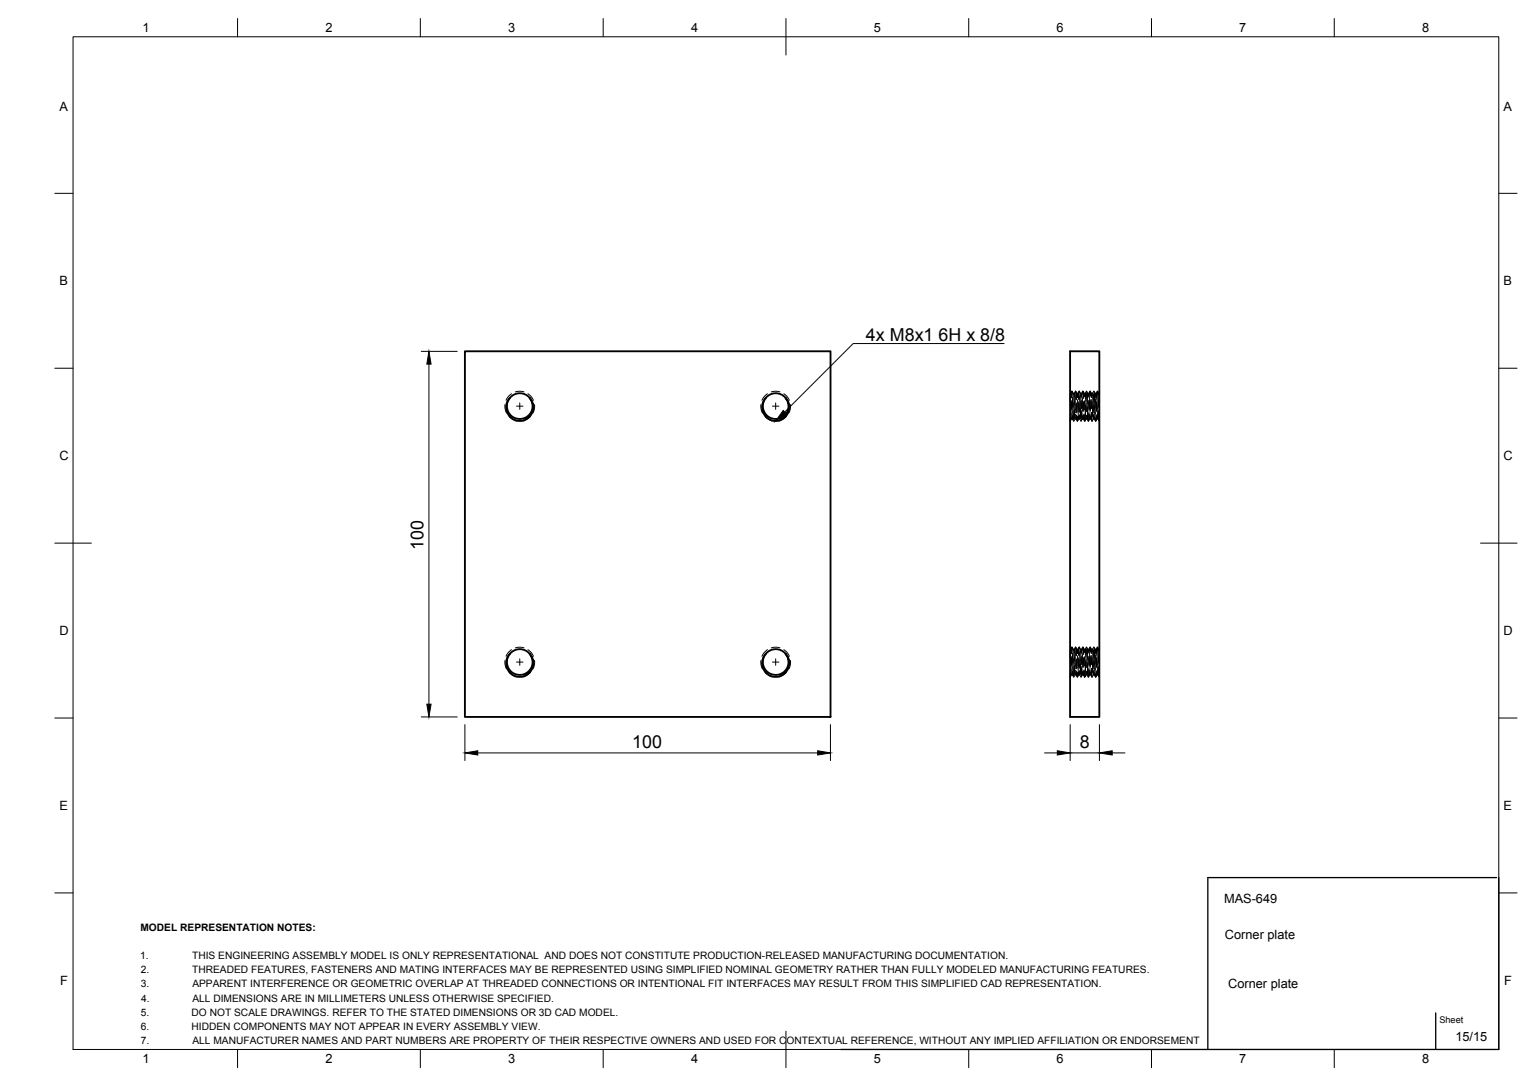
ISO-10303-21;
HEADER;
/* Generated by software containing ST-Developer
 * from STEP Tools, Inc. (www.steptools.com) 
 */

FILE_DESCRIPTION(
/* description */ ('Independent equipment support assembly with bolted 600 x 500 mm welde
d perimeter frame, four adjustable legs and swivel feet. Nominal overa
ll height 518 mm. No load rating assigned.'),
/* implementation_level */ '2;1');

FILE_NAME(
/* name */ 'Corner plate.step',
/* time_stamp */ '2026-11-07T17:30:39-08:00',
/* author */ (''),
/* organization */ (''),
/* preprocessor_version */ 'ST-DEVELOPER v20.2',
/* originating_system */ 'Autodesk Translation Framework v15.17.0.0',
/* authorisation */ '');

FILE_SCHEMA (('AUTOMOTIVE_DESIGN { 1 0 10303 214 3 1 1 }'));
ENDSEC;

DATA;
#10=MECHANICAL_DESIGN_GEOMETRIC_PRESENTATION_REPRESENTATION('',(#2210),#63755);
#257=B_SPLINE_SURFACE_WITH_KNOTS('',3,3,((#20700,#20701,#20702,#20703,#20704,
#20705,#20706,#20707,#20708,#20709,#20710,#20711,#20712,#20713,#20714,#20715,
#20716,#20717,#20718,#20719,#20720,#20721,#20722,#20723,#20724,#20725,#20726,
#20727,#20728,#20729,#20730,#20731,#20732,#20733,#20734,#20735,#20736,#20737,
#20738,#20739,#20740,#20741,#20742,#20743,#20744,#20745,#20746,#20747,#20748,
#20749,#20750,#20751,#20752,#20753,#20754,#20755),(#20756,#20757,#20758,
#20759,#20760,#20761,#20762,#20763,#20764,#20765,#20766,#20767,#20768,#20769,
#20770,#20771,#20772,#20773,#20774,#20775,#20776,#20777,#20778,#20779,#20780,
#20781,#20782,#20783,#20784,#20785,#20786,#20787,#20788,#20789,#20790,#20791,
#20792,#20793,#20794,#20795,#20796,#20797,#20798,#20799,#20800,#20801,#20802,
#20803,#20804,#20805,#20806,#20807,#20808,#20809,#20810,#20811),(#20812,
#20813,#20814,#20815,#20816,#20817,#20818,#20819,#20820,#20821,#20822,#20823,
#20824,#20825,#20826,#20827,#20828,#20829,#20830,#20831,#20832,#20833,#20834,
#20835,#20836,#20837,#20838,#20839,#20840,#20841,#20842,#20843,#20844,#20845,
#20846,#20847,#20848,#20849,#20850,#20851,#20852,#20853,#20854,#20855,#20856,
#20857,#20858,#20859,#20860,#20861,#20862,#20863,#20864,#20865,#20866,#20867),
(#20868,#20869,#20870,#20871,#20872,#20873,#20874,#20875,#20876,#20877,
#20878,#20879,#20880,#20881,#20882,#20883,#20884,#20885,#20886,#20887,#20888,
#20889,#20890,#20891,#20892,#20893,#20894,#20895,#20896,#20897,#20898,#20899,
#20900,#20901,#20902,#20903,#20904,#20905,#20906,#20907,#20908,#20909,#20910,
#20911,#20912,#20913,#20914,#20915,#20916,#20917,#20918,#20919,#20920,#20921,
#20922,#20923)),.UNSPECIFIED.,.F.,.F.,.F.,(4,4),(4,1,1,1,1,1,1,1,1,1,1,
1,1,1,1,1,1,1,1,1,1,1,1,1,1,1,1,1,1,1,1,1,1,1,1,1,1,1,1,1,1,1,1,1,1,1,1,
1,1,1,1,1,1,4),(0.,0.0642013499338865),(11.8589888623078,12.8454497557128,
13.8319106491178,14.8183715425228,15.8048324359278,16.7912933293328,17.7777542227378,
18.7642151161428,19.7506760095478,20.7371369029528,21.7235977963578,22.7100586897628,
23.6965195831678,24.6829804765728,25.6694413699778,26.6559022633828,27.6423631567878,
28.6288240501928,29.6152849435978,30.6017458370028,31.5882067304078,32.5746676238129,
33.5611285172179,34.5475894106229,35.5340503040279,36.5205111974329,37.5069720908379,
38.4934329842429,39.4798938776479,40.4663547710529,41.4528156644579,42.4392765578629,
43.4257374512679,44.4121983446729,45.3986592380779,46.3851201314829,47.3715810248879,
48.3580419182929,49.3445028116979,50.3309637051029,51.3174245985079,52.3038854919129,
53.2903463853179,54.2768072787229,55.2632681721279,56.2497290655329,57.2361899589379,
58.2226508523429,59.2091117457479,60.1955726391529,61.1820335325579,62.1684944259629,
63.1549553193679,64.1414162127729),.UNSPECIFIED.);
#258=B_SPLINE_SURFACE_WITH_KNOTS('',3,3,((#21140,#21141,#21142,#21143,#21144,
#21145,#21146,#21147,#21148,#21149,#21150,#21151,#21152,#21153,#21154,#21155,
#21156,#21157,#21158,#21159,#21160,#21161,#21162,#21163,#21164,#21165,#21166,
#21167,#21168,#21169,#21170,#21171,#21172,#21173,#21174,#21175,#21176,#21177,
#21178,#21179,#21180,#21181,#21182,#21183,#21184,#21185,#21186,#21187,#21188,
#21189,#21190,#21191,#21192,#21193,#21194,#21195),(#21196,#21197,#21198,
#21199,#21200,#21201,#21202,#21203,#21204,#21205,#21206,#21207,#21208,#21209,
#21210,#21211,#21212,#21213,#21214,#21215,#21216,#21217,#21218,#21219,#21220,
#21221,#21222,#21223,#21224,#21225,#21226,#21227,#21228,#21229,#21230,#21231,
#21232,#21233,#21234,#21235,#21236,#21237,#21238,#21239,#21240,#21241,#21242,
#21243,#21244,#21245,#21246,#21247,#21248,#21249,#21250,#21251),(#21252,
#21253,#21254,#21255,#21256,#21257,#21258,#21259,#21260,#21261,#21262,#21263,
#21264,#21265,#21266,#21267,#21268,#21269,#21270,#21271,#21272,#21273,#21274,
#21275,#21276,#21277,#21278,#21279,#21280,#21281,#21282,#21283,#21284,#21285,
#21286,#21287,#21288,#21289,#21290,#21291,#21292,#21293,#21294,#21295,#21296,
#21297,#21298,#21299,#21300,#21301,#21302,#21303,#21304,#21305,#21306,#21307),
(#21308,#21309,#21310,#21311,#21312,#21313,#21314,#21315,#21316,#21317,
#21318,#21319,#21320,#21321,#21322,#21323,#21324,#21325,#21326,#21327,#21328,
#21329,#21330,#21331,#21332,#21333,#21334,#21335,#21336,#21337,#21338,#21339,
#21340,#21341,#21342,#21343,#21344,#21345,#21346,#21347,#21348,#21349,#21350,
#21351,#21352,#21353,#21354,#21355,#21356,#21357,#21358,#21359,#21360,#21361,
#21362,#21363)),.UNSPECIFIED.,.F.,.F.,.F.,(4,4),(4,1,1,1,1,1,1,1,1,1,1,
1,1,1,1,1,1,1,1,1,1,1,1,1,1,1,1,1,1,1,1,1,1,1,1,1,1,1,1,1,1,1,1,1,1,1,1,
1,1,1,1,1,1,4),(0.,0.0642013499338865),(14.3984001269718,15.3848610203768,
16.3713219137818,17.3577828071868,18.3442437005918,19.3307045939968,20.3171654874019,
21.3036263808069,22.2900872742119,23.2765481676169,24.2630090610219,25.2494699544269,
26.2359308478319,27.2223917412369,28.2088526346419,29.1953135280469,30.1817744214519,
31.1682353148569,32.1546962082619,33.1411571016669,34.1276179950719,35.1140788884769,
36.1005397818819,37.0870006752869,38.0734615686919,39.0599224620969,40.0463833555019,
41.0328442489069,42.0193051423119,43.0057660357169,43.9922269291219,44.9786878225269,
45.9651487159319,46.9516096093369,47.9380705027419,48.9245313961469,49.9109922895519,
50.8974531829569,51.8839140763619,52.8703749697669,53.856835863172,54.843296756577,
55.829757649982,56.816218543387,57.802679436792,58.789140330197,59.775601223602,
60.762062117007,61.748523010412,62.734983903817,63.721444797222,64.707905690627,
65.694366584032,66.680827477437),.UNSPECIFIED.);
#259=B_SPLINE_SURFACE_WITH_KNOTS('',3,3,((#22184,#22185,#22186,#22187,#22188,
#22189,#22190,#22191,#22192,#22193,#22194,#22195,#22196,#22197,#22198,#22199,
#22200,#22201,#22202,#22203,#22204,#22205,#22206,#22207,#22208,#22209,#22210,
#22211,#22212,#22213,#22214,#22215,#22216,#22217,#22218,#22219,#22220,#22221,
#22222,#22223,#22224,#22225,#22226,#22227,#22228,#22229,#22230,#22231,#22232,
#22233,#22234,#22235,#22236,#22237,#22238,#22239),(#22240,#22241,#22242,
#22243,#22244,#22245,#22246,#22247,#22248,#22249,#22250,#22251,#22252,#22253,
#22254,#22255,#22256,#22257,#22258,#22259,#22260,#22261,#22262,#22263,#22264,
#22265,#22266,#22267,#22268,#22269,#22270,#22271,#22272,#22273,#22274,#22275,
#22276,#22277,#22278,#22279,#22280,#22281,#22282,#22283,#22284,#22285,#22286,
#22287,#22288,#22289,#22290,#22291,#22292,#22293,#22294,#22295),(#22296,
#22297,#22298,#22299,#22300,#22301,#22302,#22303,#22304,#22305,#22306,#22307,
#22308,#22309,#22310,#22311,#22312,#22313,#22314,#22315,#22316,#22317,#22318,
#22319,#22320,#22321,#22322,#22323,#22324,#22325,#22326,#22327,#22328,#22329,
#22330,#22331,#22332,#22333,#22334,#22335,#22336,#22337,#22338,#22339,#22340,
#22341,#22342,#22343,#22344,#22345,#22346,#22347,#22348,#22349,#22350,#22351),
(#22352,#22353,#22354,#22355,#22356,#22357,#22358,#22359,#22360,#22361,
#22362,#22363,#22364,#22365,#22366,#22367,#22368,#22369,#22370,#22371,#22372,
#22373,#22374,#22375,#22376,#22377,#22378,#22379,#22380,#22381,#22382,#22383,
#22384,#22385,#22386,#22387,#22388,#22389,#22390,#22391,#22392,#22393,#22394,
#22395,#22396,#22397,#22398,#22399,#22400,#22401,#22402,#22403,#22404,#22405,
#22406,#22407)),.UNSPECIFIED.,.F.,.F.,.F.,(4,4),(4,1,1,1,1,1,1,1,1,1,1,
1,1,1,1,1,1,1,1,1,1,1,1,1,1,1,1,1,1,1,1,1,1,1,1,1,1,1,1,1,1,1,1,1,1,1,1,
1,1,1,1,1,1,4),(0.,0.0642013499338865),(11.8589888623078,12.8454497557128,
13.8319106491178,14.8183715425228,15.8048324359278,16.7912933293328,17.7777542227378,
18.7642151161428,19.7506760095478,20.7371369029528,21.7235977963578,22.7100586897628,
23.6965195831678,24.6829804765728,25.6694413699778,26.6559022633828,27.6423631567879,
28.6288240501929,29.6152849435979,30.6017458370029,31.5882067304079,32.5746676238129,
33.5611285172179,34.5475894106229,35.5340503040279,36.5205111974329,37.5069720908379,
38.4934329842429,39.4798938776479,40.4663547710529,41.4528156644579,42.4392765578629,
43.4257374512679,44.4121983446729,45.3986592380779,46.3851201314829,47.3715810248879,
48.3580419182929,49.3445028116979,50.3309637051029,51.3174245985079,52.3038854919129,
53.2903463853179,54.2768072787229,55.2632681721279,56.2497290655329,57.2361899589379,
58.2226508523429,59.2091117457479,60.1955726391529,61.1820335325579,62.1684944259629,
63.154955319368,64.141416212773),.UNSPECIFIED.);
#260=B_SPLINE_SURFACE_WITH_KNOTS('',3,3,((#22530,#22531,#22532,#22533,#22534,
#22535,#22536,#22537,#22538,#22539,#22540,#22541,#22542,#22543,#22544,#22545,
#22546,#22547,#22548,#22549,#22550,#22551,#22552,#22553,#22554,#22555,#22556,
#22557,#22558,#22559,#22560,#22561,#22562,#22563,#22564,#22565,#22566,#22567,
#22568,#22569,#22570,#22571,#22572,#22573,#22574,#22575,#22576,#22577,#22578,
#22579,#22580,#22581,#22582,#22583,#22584,#22585),(#22586,#22587,#22588,
#22589,#22590,#22591,#22592,#22593,#22594,#22595,#22596,#22597,#22598,#22599,
#22600,#22601,#22602,#22603,#22604,#22605,#22606,#22607,#22608,#22609,#22610,
#22611,#22612,#22613,#22614,#22615,#22616,#22617,#22618,#22619,#22620,#22621,
#22622,#22623,#22624,#22625,#22626,#22627,#22628,#22629,#22630,#22631,#22632,
#22633,#22634,#22635,#22636,#22637,#22638,#22639,#22640,#22641),(#22642,
#22643,#22644,#22645,#22646,#22647,#22648,#22649,#22650,#22651,#22652,#22653,
#22654,#22655,#22656,#22657,#22658,#22659,#22660,#22661,#22662,#22663,#22664,
#22665,#22666,#22667,#22668,#22669,#22670,#22671,#22672,#22673,#22674,#22675,
#22676,#22677,#22678,#22679,#22680,#22681,#22682,#22683,#22684,#22685,#22686,
#22687,#22688,#22689,#22690,#22691,#22692,#22693,#22694,#22695,#22696,#22697),
(#22698,#22699,#22700,#22701,#22702,#22703,#22704,#22705,#22706,#22707,
#22708,#22709,#22710,#22711,#22712,#22713,#22714,#22715,#22716,#22717,#22718,
#22719,#22720,#22721,#22722,#22723,#22724,#22725,#22726,#22727,#22728,#22729,
#22730,#22731,#22732,#22733,#22734,#22735,#22736,#22737,#22738,#22739,#22740,
#22741,#22742,#22743,#22744,#22745,#22746,#22747,#22748,#22749,#22750,#22751,
#22752,#22753)),.UNSPECIFIED.,.F.,.F.,.F.,(4,4),(4,1,1,1,1,1,1,1,1,1,1,
1,1,1,1,1,1,1,1,1,1,1,1,1,1,1,1,1,1,1,1,1,1,1,1,1,1,1,1,1,1,1,1,1,1,1,1,
1,1,1,1,1,1,4),(0.,0.0642013499338865),(14.3984001269718,15.3848610203768,
16.3713219137818,17.3577828071869,18.3442437005919,19.3307045939969,20.3171654874019,
21.3036263808069,22.2900872742119,23.2765481676169,24.2630090610219,25.2494699544269,
26.2359308478319,27.2223917412369,28.2088526346419,29.1953135280469,30.1817744214519,
31.1682353148569,32.1546962082619,33.1411571016669,34.1276179950719,35.1140788884769,
36.1005397818819,37.0870006752869,38.0734615686919,39.0599224620969,40.0463833555019,
41.0328442489069,42.0193051423119,43.0057660357169,43.9922269291219,44.9786878225269,
45.9651487159319,46.9516096093369,47.9380705027419,48.9245313961469,49.9109922895519,
50.8974531829569,51.8839140763619,52.8703749697669,53.856835863172,54.843296756577,
55.829757649982,56.816218543387,57.802679436792,58.789140330197,59.775601223602,
60.762062117007,61.748523010412,62.734983903817,63.721444797222,64.707905690627,
65.694366584032,66.680827477437),.UNSPECIFIED.);
#261=B_SPLINE_SURFACE_WITH_KNOTS('',3,3,((#22895,#22896,#22897,#22898,#22899,
#22900,#22901,#22902,#22903,#22904,#22905,#22906,#22907,#22908,#22909,#22910,
#22911,#22912,#22913,#22914,#22915,#22916,#22917,#22918,#22919,#22920,#22921,
#22922,#22923,#22924,#22925,#22926,#22927,#22928,#22929,#22930,#22931,#22932,
#22933,#22934,#22935,#22936,#22937,#22938,#22939,#22940,#22941,#22942,#22943,
#22944,#22945,#22946,#22947,#22948,#22949,#22950),(#22951,#22952,#22953,
#22954,#22955,#22956,#22957,#22958,#22959,#22960,#22961,#22962,#22963,#22964,
#22965,#22966,#22967,#22968,#22969,#22970,#22971,#22972,#22973,#22974,#22975,
#22976,#22977,#22978,#22979,#22980,#22981,#22982,#22983,#22984,#22985,#22986,
#22987,#22988,#22989,#22990,#22991,#22992,#22993,#22994,#22995,#22996,#22997,
#22998,#22999,#23000,#23001,#23002,#23003,#23004,#23005,#23006),(#23007,
#23008,#23009,#23010,#23011,#23012,#23013,#23014,#23015,#23016,#23017,#23018,
#23019,#23020,#23021,#23022,#23023,#23024,#23025,#23026,#23027,#23028,#23029,
#23030,#23031,#23032,#23033,#23034,#23035,#23036,#23037,#23038,#23039,#23040,
#23041,#23042,#23043,#23044,#23045,#23046,#23047,#23048,#23049,#23050,#23051,
#23052,#23053,#23054,#23055,#23056,#23057,#23058,#23059,#23060,#23061,#23062),
(#23063,#23064,#23065,#23066,#23067,#23068,#23069,#23070,#23071,#23072,
#23073,#23074,#23075,#23076,#23077,#23078,#23079,#23080,#23081,#23082,#23083,
#23084,#23085,#23086,#23087,#23088,#23089,#23090,#23091,#23092,#23093,#23094,
#23095,#23096,#23097,#23098,#23099,#23100,#23101,#23102,#23103,#23104,#23105,
#23106,#23107,#23108,#23109,#23110,#23111,#23112,#23113,#23114,#23115,#23116,
#23117,#23118)),.UNSPECIFIED.,.F.,.F.,.F.,(4,4),(4,1,1,1,1,1,1,1,1,1,1,
1,1,1,1,1,1,1,1,1,1,1,1,1,1,1,1,1,1,1,1,1,1,1,1,1,1,1,1,1,1,1,1,1,1,1,1,
1,1,1,1,1,1,4),(0.,0.0642013499338865),(11.8589888623078,12.8454497557128,
13.8319106491178,14.8183715425228,15.8048324359278,16.7912933293328,17.7777542227378,
18.7642151161428,19.7506760095478,20.7371369029528,21.7235977963578,22.7100586897628,
23.6965195831678,24.6829804765728,25.6694413699778,26.6559022633828,27.6423631567878,
28.6288240501928,29.6152849435978,30.6017458370028,31.5882067304078,32.5746676238129,
33.5611285172179,34.5475894106229,35.5340503040279,36.5205111974329,37.5069720908379,
38.4934329842429,39.4798938776479,40.4663547710529,41.4528156644579,42.4392765578629,
43.4257374512679,44.4121983446729,45.3986592380779,46.3851201314829,47.3715810248879,
48.3580419182929,49.3445028116979,50.3309637051029,51.3174245985079,52.3038854919129,
53.2903463853179,54.2768072787229,55.2632681721279,56.2497290655329,57.2361899589379,
58.2226508523429,59.2091117457479,60.1955726391529,61.1820335325579,62.1684944259629,
63.1549553193679,64.1414162127729),.UNSPECIFIED.);
#262=B_SPLINE_SURFACE_WITH_KNOTS('',3,3,((#23241,#23242,#23243,#23244,#23245,
#23246,#23247,#23248,#23249,#23250,#23251,#23252,#23253,#23254,#23255,#23256,
#23257,#23258,#23259,#23260,#23261,#23262,#23263,#23264,#23265,#23266,#23267,
#23268,#23269,#23270,#23271,#23272,#23273,#23274,#23275,#23276,#23277,#23278,
#23279,#23280,#23281,#23282,#23283,#23284,#23285,#23286,#23287,#23288,#23289,
#23290,#23291,#23292,#23293,#23294,#23295,#23296),(#23297,#23298,#23299,
#23300,#23301,#23302,#23303,#23304,#23305,#23306,#23307,#23308,#23309,#23310,
#23311,#23312,#23313,#23314,#23315,#23316,#23317,#23318,#23319,#23320,#23321,
#23322,#23323,#23324,#23325,#23326,#23327,#23328,#23329,#23330,#23331,#23332,
#23333,#23334,#23335,#23336,#23337,#23338,#23339,#23340,#23341,#23342,#23343,
#23344,#23345,#23346,#23347,#23348,#23349,#23350,#23351,#23352),(#23353,
#23354,#23355,#23356,#23357,#23358,#23359,#23360,#23361,#23362,#23363,#23364,
#23365,#23366,#23367,#23368,#23369,#23370,#23371,#23372,#23373,#23374,#23375,
#23376,#23377,#23378,#23379,#23380,#23381,#23382,#23383,#23384,#23385,#23386,
#23387,#23388,#23389,#23390,#23391,#23392,#23393,#23394,#23395,#23396,#23397,
#23398,#23399,#23400,#23401,#23402,#23403,#23404,#23405,#23406,#23407,#23408),
(#23409,#23410,#23411,#23412,#23413,#23414,#23415,#23416,#23417,#23418,
#23419,#23420,#23421,#23422,#23423,#23424,#23425,#23426,#23427,#23428,#23429,
#23430,#23431,#23432,#23433,#23434,#23435,#23436,#23437,#23438,#23439,#23440,
#23441,#23442,#23443,#23444,#23445,#23446,#23447,#23448,#23449,#23450,#23451,
#23452,#23453,#23454,#23455,#23456,#23457,#23458,#23459,#23460,#23461,#23462,
#23463,#23464)),.UNSPECIFIED.,.F.,.F.,.F.,(4,4),(4,1,1,1,1,1,1,1,1,1,1,
1,1,1,1,1,1,1,1,1,1,1,1,1,1,1,1,1,1,1,1,1,1,1,1,1,1,1,1,1,1,1,1,1,1,1,1,
1,1,1,1,1,1,4),(0.,0.0642013499338865),(14.3984001269718,15.3848610203768,
16.3713219137818,17.3577828071868,18.3442437005918,19.3307045939968,20.3171654874019,
21.3036263808069,22.2900872742119,23.2765481676169,24.2630090610219,25.2494699544269,
26.2359308478319,27.2223917412369,28.2088526346419,29.1953135280469,30.1817744214519,
31.1682353148569,32.1546962082619,33.1411571016669,34.1276179950719,35.1140788884769,
36.1005397818819,37.0870006752869,38.0734615686919,39.0599224620969,40.0463833555019,
41.0328442489069,42.0193051423119,43.0057660357169,43.9922269291219,44.9786878225269,
45.9651487159319,46.9516096093369,47.9380705027419,48.9245313961469,49.9109922895519,
50.8974531829569,51.8839140763619,52.8703749697669,53.856835863172,54.843296756577,
55.829757649982,56.816218543387,57.802679436792,58.789140330197,59.775601223602,
60.762062117007,61.748523010412,62.734983903817,63.721444797222,64.707905690627,
65.694366584032,66.680827477437),.UNSPECIFIED.);
#263=B_SPLINE_SURFACE_WITH_KNOTS('',3,3,((#23606,#23607,#23608,#23609,#23610,
#23611,#23612,#23613,#23614,#23615,#23616,#23617,#23618,#23619,#23620,#23621,
#23622,#23623,#23624,#23625,#23626,#23627,#23628,#23629,#23630,#23631,#23632,
#23633,#23634,#23635,#23636,#23637,#23638,#23639,#23640,#23641,#23642,#23643,
#23644,#23645,#23646,#23647,#23648,#23649,#23650,#23651,#23652,#23653,#23654,
#23655,#23656,#23657,#23658,#23659,#23660,#23661),(#23662,#23663,#23664,
#23665,#23666,#23667,#23668,#23669,#23670,#23671,#23672,#23673,#23674,#23675,
#23676,#23677,#23678,#23679,#23680,#23681,#23682,#23683,#23684,#23685,#23686,
#23687,#23688,#23689,#23690,#23691,#23692,#23693,#23694,#23695,#23696,#23697,
#23698,#23699,#23700,#23701,#23702,#23703,#23704,#23705,#23706,#23707,#23708,
#23709,#23710,#23711,#23712,#23713,#23714,#23715,#23716,#23717),(#23718,
#23719,#23720,#23721,#23722,#23723,#23724,#23725,#23726,#23727,#23728,#23729,
#23730,#23731,#23732,#23733,#23734,#23735,#23736,#23737,#23738,#23739,#23740,
#23741,#23742,#23743,#23744,#23745,#23746,#23747,#23748,#23749,#23750,#23751,
#23752,#23753,#23754,#23755,#23756,#23757,#23758,#23759,#23760,#23761,#23762,
#23763,#23764,#23765,#23766,#23767,#23768,#23769,#23770,#23771,#23772,#23773),
(#23774,#23775,#23776,#23777,#23778,#23779,#23780,#23781,#23782,#23783,
#23784,#23785,#23786,#23787,#23788,#23789,#23790,#23791,#23792,#23793,#23794,
#23795,#23796,#23797,#23798,#23799,#23800,#23801,#23802,#23803,#23804,#23805,
#23806,#23807,#23808,#23809,#23810,#23811,#23812,#23813,#23814,#23815,#23816,
#23817,#23818,#23819,#23820,#23821,#23822,#23823,#23824,#23825,#23826,#23827,
#23828,#23829)),.UNSPECIFIED.,.F.,.F.,.F.,(4,4),(4,1,1,1,1,1,1,1,1,1,1,
1,1,1,1,1,1,1,1,1,1,1,1,1,1,1,1,1,1,1,1,1,1,1,1,1,1,1,1,1,1,1,1,1,1,1,1,
1,1,1,1,1,1,4),(0.,0.0642013499338865),(11.8589888623078,12.8454497557128,
13.8319106491178,14.8183715425228,15.8048324359278,16.7912933293328,17.7777542227378,
18.7642151161428,19.7506760095478,20.7371369029528,21.7235977963578,22.7100586897628,
23.6965195831678,24.6829804765728,25.6694413699778,26.6559022633828,27.6423631567879,
28.6288240501929,29.6152849435979,30.6017458370029,31.5882067304079,32.5746676238129,
33.5611285172179,34.5475894106229,35.5340503040279,36.5205111974329,37.5069720908379,
38.4934329842429,39.4798938776479,40.4663547710529,41.4528156644579,42.4392765578629,
43.4257374512679,44.4121983446729,45.3986592380779,46.3851201314829,47.3715810248879,
48.3580419182929,49.3445028116979,50.3309637051029,51.3174245985079,52.3038854919129,
53.2903463853179,54.2768072787229,55.2632681721279,56.2497290655329,57.2361899589379,
58.2226508523429,59.2091117457479,60.1955726391529,61.1820335325579,62.1684944259629,
63.154955319368,64.141416212773),.UNSPECIFIED.);
#264=B_SPLINE_SURFACE_WITH_KNOTS('',3,3,((#23952,#23953,#23954,#23955,#23956,
#23957,#23958,#23959,#23960,#23961,#23962,#23963,#23964,#23965,#23966,#23967,
#23968,#23969,#23970,#23971,#23972,#23973,#23974,#23975,#23976,#23977,#23978,
#23979,#23980,#23981,#23982,#23983,#23984,#23985,#23986,#23987,#23988,#23989,
#23990,#23991,#23992,#23993,#23994,#23995,#23996,#23997,#23998,#23999,#24000,
#24001,#24002,#24003,#24004,#24005,#24006,#24007),(#24008,#24009,#24010,
#24011,#24012,#24013,#24014,#24015,#24016,#24017,#24018,#24019,#24020,#24021,
#24022,#24023,#24024,#24025,#24026,#24027,#24028,#24029,#24030,#24031,#24032,
#24033,#24034,#24035,#24036,#24037,#24038,#24039,#24040,#24041,#24042,#24043,
#24044,#24045,#24046,#24047,#24048,#24049,#24050,#24051,#24052,#24053,#24054,
#24055,#24056,#24057,#24058,#24059,#24060,#24061,#24062,#24063),(#24064,
#24065,#24066,#24067,#24068,#24069,#24070,#24071,#24072,#24073,#24074,#24075,
#24076,#24077,#24078,#24079,#24080,#24081,#24082,#24083,#24084,#24085,#24086,
#24087,#24088,#24089,#24090,#24091,#24092,#24093,#24094,#24095,#24096,#24097,
#24098,#24099,#24100,#24101,#24102,#24103,#24104,#24105,#24106,#24107,#24108,
#24109,#24110,#24111,#24112,#24113,#24114,#24115,#24116,#24117,#24118,#24119),
(#24120,#24121,#24122,#24123,#24124,#24125,#24126,#24127,#24128,#24129,
#24130,#24131,#24132,#24133,#24134,#24135,#24136,#24137,#24138,#24139,#24140,
#24141,#24142,#24143,#24144,#24145,#24146,#24147,#24148,#24149,#24150,#24151,
#24152,#24153,#24154,#24155,#24156,#24157,#24158,#24159,#24160,#24161,#24162,
#24163,#24164,#24165,#24166,#24167,#24168,#24169,#24170,#24171,#24172,#24173,
#24174,#24175)),.UNSPECIFIED.,.F.,.F.,.F.,(4,4),(4,1,1,1,1,1,1,1,1,1,1,
1,1,1,1,1,1,1,1,1,1,1,1,1,1,1,1,1,1,1,1,1,1,1,1,1,1,1,1,1,1,1,1,1,1,1,1,
1,1,1,1,1,1,4),(0.,0.0642013499338865),(14.3984001269718,15.3848610203768,
16.3713219137818,17.3577828071869,18.3442437005919,19.3307045939969,20.3171654874019,
21.3036263808069,22.2900872742119,23.2765481676169,24.2630090610219,25.2494699544269,
26.2359308478319,27.2223917412369,28.2088526346419,29.1953135280469,30.1817744214519,
31.1682353148569,32.1546962082619,33.1411571016669,34.1276179950719,35.1140788884769,
36.1005397818819,37.0870006752869,38.0734615686919,39.0599224620969,40.0463833555019,
41.0328442489069,42.0193051423119,43.0057660357169,43.9922269291219,44.9786878225269,
45.9651487159319,46.9516096093369,47.9380705027419,48.9245313961469,49.9109922895519,
50.8974531829569,51.8839140763619,52.8703749697669,53.856835863172,54.843296756577,
55.829757649982,56.816218543387,57.802679436792,58.789140330197,59.775601223602,
60.762062117007,61.748523010412,62.734983903817,63.721444797222,64.707905690627,
65.694366584032,66.680827477437),.UNSPECIFIED.);
#285=CIRCLE('',#14528,3.5175);
#286=CIRCLE('',#14536,3.5175);
#287=CIRCLE('',#14538,3.5175);
#288=CIRCLE('',#14546,3.5175);
#289=CIRCLE('',#14548,3.5175);
#290=CIRCLE('',#14556,3.5175);
#291=CIRCLE('',#14558,3.5175);
#292=CIRCLE('',#14566,3.5175);
#293=CIRCLE('',#14568,4.0735);
#294=CIRCLE('',#14576,4.07350000000001);
#295=CIRCLE('',#14578,4.0735);
#296=CIRCLE('',#14586,4.07350000000001);
#297=CIRCLE('',#14588,4.0735);
#298=CIRCLE('',#14596,4.0735);
#299=CIRCLE('',#14598,4.0735);
#300=CIRCLE('',#14606,4.0735);
#487=B_SPLINE_CURVE_WITH_KNOTS('',3,(#18487,#18488,#18489,#18490),
 .UNSPECIFIED.,.F.,.F.,(4,4),(51.5750455984138,52.2824273504652),
 .UNSPECIFIED.);
#488=B_SPLINE_CURVE_WITH_KNOTS('',3,(#18493,#18494,#18495,#18496,#18497,
#18498,#18499,#18500,#18501,#18502),.UNSPECIFIED.,.F.,.F.,(4,3,3,4),(-50.2654824574367,
-49.3230446702501,-48.3365837768451,-47.8312715558983),.UNSPECIFIED.);
#489=B_SPLINE_CURVE_WITH_KNOTS('',3,(#18507,#18508,#18509,#18510,#18511,
#18512,#18513,#18514,#18515,#18516,#18517,#18518,#18519,#18520,#18521,#18522,
#18523,#18524,#18525,#18526,#18527,#18528,#18529,#18530,#18531),
 .UNSPECIFIED.,.F.,.F.,(4,3,3,3,3,3,3,3,4),(45.2918602912342,45.3772010966301,
46.3636619900351,47.3501228834401,48.3365837768452,49.3230446702501,50.3095055636552,
51.2959664570602,51.5750455984138),.UNSPECIFIED.);
#490=B_SPLINE_CURVE_WITH_KNOTS('',3,(#18532,#18533,#18534,#18535,#18536,
#18537,#18538,#18539,#18540,#18541,#18542,#18543,#18544,#18545,#18546,#18547,
#18548,#18549,#18550,#18551,#18552,#18553),.UNSPECIFIED.,.F.,.F.,(4,3,3,
3,3,3,3,4),(-47.8312715558983,-47.3501228834401,-46.3636619900351,-45.3772010966301,
-44.3907402032251,-43.4042793098201,-42.4178184164151,-41.5480862487187),
 .UNSPECIFIED.);
#491=B_SPLINE_CURVE_WITH_KNOTS('',3,(#18558,#18559,#18560,#18561,#18562,
#18563,#18564,#18565,#18566,#18567,#18568,#18569,#18570,#18571,#18572,#18573,
#18574,#18575,#18576,#18577,#18578,#18579),.UNSPECIFIED.,.F.,.F.,(4,3,3,
3,3,3,3,4),(39.0086749840546,39.4584357362001,40.4448966296051,41.4313575230101,
42.4178184164151,43.4042793098201,44.3907402032251,45.2918602912342),
 .UNSPECIFIED.);
#492=B_SPLINE_CURVE_WITH_KNOTS('',3,(#18580,#18581,#18582,#18583,#18584,
#18585,#18586,#18587,#18588,#18589,#18590,#18591,#18592,#18593,#18594,#18595,
#18596,#18597,#18598,#18599,#18600,#18601,#18602,#18603,#18604),
 .UNSPECIFIED.,.F.,.F.,(4,3,3,3,3,3,3,3,4),(-41.5480862487187,-41.4313575230101,
-40.4448966296051,-39.4584357362001,-38.4719748427951,-37.4855139493901,
-36.4990530559851,-35.5125921625801,-35.2649009415391),.UNSPECIFIED.);
#493=B_SPLINE_CURVE_WITH_KNOTS('',3,(#18609,#18610,#18611,#18612,#18613,
#18614,#18615,#18616,#18617,#18618,#18619,#18620,#18621,#18622,#18623,#18624,
#18625,#18626,#18627,#18628,#18629,#18630),.UNSPECIFIED.,.F.,.F.,(4,3,3,
3,3,3,3,4),(32.725489676875,33.5396703757701,34.5261312691751,35.5125921625801,
36.4990530559851,37.4855139493901,38.4719748427951,39.0086749840546),
 .UNSPECIFIED.);
#494=B_SPLINE_CURVE_WITH_KNOTS('',3,(#18631,#18632,#18633,#18634,#18635,
#18636,#18637,#18638,#18639,#18640,#18641,#18642,#18643,#18644,#18645,#18646,
#18647,#18648,#18649,#18650,#18651,#18652),.UNSPECIFIED.,.F.,.F.,(4,3,3,
3,3,3,3,4),(-35.2649009415391,-34.5261312691751,-33.5396703757701,-32.5532094823651,
-31.5667485889601,-30.5802876955551,-29.5938268021501,-28.9817156343595),
 .UNSPECIFIED.);
#495=B_SPLINE_CURVE_WITH_KNOTS('',3,(#18657,#18658,#18659,#18660,#18661,
#18662,#18663,#18664,#18665,#18666,#18667,#18668,#18669,#18670,#18671,#18672,
#18673,#18674,#18675,#18676,#18677,#18678,#18679,#18680,#18681),
 .UNSPECIFIED.,.F.,.F.,(4,3,3,3,3,3,3,3,4),(26.4423043696954,26.6344441219351,
27.6209050153401,28.6073659087451,29.5938268021501,30.5802876955551,31.5667485889601,
32.5532094823651,32.725489676875),.UNSPECIFIED.);
#496=B_SPLINE_CURVE_WITH_KNOTS('',3,(#18682,#18683,#18684,#18685,#18686,
#18687,#18688,#18689,#18690,#18691,#18692,#18693,#18694,#18695,#18696,#18697,
#18698,#18699,#18700,#18701,#18702,#18703),.UNSPECIFIED.,.F.,.F.,(4,3,3,
3,3,3,3,4),(-28.9817156343595,-28.6073659087451,-27.6209050153401,-26.6344441219351,
-25.6479832285301,-24.6615223351251,-23.6750614417201,-22.6985303271799),
 .UNSPECIFIED.);
#497=B_SPLINE_CURVE_WITH_KNOTS('',3,(#18708,#18709,#18710,#18711,#18712,
#18713,#18714,#18715,#18716,#18717,#18718,#18719,#18720,#18721,#18722,#18723,
#18724,#18725,#18726,#18727,#18728,#18729),.UNSPECIFIED.,.F.,.F.,(4,3,3,
3,3,3,3,4),(20.1591190625159,20.7156787615051,21.7021396549101,22.6886005483151,
23.6750614417201,24.6615223351251,25.6479832285301,26.4423043696954),
 .UNSPECIFIED.);
#498=B_SPLINE_CURVE_WITH_KNOTS('',3,(#18730,#18731,#18732,#18733,#18734,
#18735,#18736,#18737,#18738,#18739,#18740,#18741,#18742,#18743,#18744,#18745,
#18746,#18747,#18748,#18749,#18750,#18751,#18752,#18753,#18754),
 .UNSPECIFIED.,.F.,.F.,(4,3,3,3,3,3,3,3,4),(-22.6985303271799,-22.6886005483151,
-21.7021396549101,-20.7156787615051,-19.7292178681001,-18.7427569746951,
-17.7562960812901,-16.7698351878851,-16.4153450200003),.UNSPECIFIED.);
#499=B_SPLINE_CURVE_WITH_KNOTS('',3,(#18759,#18760,#18761,#18762,#18763,
#18764,#18765,#18766,#18767,#18768,#18769,#18770,#18771,#18772,#18773,#18774,
#18775,#18776,#18777,#18778,#18779,#18780),.UNSPECIFIED.,.F.,.F.,(4,3,3,
3,3,3,3,4),(13.8759337553363,14.7969134010751,15.78337429448,16.7698351878851,
17.75629608129,18.7427569746951,19.7292178681001,20.1591190625159),
 .UNSPECIFIED.);
#500=B_SPLINE_CURVE_WITH_KNOTS('',3,(#18781,#18782,#18783,#18784,#18785,
#18786,#18787,#18788,#18789,#18790,#18791,#18792,#18793,#18794,#18795,#18796,
#18797,#18798,#18799,#18800,#18801,#18802),.UNSPECIFIED.,.F.,.F.,(4,3,3,
3,3,3,3,4),(-16.4153450200003,-15.78337429448,-14.796913401075,-13.81045250767,
-12.823991614265,-11.83753072086,-10.851069827455,-10.1321597128207),
 .UNSPECIFIED.);
#501=B_SPLINE_CURVE_WITH_KNOTS('',3,(#18808,#18809,#18810,#18811,#18812,
#18813,#18814,#18815,#18816,#18817,#18818,#18819,#18820),.UNSPECIFIED.,
 .F.,.F.,(4,3,3,3,4),(-3.84897440564115,-2.95938268021501,-1.97292178681001,
-0.986460893405001,0.),.UNSPECIFIED.);
#502=B_SPLINE_CURVE_WITH_KNOTS('',3,(#18823,#18824,#18825,#18826,#18827,
#18828,#18829,#18830,#18831,#18832,#18833,#18834,#18835,#18836,#18837,#18838,
#18839,#18840,#18841),.UNSPECIFIED.,.F.,.F.,(4,3,3,3,3,3,4),(2.01694489302848,
2.95938268021501,3.94584357362001,4.93230446702502,5.91876536043002,6.90522625383502,
7.59274844815668),.UNSPECIFIED.);
#503=B_SPLINE_CURVE_WITH_KNOTS('',3,(#18847,#18848,#18849,#18850),
 .UNSPECIFIED.,.F.,.F.,(4,4),(51.5750455984138,52.2824273504652),
 .UNSPECIFIED.);
#504=B_SPLINE_CURVE_WITH_KNOTS('',3,(#18853,#18854,#18855,#18856,#18857,
#18858,#18859,#18860,#18861,#18862),.UNSPECIFIED.,.F.,.F.,(4,3,3,4),(-50.2654824574367,
-49.3230446702501,-48.3365837768451,-47.8312715558982),.UNSPECIFIED.);
#505=B_SPLINE_CURVE_WITH_KNOTS('',3,(#18867,#18868,#18869,#18870,#18871,
#18872,#18873,#18874,#18875,#18876,#18877,#18878,#18879,#18880,#18881,#18882,
#18883,#18884,#18885,#18886,#18887,#18888,#18889,#18890,#18891),
 .UNSPECIFIED.,.F.,.F.,(4,3,3,3,3,3,3,3,4),(45.2918602912342,45.3772010966301,
46.3636619900351,47.3501228834401,48.3365837768451,49.3230446702501,50.3095055636551,
51.2959664570602,51.5750455984138),.UNSPECIFIED.);
#506=B_SPLINE_CURVE_WITH_KNOTS('',3,(#18892,#18893,#18894,#18895,#18896,
#18897,#18898,#18899,#18900,#18901,#18902,#18903,#18904,#18905,#18906,#18907,
#18908,#18909,#18910,#18911,#18912,#18913),.UNSPECIFIED.,.F.,.F.,(4,3,3,
3,3,3,3,4),(-47.8312715558982,-47.3501228834401,-46.3636619900351,-45.3772010966301,
-44.3907402032251,-43.4042793098201,-42.4178184164151,-41.5480862487187),
 .UNSPECIFIED.);
#507=B_SPLINE_CURVE_WITH_KNOTS('',3,(#18918,#18919,#18920,#18921,#18922,
#18923,#18924,#18925,#18926,#18927,#18928,#18929,#18930,#18931,#18932,#18933,
#18934,#18935,#18936,#18937,#18938,#18939),.UNSPECIFIED.,.F.,.F.,(4,3,3,
3,3,3,3,4),(39.0086749840546,39.4584357362001,40.4448966296051,41.4313575230101,
42.4178184164151,43.4042793098201,44.3907402032251,45.2918602912342),
 .UNSPECIFIED.);
#508=B_SPLINE_CURVE_WITH_KNOTS('',3,(#18940,#18941,#18942,#18943,#18944,
#18945,#18946,#18947,#18948,#18949,#18950,#18951,#18952,#18953,#18954,#18955,
#18956,#18957,#18958,#18959,#18960,#18961,#18962,#18963,#18964),
 .UNSPECIFIED.,.F.,.F.,(4,3,3,3,3,3,3,3,4),(-41.5480862487187,-41.4313575230101,
-40.4448966296051,-39.4584357362001,-38.4719748427951,-37.4855139493901,
-36.4990530559851,-35.5125921625801,-35.2649009415391),.UNSPECIFIED.);
#509=B_SPLINE_CURVE_WITH_KNOTS('',3,(#18969,#18970,#18971,#18972,#18973,
#18974,#18975,#18976,#18977,#18978,#18979,#18980,#18981,#18982,#18983,#18984,
#18985,#18986,#18987,#18988,#18989,#18990),.UNSPECIFIED.,.F.,.F.,(4,3,3,
3,3,3,3,4),(32.725489676875,33.5396703757701,34.5261312691751,35.5125921625801,
36.4990530559851,37.4855139493901,38.4719748427951,39.0086749840546),
 .UNSPECIFIED.);
#510=B_SPLINE_CURVE_WITH_KNOTS('',3,(#18991,#18992,#18993,#18994,#18995,
#18996,#18997,#18998,#18999,#19000,#19001,#19002,#19003,#19004,#19005,#19006,
#19007,#19008,#19009,#19010,#19011,#19012),.UNSPECIFIED.,.F.,.F.,(4,3,3,
3,3,3,3,4),(-35.2649009415391,-34.5261312691751,-33.5396703757701,-32.5532094823651,
-31.5667485889601,-30.5802876955551,-29.5938268021501,-28.9817156343595),
 .UNSPECIFIED.);
#511=B_SPLINE_CURVE_WITH_KNOTS('',3,(#19017,#19018,#19019,#19020,#19021,
#19022,#19023,#19024,#19025,#19026,#19027,#19028,#19029,#19030,#19031,#19032,
#19033,#19034,#19035,#19036,#19037,#19038,#19039,#19040,#19041),
 .UNSPECIFIED.,.F.,.F.,(4,3,3,3,3,3,3,3,4),(26.4423043696954,26.6344441219351,
27.6209050153401,28.6073659087451,29.5938268021501,30.5802876955551,31.5667485889601,
32.5532094823651,32.725489676875),.UNSPECIFIED.);
#512=B_SPLINE_CURVE_WITH_KNOTS('',3,(#19042,#19043,#19044,#19045,#19046,
#19047,#19048,#19049,#19050,#19051,#19052,#19053,#19054,#19055,#19056,#19057,
#19058,#19059,#19060,#19061,#19062,#19063),.UNSPECIFIED.,.F.,.F.,(4,3,3,
3,3,3,3,4),(-28.9817156343595,-28.6073659087451,-27.6209050153401,-26.6344441219351,
-25.6479832285301,-24.6615223351251,-23.6750614417201,-22.6985303271799),
 .UNSPECIFIED.);
#513=B_SPLINE_CURVE_WITH_KNOTS('',3,(#19068,#19069,#19070,#19071,#19072,
#19073,#19074,#19075,#19076,#19077,#19078,#19079,#19080,#19081,#19082,#19083,
#19084,#19085,#19086,#19087,#19088,#19089),.UNSPECIFIED.,.F.,.F.,(4,3,3,
3,3,3,3,4),(20.1591190625158,20.7156787615051,21.7021396549101,22.6886005483151,
23.6750614417201,24.6615223351251,25.6479832285301,26.4423043696954),
 .UNSPECIFIED.);
#514=B_SPLINE_CURVE_WITH_KNOTS('',3,(#19090,#19091,#19092,#19093,#19094,
#19095,#19096,#19097,#19098,#19099,#19100,#19101,#19102,#19103,#19104,#19105,
#19106,#19107,#19108,#19109,#19110,#19111,#19112,#19113,#19114),
 .UNSPECIFIED.,.F.,.F.,(4,3,3,3,3,3,3,3,4),(-22.6985303271799,-22.6886005483151,
-21.7021396549101,-20.7156787615051,-19.7292178681001,-18.7427569746951,
-17.7562960812901,-16.7698351878851,-16.4153450200003),.UNSPECIFIED.);
#515=B_SPLINE_CURVE_WITH_KNOTS('',3,(#19119,#19120,#19121,#19122,#19123,
#19124,#19125,#19126,#19127,#19128,#19129,#19130,#19131,#19132,#19133,#19134,
#19135,#19136,#19137,#19138,#19139,#19140),.UNSPECIFIED.,.F.,.F.,(4,3,3,
3,3,3,3,4),(13.8759337553363,14.796913401075,15.78337429448,16.7698351878851,
17.7562960812901,18.7427569746951,19.7292178681001,20.1591190625158),
 .UNSPECIFIED.);
#516=B_SPLINE_CURVE_WITH_KNOTS('',3,(#19141,#19142,#19143,#19144,#19145,
#19146,#19147,#19148,#19149,#19150,#19151,#19152,#19153,#19154,#19155,#19156,
#19157,#19158,#19159,#19160,#19161,#19162),.UNSPECIFIED.,.F.,.F.,(4,3,3,
3,3,3,3,4),(-16.4153450200003,-15.7833742944801,-14.796913401075,-13.81045250767,
-12.823991614265,-11.83753072086,-10.851069827455,-10.1321597128207),
 .UNSPECIFIED.);
#517=B_SPLINE_CURVE_WITH_KNOTS('',3,(#19168,#19169,#19170,#19171,#19172,
#19173,#19174,#19175,#19176,#19177,#19178,#19179,#19180),.UNSPECIFIED.,
 .F.,.F.,(4,3,3,3,4),(-3.84897440564114,-2.95938268021501,-1.97292178681001,
-0.986460893405001,0.),.UNSPECIFIED.);
#518=B_SPLINE_CURVE_WITH_KNOTS('',3,(#19183,#19184,#19185,#19186,#19187,
#19188,#19189,#19190,#19191,#19192,#19193,#19194,#19195,#19196,#19197,#19198,
#19199,#19200,#19201),.UNSPECIFIED.,.F.,.F.,(4,3,3,3,3,3,4),(2.01694489302845,
2.95938268021501,3.94584357362001,4.93230446702501,5.91876536043001,6.90522625383501,
7.59274844815667),.UNSPECIFIED.);
#519=B_SPLINE_CURVE_WITH_KNOTS('',3,(#19207,#19208,#19209,#19210),
 .UNSPECIFIED.,.F.,.F.,(4,4),(51.5750455984138,52.2824273504652),
 .UNSPECIFIED.);
#520=B_SPLINE_CURVE_WITH_KNOTS('',3,(#19213,#19214,#19215,#19216,#19217,
#19218,#19219,#19220,#19221,#19222),.UNSPECIFIED.,.F.,.F.,(4,3,3,4),(-50.2654824574367,
-49.3230446702501,-48.3365837768451,-47.8312715558982),.UNSPECIFIED.);
#521=B_SPLINE_CURVE_WITH_KNOTS('',3,(#19227,#19228,#19229,#19230,#19231,
#19232,#19233,#19234,#19235,#19236,#19237,#19238,#19239,#19240,#19241,#19242,
#19243,#19244,#19245,#19246,#19247,#19248,#19249,#19250,#19251),
 .UNSPECIFIED.,.F.,.F.,(4,3,3,3,3,3,3,3,4),(45.2918602912342,45.3772010966301,
46.3636619900351,47.3501228834401,48.3365837768451,49.3230446702501,50.3095055636552,
51.2959664570602,51.5750455984138),.UNSPECIFIED.);
#522=B_SPLINE_CURVE_WITH_KNOTS('',3,(#19252,#19253,#19254,#19255,#19256,
#19257,#19258,#19259,#19260,#19261,#19262,#19263,#19264,#19265,#19266,#19267,
#19268,#19269,#19270,#19271,#19272,#19273),.UNSPECIFIED.,.F.,.F.,(4,3,3,
3,3,3,3,4),(-47.8312715558982,-47.3501228834401,-46.3636619900351,-45.3772010966301,
-44.3907402032251,-43.4042793098201,-42.4178184164151,-41.5480862487187),
 .UNSPECIFIED.);
#523=B_SPLINE_CURVE_WITH_KNOTS('',3,(#19278,#19279,#19280,#19281,#19282,
#19283,#19284,#19285,#19286,#19287,#19288,#19289,#19290,#19291,#19292,#19293,
#19294,#19295,#19296,#19297,#19298,#19299),.UNSPECIFIED.,.F.,.F.,(4,3,3,
3,3,3,3,4),(39.0086749840546,39.4584357362001,40.4448966296051,41.4313575230101,
42.4178184164151,43.4042793098201,44.3907402032251,45.2918602912342),
 .UNSPECIFIED.);
#524=B_SPLINE_CURVE_WITH_KNOTS('',3,(#19300,#19301,#19302,#19303,#19304,
#19305,#19306,#19307,#19308,#19309,#19310,#19311,#19312,#19313,#19314,#19315,
#19316,#19317,#19318,#19319,#19320,#19321,#19322,#19323,#19324),
 .UNSPECIFIED.,.F.,.F.,(4,3,3,3,3,3,3,3,4),(-41.5480862487187,-41.4313575230101,
-40.4448966296051,-39.4584357362001,-38.4719748427951,-37.4855139493901,
-36.4990530559851,-35.5125921625801,-35.2649009415391),.UNSPECIFIED.);
#525=B_SPLINE_CURVE_WITH_KNOTS('',3,(#19329,#19330,#19331,#19332,#19333,
#19334,#19335,#19336,#19337,#19338,#19339,#19340,#19341,#19342,#19343,#19344,
#19345,#19346,#19347,#19348,#19349,#19350),.UNSPECIFIED.,.F.,.F.,(4,3,3,
3,3,3,3,4),(32.725489676875,33.5396703757701,34.5261312691751,35.5125921625801,
36.4990530559851,37.4855139493901,38.4719748427951,39.0086749840546),
 .UNSPECIFIED.);
#526=B_SPLINE_CURVE_WITH_KNOTS('',3,(#19351,#19352,#19353,#19354,#19355,
#19356,#19357,#19358,#19359,#19360,#19361,#19362,#19363,#19364,#19365,#19366,
#19367,#19368,#19369,#19370,#19371,#19372),.UNSPECIFIED.,.F.,.F.,(4,3,3,
3,3,3,3,4),(-35.2649009415391,-34.5261312691751,-33.5396703757701,-32.5532094823651,
-31.5667485889601,-30.5802876955551,-29.5938268021501,-28.9817156343595),
 .UNSPECIFIED.);
#527=B_SPLINE_CURVE_WITH_KNOTS('',3,(#19377,#19378,#19379,#19380,#19381,
#19382,#19383,#19384,#19385,#19386,#19387,#19388,#19389,#19390,#19391,#19392,
#19393,#19394,#19395,#19396,#19397,#19398,#19399,#19400,#19401),
 .UNSPECIFIED.,.F.,.F.,(4,3,3,3,3,3,3,3,4),(26.4423043696954,26.6344441219351,
27.6209050153401,28.6073659087451,29.5938268021501,30.5802876955551,31.5667485889601,
32.5532094823651,32.725489676875),.UNSPECIFIED.);
#528=B_SPLINE_CURVE_WITH_KNOTS('',3,(#19402,#19403,#19404,#19405,#19406,
#19407,#19408,#19409,#19410,#19411,#19412,#19413,#19414,#19415,#19416,#19417,
#19418,#19419,#19420,#19421,#19422,#19423),.UNSPECIFIED.,.F.,.F.,(4,3,3,
3,3,3,3,4),(-28.9817156343595,-28.6073659087451,-27.6209050153401,-26.6344441219351,
-25.6479832285301,-24.6615223351251,-23.6750614417201,-22.6985303271799),
 .UNSPECIFIED.);
#529=B_SPLINE_CURVE_WITH_KNOTS('',3,(#19428,#19429,#19430,#19431,#19432,
#19433,#19434,#19435,#19436,#19437,#19438,#19439,#19440,#19441,#19442,#19443,
#19444,#19445,#19446,#19447,#19448,#19449),.UNSPECIFIED.,.F.,.F.,(4,3,3,
3,3,3,3,4),(20.1591190625158,20.7156787615051,21.7021396549101,22.6886005483151,
23.6750614417201,24.6615223351251,25.6479832285301,26.4423043696954),
 .UNSPECIFIED.);
#530=B_SPLINE_CURVE_WITH_KNOTS('',3,(#19450,#19451,#19452,#19453,#19454,
#19455,#19456,#19457,#19458,#19459,#19460,#19461,#19462,#19463,#19464,#19465,
#19466,#19467,#19468,#19469,#19470,#19471,#19472,#19473,#19474),
 .UNSPECIFIED.,.F.,.F.,(4,3,3,3,3,3,3,3,4),(-22.6985303271799,-22.6886005483151,
-21.7021396549101,-20.715678761505,-19.7292178681001,-18.742756974695,-17.75629608129,
-16.769835187885,-16.4153450200003),.UNSPECIFIED.);
#531=B_SPLINE_CURVE_WITH_KNOTS('',3,(#19479,#19480,#19481,#19482,#19483,
#19484,#19485,#19486,#19487,#19488,#19489,#19490,#19491,#19492,#19493,#19494,
#19495,#19496,#19497,#19498,#19499,#19500),.UNSPECIFIED.,.F.,.F.,(4,3,3,
3,3,3,3,4),(13.8759337553363,14.796913401075,15.78337429448,16.7698351878851,
17.7562960812901,18.7427569746951,19.7292178681001,20.1591190625158),
 .UNSPECIFIED.);
#532=B_SPLINE_CURVE_WITH_KNOTS('',3,(#19501,#19502,#19503,#19504,#19505,
#19506,#19507,#19508,#19509,#19510,#19511,#19512,#19513,#19514,#19515,#19516,
#19517,#19518,#19519,#19520,#19521,#19522),.UNSPECIFIED.,.F.,.F.,(4,3,3,
3,3,3,3,4),(-16.4153450200003,-15.78337429448,-14.796913401075,-13.81045250767,
-12.823991614265,-11.83753072086,-10.851069827455,-10.1321597128207),
 .UNSPECIFIED.);
#533=B_SPLINE_CURVE_WITH_KNOTS('',3,(#19528,#19529,#19530,#19531,#19532,
#19533,#19534,#19535,#19536,#19537,#19538,#19539,#19540),.UNSPECIFIED.,
 .F.,.F.,(4,3,3,3,4),(-3.84897440564114,-2.95938268021501,-1.97292178681001,
-0.986460893405004,0.),.UNSPECIFIED.);
#534=B_SPLINE_CURVE_WITH_KNOTS('',3,(#19543,#19544,#19545,#19546,#19547,
#19548,#19549,#19550,#19551,#19552,#19553,#19554,#19555,#19556,#19557,#19558,
#19559,#19560,#19561),.UNSPECIFIED.,.F.,.F.,(4,3,3,3,3,3,4),(2.01694489302844,
2.95938268021501,3.94584357362001,4.93230446702501,5.91876536043001,6.90522625383502,
7.59274844815667),.UNSPECIFIED.);
#535=B_SPLINE_CURVE_WITH_KNOTS('',3,(#19567,#19568,#19569,#19570),
 .UNSPECIFIED.,.F.,.F.,(4,4),(51.5750455984138,52.2824273504652),
 .UNSPECIFIED.);
#536=B_SPLINE_CURVE_WITH_KNOTS('',3,(#19573,#19574,#19575,#19576,#19577,
#19578,#19579,#19580,#19581,#19582),.UNSPECIFIED.,.F.,.F.,(4,3,3,4),(-50.2654824574367,
-49.3230446702501,-48.3365837768451,-47.8312715558983),.UNSPECIFIED.);
#537=B_SPLINE_CURVE_WITH_KNOTS('',3,(#19587,#19588,#19589,#19590,#19591,
#19592,#19593,#19594,#19595,#19596,#19597,#19598,#19599,#19600,#19601,#19602,
#19603,#19604,#19605,#19606,#19607,#19608,#19609,#19610,#19611),
 .UNSPECIFIED.,.F.,.F.,(4,3,3,3,3,3,3,3,4),(45.2918602912342,45.3772010966301,
46.3636619900351,47.3501228834401,48.3365837768452,49.3230446702501,50.3095055636552,
51.2959664570602,51.5750455984138),.UNSPECIFIED.);
#538=B_SPLINE_CURVE_WITH_KNOTS('',3,(#19612,#19613,#19614,#19615,#19616,
#19617,#19618,#19619,#19620,#19621,#19622,#19623,#19624,#19625,#19626,#19627,
#19628,#19629,#19630,#19631,#19632,#19633),.UNSPECIFIED.,.F.,.F.,(4,3,3,
3,3,3,3,4),(-47.8312715558983,-47.3501228834401,-46.3636619900351,-45.3772010966301,
-44.3907402032251,-43.4042793098201,-42.4178184164151,-41.5480862487187),
 .UNSPECIFIED.);
#539=B_SPLINE_CURVE_WITH_KNOTS('',3,(#19638,#19639,#19640,#19641,#19642,
#19643,#19644,#19645,#19646,#19647,#19648,#19649,#19650,#19651,#19652,#19653,
#19654,#19655,#19656,#19657,#19658,#19659),.UNSPECIFIED.,.F.,.F.,(4,3,3,
3,3,3,3,4),(39.0086749840546,39.4584357362001,40.4448966296051,41.4313575230101,
42.4178184164151,43.4042793098201,44.3907402032251,45.2918602912342),
 .UNSPECIFIED.);
#540=B_SPLINE_CURVE_WITH_KNOTS('',3,(#19660,#19661,#19662,#19663,#19664,
#19665,#19666,#19667,#19668,#19669,#19670,#19671,#19672,#19673,#19674,#19675,
#19676,#19677,#19678,#19679,#19680,#19681,#19682,#19683,#19684),
 .UNSPECIFIED.,.F.,.F.,(4,3,3,3,3,3,3,3,4),(-41.5480862487187,-41.4313575230101,
-40.4448966296051,-39.4584357362001,-38.4719748427951,-37.4855139493901,
-36.4990530559851,-35.5125921625801,-35.2649009415391),.UNSPECIFIED.);
#541=B_SPLINE_CURVE_WITH_KNOTS('',3,(#19689,#19690,#19691,#19692,#19693,
#19694,#19695,#19696,#19697,#19698,#19699,#19700,#19701,#19702,#19703,#19704,
#19705,#19706,#19707,#19708,#19709,#19710),.UNSPECIFIED.,.F.,.F.,(4,3,3,
3,3,3,3,4),(32.725489676875,33.5396703757701,34.5261312691751,35.5125921625801,
36.4990530559851,37.4855139493901,38.4719748427951,39.0086749840546),
 .UNSPECIFIED.);
#542=B_SPLINE_CURVE_WITH_KNOTS('',3,(#19711,#19712,#19713,#19714,#19715,
#19716,#19717,#19718,#19719,#19720,#19721,#19722,#19723,#19724,#19725,#19726,
#19727,#19728,#19729,#19730,#19731,#19732),.UNSPECIFIED.,.F.,.F.,(4,3,3,
3,3,3,3,4),(-35.2649009415391,-34.5261312691751,-33.5396703757701,-32.5532094823651,
-31.5667485889601,-30.5802876955551,-29.5938268021501,-28.9817156343595),
 .UNSPECIFIED.);
#543=B_SPLINE_CURVE_WITH_KNOTS('',3,(#19737,#19738,#19739,#19740,#19741,
#19742,#19743,#19744,#19745,#19746,#19747,#19748,#19749,#19750,#19751,#19752,
#19753,#19754,#19755,#19756,#19757,#19758,#19759,#19760,#19761),
 .UNSPECIFIED.,.F.,.F.,(4,3,3,3,3,3,3,3,4),(26.4423043696954,26.6344441219351,
27.6209050153401,28.6073659087451,29.5938268021501,30.5802876955551,31.5667485889601,
32.5532094823651,32.725489676875),.UNSPECIFIED.);
#544=B_SPLINE_CURVE_WITH_KNOTS('',3,(#19762,#19763,#19764,#19765,#19766,
#19767,#19768,#19769,#19770,#19771,#19772,#19773,#19774,#19775,#19776,#19777,
#19778,#19779,#19780,#19781,#19782,#19783),.UNSPECIFIED.,.F.,.F.,(4,3,3,
3,3,3,3,4),(-28.9817156343595,-28.6073659087451,-27.6209050153401,-26.6344441219351,
-25.6479832285301,-24.6615223351251,-23.6750614417201,-22.6985303271799),
 .UNSPECIFIED.);
#545=B_SPLINE_CURVE_WITH_KNOTS('',3,(#19788,#19789,#19790,#19791,#19792,
#19793,#19794,#19795,#19796,#19797,#19798,#19799,#19800,#19801,#19802,#19803,
#19804,#19805,#19806,#19807,#19808,#19809),.UNSPECIFIED.,.F.,.F.,(4,3,3,
3,3,3,3,4),(20.1591190625159,20.7156787615051,21.7021396549101,22.6886005483151,
23.6750614417201,24.6615223351251,25.6479832285301,26.4423043696954),
 .UNSPECIFIED.);
#546=B_SPLINE_CURVE_WITH_KNOTS('',3,(#19810,#19811,#19812,#19813,#19814,
#19815,#19816,#19817,#19818,#19819,#19820,#19821,#19822,#19823,#19824,#19825,
#19826,#19827,#19828,#19829,#19830,#19831,#19832,#19833,#19834),
 .UNSPECIFIED.,.F.,.F.,(4,3,3,3,3,3,3,3,4),(-22.6985303271799,-22.6886005483151,
-21.7021396549101,-20.7156787615051,-19.7292178681001,-18.7427569746951,
-17.7562960812901,-16.7698351878851,-16.4153450200003),.UNSPECIFIED.);
#547=B_SPLINE_CURVE_WITH_KNOTS('',3,(#19839,#19840,#19841,#19842,#19843,
#19844,#19845,#19846,#19847,#19848,#19849,#19850,#19851,#19852,#19853,#19854,
#19855,#19856,#19857,#19858,#19859,#19860),.UNSPECIFIED.,.F.,.F.,(4,3,3,
3,3,3,3,4),(13.8759337553363,14.7969134010751,15.78337429448,16.7698351878851,
17.75629608129,18.7427569746951,19.7292178681001,20.1591190625159),
 .UNSPECIFIED.);
#548=B_SPLINE_CURVE_WITH_KNOTS('',3,(#19861,#19862,#19863,#19864,#19865,
#19866,#19867,#19868,#19869,#19870,#19871,#19872,#19873,#19874,#19875,#19876,
#19877,#19878,#19879,#19880,#19881,#19882),.UNSPECIFIED.,.F.,.F.,(4,3,3,
3,3,3,3,4),(-16.4153450200003,-15.78337429448,-14.796913401075,-13.81045250767,
-12.823991614265,-11.83753072086,-10.851069827455,-10.1321597128207),
 .UNSPECIFIED.);
#549=B_SPLINE_CURVE_WITH_KNOTS('',3,(#19888,#19889,#19890,#19891,#19892,
#19893,#19894,#19895,#19896,#19897,#19898,#19899,#19900),.UNSPECIFIED.,
 .F.,.F.,(4,3,3,3,4),(-3.84897440564115,-2.95938268021501,-1.97292178681001,
-0.986460893405001,0.),.UNSPECIFIED.);
#550=B_SPLINE_CURVE_WITH_KNOTS('',3,(#19903,#19904,#19905,#19906,#19907,
#19908,#19909,#19910,#19911,#19912,#19913,#19914,#19915,#19916,#19917,#19918,
#19919,#19920,#19921),.UNSPECIFIED.,.F.,.F.,(4,3,3,3,3,3,4),(2.01694489302845,
2.95938268021501,3.94584357362001,4.93230446702501,5.91876536043001,6.90522625383502,
7.59274844815668),.UNSPECIFIED.);
#551=B_SPLINE_CURVE_WITH_KNOTS('',3,(#19927,#19928,#19929,#19930,#19931,
#19932,#19933,#19934),.UNSPECIFIED.,.F.,.F.,(4,1,1,1,1,4),(59.6902604182061,
60.1955726391529,61.1820335325579,62.1684944259629,63.154955319368,64.141416212773),
 .UNSPECIFIED.);
#552=B_SPLINE_CURVE_WITH_KNOTS('',3,(#19937,#19938,#19939,#19940,#19941,
#19942,#19943,#19944,#19945),.UNSPECIFIED.,.F.,.F.,(4,1,1,1,1,1,4),(59.6902604182061,
59.775601223602,60.762062117007,61.748523010412,62.734983903817,63.721444797222,
64.6638825844085),.UNSPECIFIED.);
#553=B_SPLINE_CURVE_WITH_KNOTS('',3,(#19950,#19951,#19952,#19953,#19954,
#19955,#19956,#19957,#19958,#19959),.UNSPECIFIED.,.F.,.F.,(4,1,1,1,1,1,
1,4),(53.4070751110265,54.2768072787229,55.2632681721279,56.2497290655329,
57.2361899589379,58.2226508523429,59.2091117457479,59.6902604182061),
 .UNSPECIFIED.);
#554=B_SPLINE_CURVE_WITH_KNOTS('',3,(#19960,#19961,#19962,#19963,#19964,
#19965,#19966,#19967,#19968,#19969),.UNSPECIFIED.,.F.,.F.,(4,1,1,1,1,1,
1,4),(53.4070751110265,53.856835863172,54.843296756577,55.829757649982,
56.816218543387,57.802679436792,58.789140330197,59.6902604182061),
 .UNSPECIFIED.);
#555=B_SPLINE_CURVE_WITH_KNOTS('',3,(#19974,#19975,#19976,#19977,#19978,
#19979,#19980,#19981,#19982,#19983,#19984),.UNSPECIFIED.,.F.,.F.,(4,1,1,
1,1,1,1,1,4),(47.1238898038469,47.3715810248879,48.3580419182929,49.3445028116979,
50.3309637051029,51.3174245985079,52.3038854919129,53.2903463853179,53.4070751110265),
 .UNSPECIFIED.);
#556=B_SPLINE_CURVE_WITH_KNOTS('',3,(#19985,#19986,#19987,#19988,#19989,
#19990,#19991,#19992,#19993,#19994),.UNSPECIFIED.,.F.,.F.,(4,1,1,1,1,1,
1,4),(47.1238898038469,47.9380705027419,48.9245313961469,49.9109922895519,
50.8974531829569,51.8839140763619,52.8703749697669,53.4070751110265),
 .UNSPECIFIED.);
#557=B_SPLINE_CURVE_WITH_KNOTS('',3,(#19999,#20000,#20001,#20002,#20003,
#20004,#20005,#20006,#20007,#20008),.UNSPECIFIED.,.F.,.F.,(4,1,1,1,1,1,
1,4),(40.8407044966673,41.4528156644579,42.4392765578629,43.4257374512679,
44.4121983446729,45.3986592380779,46.3851201314829,47.1238898038469),
 .UNSPECIFIED.);
#558=B_SPLINE_CURVE_WITH_KNOTS('',3,(#20009,#20010,#20011,#20012,#20013,
#20014,#20015,#20016,#20017,#20018,#20019),.UNSPECIFIED.,.F.,.F.,(4,1,1,
1,1,1,1,1,4),(40.8407044966673,41.0328442489069,42.0193051423119,43.0057660357169,
43.9922269291219,44.9786878225269,45.9651487159319,46.9516096093369,47.1238898038469),
 .UNSPECIFIED.);
#559=B_SPLINE_CURVE_WITH_KNOTS('',3,(#20024,#20025,#20026,#20027,#20028,
#20029,#20030,#20031,#20032,#20033),.UNSPECIFIED.,.F.,.F.,(4,1,1,1,1,1,
1,4),(34.5575191894877,35.5340503040279,36.5205111974329,37.5069720908379,
38.4934329842429,39.4798938776479,40.4663547710529,40.8407044966673),
 .UNSPECIFIED.);
#560=B_SPLINE_CURVE_WITH_KNOTS('',3,(#20034,#20035,#20036,#20037,#20038,
#20039,#20040,#20041,#20042,#20043),.UNSPECIFIED.,.F.,.F.,(4,1,1,1,1,1,
1,4),(34.5575191894877,35.1140788884769,36.1005397818819,37.0870006752869,
38.0734615686919,39.0599224620969,40.0463833555019,40.8407044966673),
 .UNSPECIFIED.);
#561=B_SPLINE_CURVE_WITH_KNOTS('',3,(#20048,#20049,#20050,#20051,#20052,
#20053,#20054,#20055,#20056,#20057,#20058),.UNSPECIFIED.,.F.,.F.,(4,1,1,
1,1,1,1,1,4),(28.2743338823081,28.6288240501929,29.6152849435979,30.6017458370029,
31.5882067304079,32.5746676238129,33.5611285172179,34.5475894106229,34.5575191894877),
 .UNSPECIFIED.);
#562=B_SPLINE_CURVE_WITH_KNOTS('',3,(#20059,#20060,#20061,#20062,#20063,
#20064,#20065,#20066,#20067,#20068),.UNSPECIFIED.,.F.,.F.,(4,1,1,1,1,1,
1,4),(28.2743338823081,29.1953135280469,30.1817744214519,31.1682353148569,
32.1546962082619,33.1411571016669,34.1276179950719,34.5575191894877),
 .UNSPECIFIED.);
#563=B_SPLINE_CURVE_WITH_KNOTS('',3,(#20073,#20074,#20075,#20076,#20077,
#20078,#20079,#20080,#20081,#20082),.UNSPECIFIED.,.F.,.F.,(4,1,1,1,1,1,
1,4),(21.9911485751285,22.7100586897628,23.6965195831678,24.6829804765728,
25.6694413699778,26.6559022633828,27.6423631567879,28.2743338823081),
 .UNSPECIFIED.);
#564=B_SPLINE_CURVE_WITH_KNOTS('',3,(#20083,#20084,#20085,#20086,#20087,
#20088,#20089,#20090,#20091,#20092,#20093),.UNSPECIFIED.,.F.,.F.,(4,1,1,
1,1,1,1,1,4),(21.9911485751285,22.2900872742119,23.2765481676169,24.2630090610219,
25.2494699544269,26.2359308478319,27.2223917412369,28.2088526346419,28.2743338823081),
 .UNSPECIFIED.);
#565=B_SPLINE_CURVE_WITH_KNOTS('',3,(#20099,#20100,#20101,#20102,#20103),
 .UNSPECIFIED.,.F.,.F.,(4,1,4),(14.3984001269718,15.3848610203768,15.7079632679489),
 .UNSPECIFIED.);
#566=B_SPLINE_CURVE_WITH_KNOTS('',3,(#20106,#20107,#20108,#20109,#20110),
 .UNSPECIFIED.,.F.,.F.,(4,1,4),(13.8759337553363,14.8183715425228,15.7079632679489),
 .UNSPECIFIED.);
#567=B_SPLINE_CURVE_WITH_KNOTS('',3,(#20116,#20117,#20118,#20119,#20120,
#20121,#20122,#20123),.UNSPECIFIED.,.F.,.F.,(4,1,1,1,1,4),(59.6902604182061,
60.1955726391529,61.1820335325579,62.1684944259629,63.1549553193679,64.1414162127729),
 .UNSPECIFIED.);
#568=B_SPLINE_CURVE_WITH_KNOTS('',3,(#20126,#20127,#20128,#20129,#20130,
#20131,#20132,#20133,#20134),.UNSPECIFIED.,.F.,.F.,(4,1,1,1,1,1,4),(59.6902604182061,
59.775601223602,60.762062117007,61.748523010412,62.734983903817,63.721444797222,
64.6638825844085),.UNSPECIFIED.);
#569=B_SPLINE_CURVE_WITH_KNOTS('',3,(#20139,#20140,#20141,#20142,#20143,
#20144,#20145,#20146,#20147,#20148),.UNSPECIFIED.,.F.,.F.,(4,1,1,1,1,1,
1,4),(53.4070751110265,54.2768072787229,55.2632681721279,56.2497290655329,
57.2361899589379,58.2226508523429,59.2091117457479,59.6902604182061),
 .UNSPECIFIED.);
#570=B_SPLINE_CURVE_WITH_KNOTS('',3,(#20149,#20150,#20151,#20152,#20153,
#20154,#20155,#20156,#20157,#20158),.UNSPECIFIED.,.F.,.F.,(4,1,1,1,1,1,
1,4),(53.4070751110265,53.856835863172,54.843296756577,55.829757649982,
56.816218543387,57.802679436792,58.789140330197,59.6902604182061),
 .UNSPECIFIED.);
#571=B_SPLINE_CURVE_WITH_KNOTS('',3,(#20163,#20164,#20165,#20166,#20167,
#20168,#20169,#20170,#20171,#20172,#20173),.UNSPECIFIED.,.F.,.F.,(4,1,1,
1,1,1,1,1,4),(47.1238898038469,47.3715810248879,48.3580419182929,49.3445028116979,
50.3309637051029,51.3174245985079,52.3038854919129,53.2903463853179,53.4070751110265),
 .UNSPECIFIED.);
#572=B_SPLINE_CURVE_WITH_KNOTS('',3,(#20174,#20175,#20176,#20177,#20178,
#20179,#20180,#20181,#20182,#20183),.UNSPECIFIED.,.F.,.F.,(4,1,1,1,1,1,
1,4),(47.1238898038469,47.9380705027419,48.9245313961469,49.9109922895519,
50.8974531829569,51.8839140763619,52.8703749697669,53.4070751110265),
 .UNSPECIFIED.);
#573=B_SPLINE_CURVE_WITH_KNOTS('',3,(#20188,#20189,#20190,#20191,#20192,
#20193,#20194,#20195,#20196,#20197),.UNSPECIFIED.,.F.,.F.,(4,1,1,1,1,1,
1,4),(40.8407044966673,41.4528156644579,42.4392765578629,43.4257374512679,
44.4121983446729,45.3986592380779,46.3851201314829,47.1238898038469),
 .UNSPECIFIED.);
#574=B_SPLINE_CURVE_WITH_KNOTS('',3,(#20198,#20199,#20200,#20201,#20202,
#20203,#20204,#20205,#20206,#20207,#20208),.UNSPECIFIED.,.F.,.F.,(4,1,1,
1,1,1,1,1,4),(40.8407044966673,41.0328442489069,42.0193051423119,43.0057660357169,
43.9922269291219,44.9786878225269,45.9651487159319,46.9516096093369,47.1238898038469),
 .UNSPECIFIED.);
#575=B_SPLINE_CURVE_WITH_KNOTS('',3,(#20213,#20214,#20215,#20216,#20217,
#20218,#20219,#20220,#20221,#20222),.UNSPECIFIED.,.F.,.F.,(4,1,1,1,1,1,
1,4),(34.5575191894877,35.5340503040279,36.5205111974329,37.5069720908379,
38.4934329842429,39.4798938776479,40.4663547710529,40.8407044966673),
 .UNSPECIFIED.);
#576=B_SPLINE_CURVE_WITH_KNOTS('',3,(#20223,#20224,#20225,#20226,#20227,
#20228,#20229,#20230,#20231,#20232),.UNSPECIFIED.,.F.,.F.,(4,1,1,1,1,1,
1,4),(34.5575191894877,35.1140788884769,36.1005397818819,37.0870006752869,
38.0734615686919,39.0599224620969,40.0463833555019,40.8407044966673),
 .UNSPECIFIED.);
#577=B_SPLINE_CURVE_WITH_KNOTS('',3,(#20237,#20238,#20239,#20240,#20241,
#20242,#20243,#20244,#20245,#20246,#20247),.UNSPECIFIED.,.F.,.F.,(4,1,1,
1,1,1,1,1,4),(28.2743338823081,28.6288240501928,29.6152849435978,30.6017458370028,
31.5882067304078,32.5746676238129,33.5611285172179,34.5475894106229,34.5575191894877),
 .UNSPECIFIED.);
#578=B_SPLINE_CURVE_WITH_KNOTS('',3,(#20248,#20249,#20250,#20251,#20252,
#20253,#20254,#20255,#20256,#20257),.UNSPECIFIED.,.F.,.F.,(4,1,1,1,1,1,
1,4),(28.2743338823081,29.1953135280469,30.1817744214519,31.1682353148569,
32.1546962082619,33.1411571016669,34.1276179950719,34.5575191894877),
 .UNSPECIFIED.);
#579=B_SPLINE_CURVE_WITH_KNOTS('',3,(#20262,#20263,#20264,#20265,#20266,
#20267,#20268,#20269,#20270,#20271),.UNSPECIFIED.,.F.,.F.,(4,1,1,1,1,1,
1,4),(21.9911485751285,22.7100586897628,23.6965195831678,24.6829804765728,
25.6694413699778,26.6559022633828,27.6423631567878,28.2743338823081),
 .UNSPECIFIED.);
#580=B_SPLINE_CURVE_WITH_KNOTS('',3,(#20272,#20273,#20274,#20275,#20276,
#20277,#20278,#20279,#20280,#20281,#20282),.UNSPECIFIED.,.F.,.F.,(4,1,1,
1,1,1,1,1,4),(21.9911485751285,22.2900872742119,23.2765481676169,24.2630090610219,
25.2494699544269,26.2359308478319,27.2223917412369,28.2088526346419,28.2743338823081),
 .UNSPECIFIED.);
#581=B_SPLINE_CURVE_WITH_KNOTS('',3,(#20288,#20289,#20290,#20291,#20292),
 .UNSPECIFIED.,.F.,.F.,(4,1,4),(14.3984001269718,15.3848610203768,15.7079632679489),
 .UNSPECIFIED.);
#582=B_SPLINE_CURVE_WITH_KNOTS('',3,(#20295,#20296,#20297,#20298,#20299),
 .UNSPECIFIED.,.F.,.F.,(4,1,4),(13.8759337553362,14.8183715425228,15.707963267949),
 .UNSPECIFIED.);
#583=B_SPLINE_CURVE_WITH_KNOTS('',3,(#20305,#20306,#20307,#20308,#20309,
#20310,#20311,#20312),.UNSPECIFIED.,.F.,.F.,(4,1,1,1,1,4),(59.6902604182061,
60.1955726391529,61.1820335325579,62.1684944259629,63.154955319368,64.141416212773),
 .UNSPECIFIED.);
#584=B_SPLINE_CURVE_WITH_KNOTS('',3,(#20315,#20316,#20317,#20318,#20319,
#20320,#20321,#20322,#20323),.UNSPECIFIED.,.F.,.F.,(4,1,1,1,1,1,4),(59.6902604182061,
59.775601223602,60.762062117007,61.748523010412,62.734983903817,63.721444797222,
64.6638825844085),.UNSPECIFIED.);
#585=B_SPLINE_CURVE_WITH_KNOTS('',3,(#20328,#20329,#20330,#20331,#20332,
#20333,#20334,#20335,#20336,#20337),.UNSPECIFIED.,.F.,.F.,(4,1,1,1,1,1,
1,4),(53.4070751110265,54.2768072787229,55.2632681721279,56.2497290655329,
57.2361899589379,58.2226508523429,59.2091117457479,59.6902604182061),
 .UNSPECIFIED.);
#586=B_SPLINE_CURVE_WITH_KNOTS('',3,(#20338,#20339,#20340,#20341,#20342,
#20343,#20344,#20345,#20346,#20347),.UNSPECIFIED.,.F.,.F.,(4,1,1,1,1,1,
1,4),(53.4070751110265,53.856835863172,54.843296756577,55.829757649982,
56.816218543387,57.802679436792,58.789140330197,59.6902604182061),
 .UNSPECIFIED.);
#587=B_SPLINE_CURVE_WITH_KNOTS('',3,(#20352,#20353,#20354,#20355,#20356,
#20357,#20358,#20359,#20360,#20361,#20362),.UNSPECIFIED.,.F.,.F.,(4,1,1,
1,1,1,1,1,4),(47.1238898038469,47.3715810248879,48.3580419182929,49.3445028116979,
50.3309637051029,51.3174245985079,52.3038854919129,53.2903463853179,53.4070751110265),
 .UNSPECIFIED.);
#588=B_SPLINE_CURVE_WITH_KNOTS('',3,(#20363,#20364,#20365,#20366,#20367,
#20368,#20369,#20370,#20371,#20372),.UNSPECIFIED.,.F.,.F.,(4,1,1,1,1,1,
1,4),(47.1238898038469,47.9380705027419,48.9245313961469,49.9109922895519,
50.8974531829569,51.8839140763619,52.8703749697669,53.4070751110265),
 .UNSPECIFIED.);
#589=B_SPLINE_CURVE_WITH_KNOTS('',3,(#20377,#20378,#20379,#20380,#20381,
#20382,#20383,#20384,#20385,#20386),.UNSPECIFIED.,.F.,.F.,(4,1,1,1,1,1,
1,4),(40.8407044966673,41.4528156644579,42.4392765578629,43.4257374512679,
44.4121983446729,45.3986592380779,46.3851201314829,47.1238898038469),
 .UNSPECIFIED.);
#590=B_SPLINE_CURVE_WITH_KNOTS('',3,(#20387,#20388,#20389,#20390,#20391,
#20392,#20393,#20394,#20395,#20396,#20397),.UNSPECIFIED.,.F.,.F.,(4,1,1,
1,1,1,1,1,4),(40.8407044966673,41.0328442489069,42.0193051423119,43.0057660357169,
43.9922269291219,44.9786878225269,45.9651487159319,46.9516096093369,47.1238898038469),
 .UNSPECIFIED.);
#591=B_SPLINE_CURVE_WITH_KNOTS('',3,(#20402,#20403,#20404,#20405,#20406,
#20407,#20408,#20409,#20410,#20411),.UNSPECIFIED.,.F.,.F.,(4,1,1,1,1,1,
1,4),(34.5575191894877,35.5340503040279,36.5205111974329,37.5069720908379,
38.4934329842429,39.4798938776479,40.4663547710529,40.8407044966673),
 .UNSPECIFIED.);
#592=B_SPLINE_CURVE_WITH_KNOTS('',3,(#20412,#20413,#20414,#20415,#20416,
#20417,#20418,#20419,#20420,#20421),.UNSPECIFIED.,.F.,.F.,(4,1,1,1,1,1,
1,4),(34.5575191894877,35.1140788884769,36.1005397818819,37.0870006752869,
38.0734615686919,39.0599224620969,40.0463833555019,40.8407044966673),
 .UNSPECIFIED.);
#593=B_SPLINE_CURVE_WITH_KNOTS('',3,(#20426,#20427,#20428,#20429,#20430,
#20431,#20432,#20433,#20434,#20435,#20436),.UNSPECIFIED.,.F.,.F.,(4,1,1,
1,1,1,1,1,4),(28.2743338823081,28.6288240501929,29.6152849435979,30.6017458370029,
31.5882067304079,32.5746676238129,33.5611285172179,34.5475894106229,34.5575191894877),
 .UNSPECIFIED.);
#594=B_SPLINE_CURVE_WITH_KNOTS('',3,(#20437,#20438,#20439,#20440,#20441,
#20442,#20443,#20444,#20445,#20446),.UNSPECIFIED.,.F.,.F.,(4,1,1,1,1,1,
1,4),(28.2743338823081,29.1953135280469,30.1817744214519,31.1682353148569,
32.1546962082619,33.1411571016669,34.1276179950719,34.5575191894877),
 .UNSPECIFIED.);
#595=B_SPLINE_CURVE_WITH_KNOTS('',3,(#20451,#20452,#20453,#20454,#20455,
#20456,#20457,#20458,#20459,#20460),.UNSPECIFIED.,.F.,.F.,(4,1,1,1,1,1,
1,4),(21.9911485751285,22.7100586897628,23.6965195831678,24.6829804765728,
25.6694413699778,26.6559022633828,27.6423631567879,28.2743338823081),
 .UNSPECIFIED.);
#596=B_SPLINE_CURVE_WITH_KNOTS('',3,(#20461,#20462,#20463,#20464,#20465,
#20466,#20467,#20468,#20469,#20470,#20471),.UNSPECIFIED.,.F.,.F.,(4,1,1,
1,1,1,1,1,4),(21.9911485751285,22.2900872742119,23.2765481676169,24.2630090610219,
25.2494699544269,26.2359308478319,27.2223917412369,28.2088526346419,28.2743338823081),
 .UNSPECIFIED.);
#597=B_SPLINE_CURVE_WITH_KNOTS('',3,(#20477,#20478,#20479,#20480,#20481),
 .UNSPECIFIED.,.F.,.F.,(4,1,4),(14.3984001269718,15.3848610203768,15.7079632679489),
 .UNSPECIFIED.);
#598=B_SPLINE_CURVE_WITH_KNOTS('',3,(#20484,#20485,#20486,#20487,#20488),
 .UNSPECIFIED.,.F.,.F.,(4,1,4),(13.8759337553363,14.8183715425228,15.707963267949),
 .UNSPECIFIED.);
#599=B_SPLINE_CURVE_WITH_KNOTS('',3,(#20494,#20495,#20496,#20497,#20498,
#20499,#20500,#20501),.UNSPECIFIED.,.F.,.F.,(4,1,1,1,1,4),(59.6902604182061,
60.1955726391529,61.1820335325579,62.1684944259629,63.1549553193679,64.1414162127729),
 .UNSPECIFIED.);
#600=B_SPLINE_CURVE_WITH_KNOTS('',3,(#20504,#20505,#20506,#20507,#20508,
#20509,#20510,#20511,#20512),.UNSPECIFIED.,.F.,.F.,(4,1,1,1,1,1,4),(59.6902604182061,
59.775601223602,60.762062117007,61.748523010412,62.734983903817,63.721444797222,
64.6638825844085),.UNSPECIFIED.);
#601=B_SPLINE_CURVE_WITH_KNOTS('',3,(#20517,#20518,#20519,#20520,#20521,
#20522,#20523,#20524,#20525,#20526),.UNSPECIFIED.,.F.,.F.,(4,1,1,1,1,1,
1,4),(53.4070751110265,54.2768072787229,55.2632681721279,56.2497290655329,
57.2361899589379,58.2226508523429,59.2091117457479,59.6902604182061),
 .UNSPECIFIED.);
#602=B_SPLINE_CURVE_WITH_KNOTS('',3,(#20527,#20528,#20529,#20530,#20531,
#20532,#20533,#20534,#20535,#20536),.UNSPECIFIED.,.F.,.F.,(4,1,1,1,1,1,
1,4),(53.4070751110265,53.856835863172,54.843296756577,55.829757649982,
56.816218543387,57.802679436792,58.789140330197,59.6902604182061),
 .UNSPECIFIED.);
#603=B_SPLINE_CURVE_WITH_KNOTS('',3,(#20541,#20542,#20543,#20544,#20545,
#20546,#20547,#20548,#20549,#20550,#20551),.UNSPECIFIED.,.F.,.F.,(4,1,1,
1,1,1,1,1,4),(47.1238898038469,47.3715810248879,48.3580419182929,49.3445028116979,
50.3309637051029,51.3174245985079,52.3038854919129,53.2903463853179,53.4070751110265),
 .UNSPECIFIED.);
#604=B_SPLINE_CURVE_WITH_KNOTS('',3,(#20552,#20553,#20554,#20555,#20556,
#20557,#20558,#20559,#20560,#20561),.UNSPECIFIED.,.F.,.F.,(4,1,1,1,1,1,
1,4),(47.1238898038469,47.9380705027419,48.9245313961469,49.9109922895519,
50.8974531829569,51.8839140763619,52.8703749697669,53.4070751110265),
 .UNSPECIFIED.);
#605=B_SPLINE_CURVE_WITH_KNOTS('',3,(#20566,#20567,#20568,#20569,#20570,
#20571,#20572,#20573,#20574,#20575),.UNSPECIFIED.,.F.,.F.,(4,1,1,1,1,1,
1,4),(40.8407044966673,41.4528156644579,42.4392765578629,43.4257374512679,
44.4121983446729,45.3986592380779,46.3851201314829,47.1238898038469),
 .UNSPECIFIED.);
#606=B_SPLINE_CURVE_WITH_KNOTS('',3,(#20576,#20577,#20578,#20579,#20580,
#20581,#20582,#20583,#20584,#20585,#20586),.UNSPECIFIED.,.F.,.F.,(4,1,1,
1,1,1,1,1,4),(40.8407044966673,41.0328442489069,42.0193051423119,43.0057660357169,
43.9922269291219,44.9786878225269,45.9651487159319,46.9516096093369,47.1238898038469),
 .UNSPECIFIED.);
#607=B_SPLINE_CURVE_WITH_KNOTS('',3,(#20591,#20592,#20593,#20594,#20595,
#20596,#20597,#20598,#20599,#20600),.UNSPECIFIED.,.F.,.F.,(4,1,1,1,1,1,
1,4),(34.5575191894877,35.5340503040279,36.5205111974329,37.5069720908379,
38.4934329842429,39.4798938776479,40.4663547710529,40.8407044966673),
 .UNSPECIFIED.);
#608=B_SPLINE_CURVE_WITH_KNOTS('',3,(#20601,#20602,#20603,#20604,#20605,
#20606,#20607,#20608,#20609,#20610),.UNSPECIFIED.,.F.,.F.,(4,1,1,1,1,1,
1,4),(34.5575191894877,35.1140788884769,36.1005397818819,37.0870006752869,
38.0734615686919,39.0599224620969,40.0463833555019,40.8407044966673),
 .UNSPECIFIED.);
#609=B_SPLINE_CURVE_WITH_KNOTS('',3,(#20615,#20616,#20617,#20618,#20619,
#20620,#20621,#20622,#20623,#20624,#20625),.UNSPECIFIED.,.F.,.F.,(4,1,1,
1,1,1,1,1,4),(28.2743338823081,28.6288240501928,29.6152849435978,30.6017458370028,
31.5882067304078,32.5746676238129,33.5611285172179,34.5475894106229,34.5575191894877),
 .UNSPECIFIED.);
#610=B_SPLINE_CURVE_WITH_KNOTS('',3,(#20626,#20627,#20628,#20629,#20630,
#20631,#20632,#20633,#20634,#20635),.UNSPECIFIED.,.F.,.F.,(4,1,1,1,1,1,
1,4),(28.2743338823081,29.1953135280469,30.1817744214519,31.1682353148569,
32.1546962082619,33.1411571016669,34.1276179950719,34.5575191894877),
 .UNSPECIFIED.);
#611=B_SPLINE_CURVE_WITH_KNOTS('',3,(#20640,#20641,#20642,#20643,#20644,
#20645,#20646,#20647,#20648,#20649),.UNSPECIFIED.,.F.,.F.,(4,1,1,1,1,1,
1,4),(21.9911485751285,22.7100586897628,23.6965195831678,24.6829804765728,
25.6694413699778,26.6559022633828,27.6423631567878,28.2743338823081),
 .UNSPECIFIED.);
#612=B_SPLINE_CURVE_WITH_KNOTS('',3,(#20650,#20651,#20652,#20653,#20654,
#20655,#20656,#20657,#20658,#20659,#20660),.UNSPECIFIED.,.F.,.F.,(4,1,1,
1,1,1,1,1,4),(21.9911485751285,22.2900872742119,23.2765481676169,24.2630090610219,
25.2494699544269,26.2359308478319,27.2223917412369,28.2088526346419,28.2743338823081),
 .UNSPECIFIED.);
#613=B_SPLINE_CURVE_WITH_KNOTS('',3,(#20666,#20667,#20668,#20669,#20670),
 .UNSPECIFIED.,.F.,.F.,(4,1,4),(14.3984001269718,15.3848610203768,15.7079632679489),
 .UNSPECIFIED.);
#614=B_SPLINE_CURVE_WITH_KNOTS('',3,(#20673,#20674,#20675,#20676,#20677),
 .UNSPECIFIED.,.F.,.F.,(4,1,4),(13.8759337553362,14.8183715425228,15.707963267949),
 .UNSPECIFIED.);
#615=B_SPLINE_CURVE_WITH_KNOTS('',3,(#20679,#20680,#20681,#20682,#20683,
#20684,#20685,#20686,#20687,#20688,#20689),.UNSPECIFIED.,.F.,.F.,(4,1,1,
1,1,1,1,1,4),(15.707963267949,15.8048324359278,16.7912933293328,17.7777542227378,
18.7642151161428,19.7506760095478,20.7371369029528,21.7235977963578,21.9911485751285),
 .UNSPECIFIED.);
#616=B_SPLINE_CURVE_WITH_KNOTS('',3,(#20690,#20691,#20692,#20693,#20694,
#20695,#20696,#20697,#20698,#20699),.UNSPECIFIED.,.F.,.F.,(4,1,1,1,1,1,
1,4),(15.7079632679489,16.3713219137818,17.3577828071868,18.3442437005918,
19.3307045939968,20.3171654874019,21.3036263808069,21.9911485751285),
 .UNSPECIFIED.);
#617=B_SPLINE_CURVE_WITH_KNOTS('',3,(#20924,#20925,#20926,#20927,#20928,
#20929,#20930,#20931,#20932,#20933,#20934,#20935,#20936,#20937,#20938,#20939,
#20940,#20941,#20942,#20943,#20944,#20945,#20946,#20947,#20948,#20949,#20950,
#20951,#20952,#20953,#20954,#20955,#20956,#20957,#20958,#20959,#20960,#20961,
#20962,#20963,#20964,#20965,#20966,#20967,#20968,#20969,#20970,#20971,#20972,
#20973,#20974,#20975,#20976,#20977,#20978,#20979,#20980,#20981,#20982,#20983,
#20984,#20985,#20986,#20987,#20988,#20989,#20990,#20991,#20992,#20993,#20994,
#20995,#20996,#20997,#20998,#20999,#21000,#21001,#21002,#21003,#21004,#21005,
#21006,#21007,#21008,#21009,#21010,#21011,#21012,#21013,#21014,#21015,#21016,
#21017,#21018,#21019,#21020),.UNSPECIFIED.,.F.,.F.,(4,3,3,3,3,3,3,3,3,3,
3,3,3,3,3,3,3,3,3,3,3,3,3,3,3,3,3,3,3,3,3,3,4),(0.,0.0368039760561726,0.0744333368184212,
0.113993729911609,0.148609073868149,0.155428926386467,0.160415234743925,
0.197652231831378,0.234804645306633,0.271449203389433,0.301316022933056,
0.308903620706599,0.314301810562592,0.350380482429235,0.385744360315095,
0.390916481563925,0.427339708572203,0.447829010654916,0.457282929707203,
0.462717601073039,0.49927396867586,0.535072006502099,0.570520288994985,
0.593601320607563,0.601390745293023,0.606406519246091,0.641366357839995,
0.669816903853899,0.683592867357584,0.691680491796103,0.725189672020684,
0.755168541895609,0.770777738583641),.UNSPECIFIED.);
#618=B_SPLINE_CURVE_WITH_KNOTS('',3,(#21021,#21022,#21023,#21024,#21025,
#21026,#21027,#21028,#21029,#21030,#21031,#21032,#21033,#21034,#21035,#21036,
#21037,#21038,#21039,#21040,#21041,#21042,#21043,#21044,#21045,#21046,#21047,
#21048,#21049,#21050,#21051,#21052,#21053,#21054,#21055,#21056,#21057,#21058,
#21059,#21060,#21061,#21062,#21063,#21064,#21065,#21066,#21067,#21068,#21069,
#21070,#21071,#21072,#21073,#21074,#21075,#21076,#21077,#21078,#21079,#21080,
#21081,#21082,#21083,#21084,#21085,#21086,#21087,#21088,#21089,#21090,#21091,
#21092,#21093,#21094,#21095,#21096,#21097,#21098,#21099,#21100,#21101,#21102,
#21103,#21104,#21105,#21106,#21107,#21108,#21109,#21110,#21111,#21112,#21113,
#21114),.UNSPECIFIED.,.F.,.F.,(4,3,3,3,3,3,3,3,3,3,3,3,3,3,3,3,3,3,3,3,
3,3,3,3,3,3,3,3,3,3,3,4),(0.,0.032722467477059,0.0662804545367435,0.10053688939052,
0.133256613707586,0.138568806761047,0.143645866999149,0.178633816756561,
0.214080697136686,0.251134193834276,0.278924316357469,0.285558989874725,
0.321777082201843,0.35776277380543,0.362294683927046,0.397656589907163,
0.419708610865643,0.427245995316486,0.432639299360784,0.468078725795143,
0.504737384281388,0.54174098163239,0.567834474583697,0.579481956142016,
0.584481809181592,0.622063983748247,0.654170219121896,0.668576993434055,
0.678363333947687,0.716158233455664,0.750488925242844,0.768398079192646),
 .UNSPECIFIED.);
#619=B_SPLINE_CURVE_WITH_KNOTS('',3,(#21115,#21116,#21117,#21118,#21119,
#21120,#21121,#21122,#21123,#21124,#21125,#21126,#21127,#21128,#21129,#21130,
#21131,#21132,#21133,#21134,#21135,#21136,#21137,#21138,#21139),
 .UNSPECIFIED.,.F.,.F.,(4,3,3,3,3,3,3,3,4),(-10.1321597128207,-9.86460893405003,
-8.87814804064502,-7.89168714724003,-6.90522625383502,-5.91876536043002,
-4.93230446702502,-3.94584357362001,-3.84897440564115),.UNSPECIFIED.);
#620=B_SPLINE_CURVE_WITH_KNOTS('',3,(#21364,#21365,#21366,#21367,#21368,
#21369,#21370,#21371,#21372,#21373,#21374,#21375,#21376,#21377,#21378,#21379,
#21380,#21381,#21382,#21383,#21384,#21385,#21386,#21387,#21388,#21389,#21390,
#21391,#21392,#21393,#21394,#21395,#21396,#21397,#21398,#21399,#21400,#21401,
#21402,#21403,#21404,#21405,#21406,#21407,#21408,#21409,#21410,#21411,#21412,
#21413,#21414,#21415,#21416,#21417,#21418,#21419,#21420,#21421,#21422,#21423,
#21424,#21425,#21426,#21427,#21428,#21429,#21430,#21431,#21432,#21433,#21434,
#21435,#21436,#21437,#21438,#21439,#21440,#21441,#21442,#21443,#21444,#21445,
#21446,#21447,#21448,#21449,#21450,#21451,#21452,#21453,#21454,#21455,#21456,
#21457),.UNSPECIFIED.,.F.,.F.,(4,3,3,3,3,3,3,3,3,3,3,3,3,3,3,3,3,3,3,3,
3,3,3,3,3,3,3,3,3,3,3,4),(0.,0.0327225799773267,0.0662806658545984,0.100537171029244,
0.133256860141472,0.138569969050608,0.143646002487887,0.178634022059388,
0.214080931165366,0.251134369355791,0.27892444799861,0.285558993885552,
0.321777092476967,0.357762747477908,0.362294683927068,0.397656542631737,
0.419708566544936,0.427246605750548,0.432639210952107,0.468078568034648,
0.504737197455354,0.541740788532467,0.567834305621274,0.579481260120421,
0.584480754431237,0.622062913075079,0.654169416117039,0.668576403279121,
0.678363443657298,0.716158340709877,0.750488925242921,0.768398079192729),
 .UNSPECIFIED.);
#621=B_SPLINE_CURVE_WITH_KNOTS('',3,(#21458,#21459,#21460,#21461,#21462,
#21463,#21464,#21465,#21466,#21467,#21468,#21469,#21470,#21471,#21472,#21473,
#21474,#21475,#21476,#21477,#21478,#21479,#21480,#21481,#21482),
 .UNSPECIFIED.,.F.,.F.,(4,3,3,3,3,3,3,3,4),(7.59274844815668,7.89168714724002,
8.87814804064503,9.86460893405003,10.851069827455,11.83753072086,12.823991614265,
13.81045250767,13.8759337553363),.UNSPECIFIED.);
#622=B_SPLINE_CURVE_WITH_KNOTS('',3,(#21483,#21484,#21485,#21486,#21487,
#21488,#21489,#21490,#21491,#21492,#21493,#21494,#21495,#21496,#21497,#21498,
#21499,#21500,#21501,#21502,#21503,#21504,#21505,#21506,#21507,#21508,#21509,
#21510,#21511,#21512,#21513,#21514,#21515,#21516,#21517,#21518,#21519,#21520,
#21521,#21522,#21523,#21524,#21525,#21526,#21527,#21528,#21529,#21530,#21531,
#21532,#21533,#21534,#21535,#21536,#21537,#21538,#21539,#21540,#21541,#21542,
#21543,#21544,#21545,#21546,#21547,#21548,#21549,#21550,#21551,#21552,#21553,
#21554,#21555,#21556,#21557,#21558,#21559,#21560,#21561,#21562,#21563,#21564,
#21565,#21566,#21567,#21568,#21569,#21570,#21571,#21572,#21573,#21574,#21575,
#21576,#21577,#21578,#21579),.UNSPECIFIED.,.F.,.F.,(4,3,3,3,3,3,3,3,3,3,
3,3,3,3,3,3,3,3,3,3,3,3,3,3,3,3,3,3,3,3,3,3,4),(0.,0.0368040733914109,0.0744334923513577,
0.113993866002931,0.148609192948057,0.155429662167008,0.160415950914505,
0.197652959912295,0.23480534579311,0.271449857509325,0.301316513522979,
0.308905291482282,0.314302114409216,0.350380752512021,0.385744595636286,
0.390916481563942,0.427339707606562,0.447829009749629,0.457282909273663,
0.462717595625807,0.499273963909537,0.53507200404104,0.57052027575377,0.593601309021504,
0.60139070143526,0.60640643038342,0.641366263001721,0.669816832725203,0.683592798284754,
0.691680481858046,0.725189622506651,0.755168541895646,0.770777738583679),
 .UNSPECIFIED.);
#623=B_SPLINE_CURVE_WITH_KNOTS('',3,(#21589,#21590,#21591,#21592,#21593,
#21594,#21595,#21596,#21597,#21598,#21599,#21600,#21601,#21602,#21603,#21604,
#21605,#21606,#21607,#21608,#21609,#21610,#21611,#21612,#21613,#21614,#21615,
#21616,#21617,#21618,#21619,#21620,#21621,#21622,#21623,#21624,#21625,#21626,
#21627,#21628,#21629,#21630,#21631,#21632,#21633,#21634,#21635,#21636,#21637,
#21638,#21639,#21640,#21641,#21642,#21643,#21644,#21645,#21646,#21647,#21648,
#21649,#21650,#21651,#21652,#21653,#21654,#21655,#21656,#21657,#21658,#21659,
#21660,#21661,#21662,#21663,#21664,#21665,#21666,#21667,#21668,#21669,#21670,
#21671,#21672,#21673,#21674,#21675,#21676,#21677,#21678,#21679,#21680,#21681,
#21682),.UNSPECIFIED.,.F.,.F.,(4,3,3,3,3,3,3,3,3,3,3,3,3,3,3,3,3,3,3,3,
3,3,3,3,3,3,3,3,3,3,3,4),(0.,0.0327224959120641,0.0662805079475318,0.100536960576692,
0.133256675995489,0.138569100515552,0.143645901206212,0.1786338686101,0.214080756253453,
0.251134238171856,0.278924349610658,0.285558990870915,0.321777084786821,
0.35776276714434,0.362294683927063,0.39765657796237,0.419708599667403,0.427246149485785,
0.432639276975905,0.468078685886249,0.504737337027106,0.541740932792406,
0.567834431848717,0.579481780097231,0.584481542244862,0.622063712786212,
0.654170015900382,0.6685768440841,0.678363361689231,0.716158260579035,0.750488925242892,
0.768398079192696),.UNSPECIFIED.);
#624=B_SPLINE_CURVE_WITH_KNOTS('',3,(#21683,#21684,#21685,#21686,#21687,
#21688,#21689,#21690,#21691,#21692,#21693,#21694,#21695,#21696,#21697,#21698,
#21699,#21700,#21701,#21702,#21703,#21704,#21705,#21706,#21707,#21708,#21709,
#21710,#21711,#21712,#21713,#21714,#21715,#21716,#21717,#21718,#21719,#21720,
#21721,#21722,#21723,#21724,#21725,#21726,#21727,#21728,#21729,#21730,#21731,
#21732,#21733,#21734,#21735,#21736,#21737,#21738,#21739,#21740,#21741,#21742,
#21743,#21744,#21745,#21746,#21747,#21748,#21749,#21750,#21751,#21752,#21753,
#21754,#21755,#21756,#21757,#21758,#21759,#21760,#21761,#21762,#21763,#21764,
#21765,#21766,#21767,#21768,#21769,#21770,#21771,#21772,#21773,#21774,#21775,
#21776,#21777,#21778,#21779),.UNSPECIFIED.,.F.,.F.,(4,3,3,3,3,3,3,3,3,3,
3,3,3,3,3,3,3,3,3,3,3,3,3,3,3,3,3,3,3,3,3,3,4),(0.,0.0368039914157241,0.0744333613634087,
0.113993751388472,0.148609092660403,0.155429042492168,0.160415347695229,
0.197652346662473,0.234804755786334,0.271449306551343,0.301316100304487,
0.308903884150417,0.314301858425386,0.350380524963378,0.385744397367857,
0.390916481563918,0.427339708424226,0.447829010516186,0.457282926489124,
0.462717600214839,0.499273967924932,0.53507200611566,0.570520286913965,
0.593601318786667,0.601390738323114,0.606406505217338,0.64136634286951,
0.669816892626028,0.683592856456032,0.691680490247784,0.725189664234744,
0.75516854189558,0.770777738583609),.UNSPECIFIED.);
#625=B_SPLINE_CURVE_WITH_KNOTS('',3,(#21780,#21781,#21782,#21783,#21784,
#21785,#21786,#21787,#21788,#21789,#21790,#21791,#21792,#21793,#21794,#21795,
#21796,#21797,#21798,#21799,#21800,#21801,#21802,#21803,#21804,#21805,#21806,
#21807,#21808,#21809,#21810,#21811,#21812,#21813,#21814,#21815,#21816,#21817,
#21818,#21819,#21820,#21821,#21822,#21823,#21824,#21825,#21826,#21827,#21828,
#21829,#21830,#21831,#21832,#21833,#21834,#21835,#21836,#21837,#21838,#21839,
#21840,#21841,#21842,#21843,#21844,#21845,#21846,#21847,#21848,#21849,#21850,
#21851,#21852,#21853,#21854,#21855,#21856,#21857,#21858,#21859,#21860,#21861,
#21862,#21863,#21864,#21865,#21866,#21867,#21868,#21869,#21870,#21871,#21872,
#21873),.UNSPECIFIED.,.F.,.F.,(4,3,3,3,3,3,3,3,3,3,3,3,3,3,3,3,3,3,3,3,
3,3,3,3,3,3,3,3,3,3,3,4),(0.,0.0327225294770781,0.0662805709960721,0.100537044605592,
0.133256749520777,0.138569447222746,0.143645941610917,0.17863392984422,
0.214080826059521,0.251134290526409,0.278924388876575,0.285558992053491,
0.321777087844177,0.357762759284444,0.362294683927074,0.397656563857957,
0.419708586444518,0.427246331524387,0.432639250564409,0.468078638783316,
0.50473728125208,0.541740875145429,0.567834381407617,0.579481572313244,
0.584481227357561,0.622063393148413,0.654169776172043,0.668576667903374,
0.678363394448717,0.71615829260595,0.750488925242933,0.768398079192735),
 .UNSPECIFIED.);
#626=B_SPLINE_CURVE_WITH_KNOTS('',3,(#21874,#21875,#21876,#21877,#21878,
#21879,#21880,#21881,#21882,#21883,#21884,#21885,#21886,#21887,#21888,#21889,
#21890,#21891,#21892,#21893,#21894,#21895,#21896,#21897,#21898,#21899,#21900,
#21901,#21902,#21903,#21904,#21905,#21906,#21907,#21908,#21909,#21910,#21911,
#21912,#21913,#21914,#21915,#21916,#21917,#21918,#21919,#21920,#21921,#21922,
#21923,#21924,#21925,#21926,#21927,#21928,#21929,#21930,#21931,#21932,#21933,
#21934,#21935,#21936,#21937,#21938,#21939,#21940,#21941,#21942,#21943,#21944,
#21945,#21946,#21947,#21948,#21949,#21950,#21951,#21952,#21953,#21954,#21955,
#21956,#21957,#21958,#21959,#21960,#21961,#21962,#21963,#21964,#21965,#21966,
#21967,#21968,#21969,#21970),.UNSPECIFIED.,.F.,.F.,(4,3,3,3,3,3,3,3,3,3,
3,3,3,3,3,3,3,3,3,3,3,3,3,3,3,3,3,3,3,3,3,3,4),(0.,0.0368040169038835,0.0744334020924358,
0.11399378702637,0.148609123843563,0.155429235171562,0.160415535189551,
0.197652537277058,0.234804939176668,0.271449477805488,0.301316228745094,
0.308904321525207,0.31430193792665,0.350380595626898,0.385744458930709,
0.390916481563911,0.427339708170469,0.447829010278287,0.45728292112946,
0.462717598788197,0.499273966676618,0.535072005472898,0.570520283450759,
0.593601315756361,0.601390726866048,0.606406481970154,0.641366318060403,
0.669816874019195,0.683592838382448,0.691680487645043,0.725189651274617,
0.75516854189557,0.770777738583599),.UNSPECIFIED.);
#627=B_SPLINE_CURVE_WITH_KNOTS('',3,(#21971,#21972,#21973,#21974,#21975,
#21976,#21977,#21978,#21979,#21980,#21981,#21982,#21983,#21984,#21985,#21986,
#21987,#21988,#21989,#21990,#21991,#21992,#21993,#21994,#21995,#21996,#21997,
#21998,#21999,#22000,#22001,#22002,#22003,#22004,#22005,#22006,#22007,#22008,
#22009,#22010,#22011,#22012,#22013,#22014,#22015,#22016,#22017,#22018,#22019,
#22020,#22021,#22022,#22023,#22024,#22025,#22026,#22027,#22028,#22029,#22030,
#22031,#22032,#22033,#22034,#22035,#22036,#22037,#22038,#22039,#22040,#22041,
#22042,#22043,#22044,#22045,#22046,#22047,#22048,#22049,#22050,#22051,#22052,
#22053,#22054,#22055,#22056,#22057,#22058,#22059,#22060,#22061,#22062,#22063,
#22064),.UNSPECIFIED.,.F.,.F.,(4,3,3,3,3,3,3,3,3,3,3,3,3,3,3,3,3,3,3,3,
3,3,3,3,3,3,3,3,3,3,3,4),(0.,0.0327224441775746,0.0662804107708102,0.100536831058394,
0.133256562666979,0.138568566128973,0.143645838996043,0.178633774293771,
0.214080648720454,0.251134157522108,0.278924289123348,0.285558989031475,
0.321777080052277,0.357762779229756,0.362294683927068,0.397656599693718,
0.419708620040541,0.427245869011975,0.432639317722629,0.468078758515067,
0.504737423019667,0.541741021670041,0.567834509616647,0.5794821004587,0.584482028048437,
0.622064205916635,0.6541703857482,0.668577115889702,0.678363311229139,0.716158211242659,
0.750488925242892,0.768398079192695),.UNSPECIFIED.);
#628=B_SPLINE_CURVE_WITH_KNOTS('',3,(#22065,#22066,#22067,#22068,#22069,
#22070,#22071,#22072,#22073,#22074,#22075,#22076,#22077,#22078,#22079,#22080,
#22081,#22082,#22083,#22084,#22085,#22086,#22087,#22088,#22089,#22090,#22091,
#22092,#22093,#22094,#22095,#22096,#22097,#22098,#22099,#22100,#22101,#22102,
#22103,#22104,#22105,#22106,#22107,#22108,#22109,#22110,#22111,#22112,#22113,
#22114,#22115,#22116,#22117,#22118,#22119,#22120,#22121,#22122,#22123,#22124,
#22125,#22126,#22127,#22128,#22129,#22130,#22131,#22132,#22133,#22134,#22135,
#22136,#22137,#22138,#22139,#22140,#22141,#22142,#22143,#22144,#22145,#22146,
#22147,#22148,#22149,#22150,#22151,#22152,#22153,#22154,#22155,#22156,#22157,
#22158,#22159,#22160,#22161),.UNSPECIFIED.,.F.,.F.,(4,3,3,3,3,3,3,3,3,3,
3,3,3,3,3,3,3,3,3,3,3,3,3,3,3,3,3,3,3,3,3,3,4),(0.,0.036804046830165,0.0744334499110545,
0.113993828867664,0.148609160454698,0.155429461366191,0.160415755364031,
0.197652761113477,0.234805154528782,0.271449678901402,0.301316379567035,
0.30890483519103,0.314302031357973,0.350380678677425,0.385744531292533,
0.390916481563933,0.427339707871941,0.447829009998422,0.457282914861488,
0.462717597114684,0.499273965212302,0.535072004716797,0.570520279377824,
0.59360131219255,0.601390713399489,0.606406454642536,0.641366288894707,
0.669816852144937,0.683592817141769,0.691680484574319,0.72518963603372,
0.75516854189563,0.77077773858366),.UNSPECIFIED.);
#629=B_SPLINE_CURVE_WITH_KNOTS('',3,(#22163,#22164,#22165,#22166,#22167,
#22168,#22169,#22170,#22171,#22172,#22173),.UNSPECIFIED.,.F.,.F.,(4,1,1,
1,1,1,1,1,4),(15.707963267949,15.8048324359278,16.7912933293328,17.7777542227378,
18.7642151161428,19.7506760095478,20.7371369029528,21.7235977963578,21.9911485751285),
 .UNSPECIFIED.);
#630=B_SPLINE_CURVE_WITH_KNOTS('',3,(#22174,#22175,#22176,#22177,#22178,
#22179,#22180,#22181,#22182,#22183),.UNSPECIFIED.,.F.,.F.,(4,1,1,1,1,1,
1,4),(15.7079632679489,16.3713219137818,17.3577828071869,18.3442437005919,
19.3307045939969,20.3171654874019,21.3036263808069,21.9911485751285),
 .UNSPECIFIED.);
#631=B_SPLINE_CURVE_WITH_KNOTS('',3,(#22408,#22409,#22410,#22411,#22412,
#22413,#22414,#22415,#22416,#22417,#22418,#22419,#22420,#22421,#22422,#22423,
#22424,#22425,#22426,#22427,#22428,#22429,#22430,#22431,#22432,#22433,#22434,
#22435,#22436,#22437,#22438,#22439,#22440,#22441,#22442,#22443,#22444,#22445,
#22446,#22447,#22448,#22449,#22450,#22451,#22452,#22453,#22454,#22455,#22456,
#22457,#22458,#22459,#22460,#22461,#22462,#22463,#22464,#22465,#22466,#22467,
#22468,#22469,#22470,#22471,#22472,#22473,#22474,#22475,#22476,#22477,#22478,
#22479,#22480,#22481,#22482,#22483,#22484,#22485,#22486,#22487,#22488,#22489,
#22490,#22491,#22492,#22493,#22494,#22495,#22496,#22497,#22498,#22499,#22500,
#22501,#22502,#22503,#22504),.UNSPECIFIED.,.F.,.F.,(4,3,3,3,3,3,3,3,3,3,
3,3,3,3,3,3,3,3,3,3,3,3,3,3,3,3,3,3,3,3,3,3,4),(0.,0.0368040006584821,0.0744333761311954,
0.113993764310286,0.14860910396699,0.155429112383965,0.160415415803185,
0.19765241590165,0.234804822404722,0.27144936877189,0.301316146969897,0.308904043046986,
0.314301887301155,0.350380550636825,0.385744419741531,0.39091648156392,
0.427339708332513,0.447829010430206,0.45728292453119,0.462717599696291,
0.499273967471206,0.535072005882051,0.570520285658179,0.593601317687859,
0.601390734201157,0.60640649698701,0.641366334082055,0.669816886035445,
0.683592850009941,0.691680489272535,0.725189659504915,0.755168541895614,
0.770777738583643),.UNSPECIFIED.);
#632=B_SPLINE_CURVE_WITH_KNOTS('',3,(#22505,#22506,#22507,#22508,#22509,
#22510,#22511,#22512,#22513,#22514,#22515,#22516,#22517,#22518,#22519,#22520,
#22521,#22522,#22523,#22524,#22525,#22526,#22527,#22528,#22529),
 .UNSPECIFIED.,.F.,.F.,(4,3,3,3,3,3,3,3,4),(-10.1321597128207,-9.86460893405003,
-8.87814804064502,-7.89168714724002,-6.90522625383502,-5.91876536043002,
-4.93230446702501,-3.94584357362001,-3.84897440564114),.UNSPECIFIED.);
#633=B_SPLINE_CURVE_WITH_KNOTS('',3,(#22754,#22755,#22756,#22757,#22758,
#22759,#22760,#22761,#22762,#22763,#22764,#22765,#22766,#22767,#22768,#22769,
#22770,#22771,#22772,#22773,#22774,#22775,#22776,#22777,#22778,#22779,#22780,
#22781,#22782,#22783,#22784,#22785,#22786,#22787,#22788,#22789,#22790,#22791,
#22792,#22793,#22794,#22795,#22796,#22797,#22798,#22799,#22800,#22801,#22802,
#22803,#22804,#22805,#22806,#22807,#22808,#22809,#22810,#22811,#22812,#22813,
#22814,#22815,#22816,#22817,#22818,#22819,#22820,#22821,#22822,#22823,#22824,
#22825,#22826,#22827,#22828,#22829,#22830,#22831,#22832,#22833,#22834,#22835,
#22836,#22837,#22838,#22839,#22840,#22841,#22842,#22843,#22844,#22845,#22846,
#22847),.UNSPECIFIED.,.F.,.F.,(4,3,3,3,3,3,3,3,3,3,3,3,3,3,3,3,3,3,3,3,
3,3,3,3,3,3,3,3,3,3,3,4),(0.,0.0327224852298601,0.0662804878799529,0.100536933829056,
0.133256652591307,0.138568990289855,0.143645888367285,0.178633849142766,
0.214080734056413,0.251134221524075,0.278924337124821,0.285558990484342,
0.321777083808023,0.357762769641534,0.362294683927059,0.397656582449134,
0.419708603873742,0.427246091593913,0.432639285230977,0.468078700718258,
0.504737354615871,0.541740950976496,0.567834447759792,0.579481845655055,
0.584481641657808,0.62206381370368,0.654170091588477,0.668576899729838,
0.678363351333556,0.716158250454694,0.750488925242868,0.768398079192674),
 .UNSPECIFIED.);
#634=B_SPLINE_CURVE_WITH_KNOTS('',3,(#22848,#22849,#22850,#22851,#22852,
#22853,#22854,#22855,#22856,#22857,#22858,#22859,#22860,#22861,#22862,#22863,
#22864,#22865,#22866,#22867,#22868,#22869,#22870,#22871,#22872),
 .UNSPECIFIED.,.F.,.F.,(4,3,3,3,3,3,3,3,4),(7.59274844815667,7.89168714724002,
8.87814804064502,9.86460893405003,10.851069827455,11.83753072086,12.823991614265,
13.81045250767,13.8759337553363),.UNSPECIFIED.);
#635=B_SPLINE_CURVE_WITH_KNOTS('',3,(#22874,#22875,#22876,#22877,#22878,
#22879,#22880,#22881,#22882,#22883,#22884),.UNSPECIFIED.,.F.,.F.,(4,1,1,
1,1,1,1,1,4),(15.707963267949,15.8048324359278,16.7912933293328,17.7777542227378,
18.7642151161428,19.7506760095478,20.7371369029528,21.7235977963578,21.9911485751285),
 .UNSPECIFIED.);
#636=B_SPLINE_CURVE_WITH_KNOTS('',3,(#22885,#22886,#22887,#22888,#22889,
#22890,#22891,#22892,#22893,#22894),.UNSPECIFIED.,.F.,.F.,(4,1,1,1,1,1,
1,4),(15.7079632679489,16.3713219137818,17.3577828071868,18.3442437005918,
19.3307045939968,20.3171654874019,21.3036263808069,21.9911485751285),
 .UNSPECIFIED.);
#637=B_SPLINE_CURVE_WITH_KNOTS('',3,(#23119,#23120,#23121,#23122,#23123,
#23124,#23125,#23126,#23127,#23128,#23129,#23130,#23131,#23132,#23133,#23134,
#23135,#23136,#23137,#23138,#23139,#23140,#23141,#23142,#23143,#23144,#23145,
#23146,#23147,#23148,#23149,#23150,#23151,#23152,#23153,#23154,#23155,#23156,
#23157,#23158,#23159,#23160,#23161,#23162,#23163,#23164,#23165,#23166,#23167,
#23168,#23169,#23170,#23171,#23172,#23173,#23174,#23175,#23176,#23177,#23178,
#23179,#23180,#23181,#23182,#23183,#23184,#23185,#23186,#23187,#23188,#23189,
#23190,#23191,#23192,#23193,#23194,#23195,#23196,#23197,#23198,#23199,#23200,
#23201,#23202,#23203,#23204,#23205,#23206,#23207,#23208,#23209,#23210,#23211,
#23212,#23213,#23214,#23215),.UNSPECIFIED.,.F.,.F.,(4,3,3,3,3,3,3,3,3,3,
3,3,3,3,3,3,3,3,3,3,3,3,3,3,3,3,3,3,3,3,3,3,4),(0.,0.0368039558979425,0.074433304608195,
0.113993701727663,0.148609049207197,0.155428774052918,0.160415086629183,
0.19765208124705,0.234804500431717,0.271449068097489,0.301315921464101,
0.308903275242872,0.314301747825082,0.350380426672586,0.385744311753463,
0.390916481563936,0.427339708778546,0.447829010848363,0.457282933923372,
0.462717602197838,0.49927396966006,0.535072007005015,0.570520291726377,
0.593601322997532,0.601390754314479,0.606406537654944,0.641366377472567,
0.669816918578329,0.683592881655056,0.691680493901417,0.725189682307058,
0.755168541895614,0.770777738583641),.UNSPECIFIED.);
#638=B_SPLINE_CURVE_WITH_KNOTS('',3,(#23216,#23217,#23218,#23219,#23220,
#23221,#23222,#23223,#23224,#23225,#23226,#23227,#23228,#23229,#23230,#23231,
#23232,#23233,#23234,#23235,#23236,#23237,#23238,#23239,#23240),
 .UNSPECIFIED.,.F.,.F.,(4,3,3,3,3,3,3,3,4),(-10.1321597128207,-9.86460893405003,
-8.87814804064502,-7.89168714724003,-6.90522625383502,-5.91876536043002,
-4.93230446702502,-3.94584357362001,-3.84897440564115),.UNSPECIFIED.);
#639=B_SPLINE_CURVE_WITH_KNOTS('',3,(#23465,#23466,#23467,#23468,#23469,
#23470,#23471,#23472,#23473,#23474,#23475,#23476,#23477,#23478,#23479,#23480,
#23481,#23482,#23483,#23484,#23485,#23486,#23487,#23488,#23489,#23490,#23491,
#23492,#23493,#23494,#23495,#23496,#23497,#23498,#23499,#23500,#23501,#23502,
#23503,#23504,#23505,#23506,#23507,#23508,#23509,#23510,#23511,#23512,#23513,
#23514,#23515,#23516,#23517,#23518,#23519,#23520,#23521,#23522,#23523,#23524,
#23525,#23526,#23527,#23528,#23529,#23530,#23531,#23532,#23533,#23534,#23535,
#23536,#23537,#23538,#23539,#23540,#23541,#23542,#23543,#23544,#23545,#23546,
#23547,#23548,#23549,#23550,#23551,#23552,#23553,#23554,#23555,#23556,#23557,
#23558),.UNSPECIFIED.,.F.,.F.,(4,3,3,3,3,3,3,3,3,3,3,3,3,3,3,3,3,3,3,3,
3,3,3,3,3,3,3,3,3,3,3,4),(0.,0.0327225492804934,0.0662806081929849,0.100537094180834,
0.133256792899112,0.138569651942616,0.143645965484312,0.178633966005382,
0.214080867277344,0.251134321439773,0.278924412061594,0.285558992744241,
0.321777089637378,0.35776275463403,0.362294683927058,0.397656555534726,
0.419708578641487,0.427246439006672,0.432639234997264,0.468078611004923,
0.504737248356826,0.541740841146129,0.567834351658225,0.579481449773753,
0.584481041781399,0.622063204762494,0.654169634882595,0.668576564062872,
0.678363413635591,0.716158311359956,0.750488925242897,0.768398079192707),
 .UNSPECIFIED.);
#640=B_SPLINE_CURVE_WITH_KNOTS('',3,(#23559,#23560,#23561,#23562,#23563,
#23564,#23565,#23566,#23567,#23568,#23569,#23570,#23571,#23572,#23573,#23574,
#23575,#23576,#23577,#23578,#23579,#23580,#23581,#23582,#23583),
 .UNSPECIFIED.,.F.,.F.,(4,3,3,3,3,3,3,3,4),(7.59274844815668,7.89168714724002,
8.87814804064503,9.86460893405003,10.851069827455,11.83753072086,12.823991614265,
13.81045250767,13.8759337553363),.UNSPECIFIED.);
#641=B_SPLINE_CURVE_WITH_KNOTS('',3,(#23585,#23586,#23587,#23588,#23589,
#23590,#23591,#23592,#23593,#23594,#23595),.UNSPECIFIED.,.F.,.F.,(4,1,1,
1,1,1,1,1,4),(15.7079632679489,15.8048324359278,16.7912933293328,17.7777542227378,
18.7642151161428,19.7506760095478,20.7371369029528,21.7235977963578,21.9911485751285),
 .UNSPECIFIED.);
#642=B_SPLINE_CURVE_WITH_KNOTS('',3,(#23596,#23597,#23598,#23599,#23600,
#23601,#23602,#23603,#23604,#23605),.UNSPECIFIED.,.F.,.F.,(4,1,1,1,1,1,
1,4),(15.7079632679489,16.3713219137818,17.3577828071869,18.3442437005919,
19.3307045939969,20.3171654874019,21.3036263808069,21.9911485751285),
 .UNSPECIFIED.);
#643=B_SPLINE_CURVE_WITH_KNOTS('',3,(#23830,#23831,#23832,#23833,#23834,
#23835,#23836,#23837,#23838,#23839,#23840,#23841,#23842,#23843,#23844,#23845,
#23846,#23847,#23848,#23849,#23850,#23851,#23852,#23853,#23854,#23855,#23856,
#23857,#23858,#23859,#23860,#23861,#23862,#23863,#23864,#23865,#23866,#23867,
#23868,#23869,#23870,#23871,#23872,#23873,#23874,#23875,#23876,#23877,#23878,
#23879,#23880,#23881,#23882,#23883,#23884,#23885,#23886,#23887,#23888,#23889,
#23890,#23891,#23892,#23893,#23894,#23895,#23896,#23897,#23898,#23899,#23900,
#23901,#23902,#23903,#23904,#23905,#23906,#23907,#23908,#23909,#23910,#23911,
#23912,#23913,#23914,#23915,#23916,#23917,#23918,#23919,#23920,#23921,#23922,
#23923,#23924,#23925,#23926),.UNSPECIFIED.,.F.,.F.,(4,3,3,3,3,3,3,3,3,3,
3,3,3,3,3,3,3,3,3,3,3,3,3,3,3,3,3,3,3,3,3,3,4),(0.,0.0368040296983295,0.0744334225357169,
0.113993804914242,0.148609139495452,0.155429331856321,0.160415629309949,
0.19765263296232,0.234805031233744,0.271449563770314,0.301316293218716,
0.308904541097941,0.314301977856807,0.350380631124549,0.385744489860858,
0.39091648156392,0.427339708037647,0.447829010153769,0.457282918385807,
0.462717598065727,0.499273966044462,0.535072005142963,0.570520281705417,
0.593601314229191,0.601390721049491,0.606406470197016,0.641366305496701,
0.669816864596427,0.6835928292529,0.691680486306265,0.725189644734797,0.755168541895606,
0.770777738583634),.UNSPECIFIED.);
#644=B_SPLINE_CURVE_WITH_KNOTS('',3,(#23927,#23928,#23929,#23930,#23931,
#23932,#23933,#23934,#23935,#23936,#23937,#23938,#23939,#23940,#23941,#23942,
#23943,#23944,#23945,#23946,#23947,#23948,#23949,#23950,#23951),
 .UNSPECIFIED.,.F.,.F.,(4,3,3,3,3,3,3,3,4),(-10.1321597128207,-9.86460893405003,
-8.87814804064502,-7.89168714724002,-6.90522625383502,-5.91876536043002,
-4.93230446702502,-3.94584357362001,-3.84897440564114),.UNSPECIFIED.);
#645=B_SPLINE_CURVE_WITH_KNOTS('',3,(#24176,#24177,#24178,#24179,#24180,
#24181,#24182,#24183,#24184,#24185,#24186,#24187,#24188,#24189,#24190,#24191,
#24192,#24193,#24194,#24195,#24196,#24197,#24198,#24199,#24200,#24201,#24202,
#24203,#24204,#24205,#24206,#24207,#24208,#24209,#24210,#24211,#24212,#24213,
#24214,#24215,#24216,#24217,#24218,#24219,#24220,#24221,#24222,#24223,#24224,
#24225,#24226,#24227,#24228,#24229,#24230,#24231,#24232,#24233,#24234,#24235,
#24236,#24237,#24238,#24239,#24240,#24241,#24242,#24243,#24244,#24245,#24246,
#24247,#24248,#24249,#24250,#24251,#24252,#24253,#24254,#24255,#24256,#24257,
#24258,#24259,#24260,#24261,#24262,#24263,#24264,#24265,#24266,#24267,#24268,
#24269),.UNSPECIFIED.,.F.,.F.,(4,3,3,3,3,3,3,3,3,3,3,3,3,3,3,3,3,3,3,3,
3,3,3,3,3,3,3,3,3,3,3,4),(0.,0.0327225146876364,0.0662805432171355,0.10053700758566,
0.133256717128334,0.138569294358745,0.143645923792125,0.178633902850418,
0.21408079528951,0.251134267448895,0.278924371568434,0.28555899152832,0.321777086502174,
0.357762762756158,0.36229468392705,0.397656570072467,0.419708592270616,
0.427246251204994,0.432639262274467,0.468078659615991,0.504737305906693,
0.541740900625277,0.567834403702473,0.579481664146009,0.584481366534682,
0.622063534445468,0.654169882144813,0.668576745773135,0.678363380045444,
0.716158278526066,0.750488925242846,0.768398079192654),.UNSPECIFIED.);
#646=B_SPLINE_CURVE_WITH_KNOTS('',3,(#24270,#24271,#24272,#24273,#24274,
#24275,#24276,#24277,#24278,#24279,#24280,#24281,#24282,#24283,#24284,#24285,
#24286,#24287,#24288,#24289,#24290,#24291,#24292,#24293,#24294),
 .UNSPECIFIED.,.F.,.F.,(4,3,3,3,3,3,3,3,4),(7.59274844815667,7.89168714724002,
8.87814804064502,9.86460893405002,10.851069827455,11.83753072086,12.823991614265,
13.81045250767,13.8759337553363),.UNSPECIFIED.);
#1590=CYLINDRICAL_SURFACE('',#14527,3.5175);
#1591=CYLINDRICAL_SURFACE('',#14529,3.5175);
#1592=CYLINDRICAL_SURFACE('',#14530,3.5175);
#1593=CYLINDRICAL_SURFACE('',#14531,3.5175);
#1594=CYLINDRICAL_SURFACE('',#14532,3.5175);
#1595=CYLINDRICAL_SURFACE('',#14533,3.5175);
#1596=CYLINDRICAL_SURFACE('',#14534,3.5175);
#1597=CYLINDRICAL_SURFACE('',#14535,3.5175);
#1598=CYLINDRICAL_SURFACE('',#14537,3.5175);
#1599=CYLINDRICAL_SURFACE('',#14539,3.5175);
#1600=CYLINDRICAL_SURFACE('',#14540,3.5175);
#1601=CYLINDRICAL_SURFACE('',#14541,3.5175);
#1602=CYLINDRICAL_SURFACE('',#14542,3.5175);
#1603=CYLINDRICAL_SURFACE('',#14543,3.5175);
#1604=CYLINDRICAL_SURFACE('',#14544,3.5175);
#1605=CYLINDRICAL_SURFACE('',#14545,3.5175);
#1606=CYLINDRICAL_SURFACE('',#14547,3.5175);
#1607=CYLINDRICAL_SURFACE('',#14549,3.5175);
#1608=CYLINDRICAL_SURFACE('',#14550,3.5175);
#1609=CYLINDRICAL_SURFACE('',#14551,3.5175);
#1610=CYLINDRICAL_SURFACE('',#14552,3.5175);
#1611=CYLINDRICAL_SURFACE('',#14553,3.5175);
#1612=CYLINDRICAL_SURFACE('',#14554,3.5175);
#1613=CYLINDRICAL_SURFACE('',#14555,3.5175);
#1614=CYLINDRICAL_SURFACE('',#14557,3.5175);
#1615=CYLINDRICAL_SURFACE('',#14559,3.5175);
#1616=CYLINDRICAL_SURFACE('',#14560,3.5175);
#1617=CYLINDRICAL_SURFACE('',#14561,3.5175);
#1618=CYLINDRICAL_SURFACE('',#14562,3.5175);
#1619=CYLINDRICAL_SURFACE('',#14563,3.5175);
#1620=CYLINDRICAL_SURFACE('',#14564,3.5175);
#1621=CYLINDRICAL_SURFACE('',#14565,3.5175);
#1622=CYLINDRICAL_SURFACE('',#14567,4.07350000000001);
#1623=CYLINDRICAL_SURFACE('',#14569,4.07350000000001);
#1624=CYLINDRICAL_SURFACE('',#14570,4.07350000000001);
#1625=CYLINDRICAL_SURFACE('',#14571,4.07350000000001);
#1626=CYLINDRICAL_SURFACE('',#14572,4.07350000000001);
#1627=CYLINDRICAL_SURFACE('',#14573,4.07350000000001);
#1628=CYLINDRICAL_SURFACE('',#14574,4.07350000000001);
#1629=CYLINDRICAL_SURFACE('',#14575,4.07350000000001);
#1630=CYLINDRICAL_SURFACE('',#14577,4.07350000000001);
#1631=CYLINDRICAL_SURFACE('',#14579,4.07350000000001);
#1632=CYLINDRICAL_SURFACE('',#14580,4.07350000000001);
#1633=CYLINDRICAL_SURFACE('',#14581,4.07350000000001);
#1634=CYLINDRICAL_SURFACE('',#14582,4.07350000000001);
#1635=CYLINDRICAL_SURFACE('',#14583,4.07350000000001);
#1636=CYLINDRICAL_SURFACE('',#14584,4.07350000000001);
#1637=CYLINDRICAL_SURFACE('',#14585,4.07350000000001);
#1638=CYLINDRICAL_SURFACE('',#14587,4.0735);
#1639=CYLINDRICAL_SURFACE('',#14589,4.0735);
#1640=CYLINDRICAL_SURFACE('',#14590,4.0735);
#1641=CYLINDRICAL_SURFACE('',#14591,4.0735);
#1642=CYLINDRICAL_SURFACE('',#14592,4.0735);
#1643=CYLINDRICAL_SURFACE('',#14593,4.0735);
#1644=CYLINDRICAL_SURFACE('',#14594,4.0735);
#1645=CYLINDRICAL_SURFACE('',#14595,4.0735);
#1646=CYLINDRICAL_SURFACE('',#14597,4.0735);
#1647=CYLINDRICAL_SURFACE('',#14599,4.0735);
#1648=CYLINDRICAL_SURFACE('',#14600,4.0735);
#1649=CYLINDRICAL_SURFACE('',#14601,4.0735);
#1650=CYLINDRICAL_SURFACE('',#14602,4.0735);
#1651=CYLINDRICAL_SURFACE('',#14603,4.0735);
#1652=CYLINDRICAL_SURFACE('',#14604,4.0735);
#1653=CYLINDRICAL_SURFACE('',#14605,4.0735);
#1654=CYLINDRICAL_SURFACE('',#14607,4.0735);
#1655=CYLINDRICAL_SURFACE('',#14609,4.0735);
#1656=CYLINDRICAL_SURFACE('',#14610,4.07350000000001);
#1657=CYLINDRICAL_SURFACE('',#14611,4.07350000000001);
#1658=CYLINDRICAL_SURFACE('',#14612,3.5175);
#1659=CYLINDRICAL_SURFACE('',#14613,3.5175);
#1660=CYLINDRICAL_SURFACE('',#14614,3.5175);
#1661=CYLINDRICAL_SURFACE('',#14615,3.5175);
#2178=SHAPE_REPRESENTATION_RELATIONSHIP('SRR','None',#63862,#2194);
#2194=ADVANCED_BREP_SHAPE_REPRESENTATION('',(#2226),#63740);
#2210=STYLED_ITEM('',(#63959),#2226);
#2226=MANIFOLD_SOLID_BREP('Body1',#14311);
#2244=FACE_BOUND('',#3155,.T.);
#2245=FACE_BOUND('',#3156,.T.);
#2246=FACE_BOUND('',#3157,.T.);
#2247=FACE_BOUND('',#3158,.T.);
#2248=FACE_BOUND('',#3177,.T.);
#2249=FACE_BOUND('',#3178,.T.);
#2250=FACE_BOUND('',#3179,.T.);
#2251=FACE_BOUND('',#3180,.T.);
#2323=FACE_OUTER_BOUND('',#3087,.T.);
#2324=FACE_OUTER_BOUND('',#3088,.T.);
#2325=FACE_OUTER_BOUND('',#3089,.T.);
#2326=FACE_OUTER_BOUND('',#3090,.T.);
#2327=FACE_OUTER_BOUND('',#3091,.T.);
#2328=FACE_OUTER_BOUND('',#3092,.T.);
#2329=FACE_OUTER_BOUND('',#3093,.T.);
#2330=FACE_OUTER_BOUND('',#3094,.T.);
#2331=FACE_OUTER_BOUND('',#3095,.T.);
#2332=FACE_OUTER_BOUND('',#3096,.T.);
#2333=FACE_OUTER_BOUND('',#3097,.T.);
#2334=FACE_OUTER_BOUND('',#3098,.T.);
#2335=FACE_OUTER_BOUND('',#3099,.T.);
#2336=FACE_OUTER_BOUND('',#3100,.T.);
#2337=FACE_OUTER_BOUND('',#3101,.T.);
#2338=FACE_OUTER_BOUND('',#3102,.T.);
#2339=FACE_OUTER_BOUND('',#3103,.T.);
#2340=FACE_OUTER_BOUND('',#3104,.T.);
#2341=FACE_OUTER_BOUND('',#3105,.T.);
#2342=FACE_OUTER_BOUND('',#3106,.T.);
#2343=FACE_OUTER_BOUND('',#3107,.T.);
#2344=FACE_OUTER_BOUND('',#3108,.T.);
#2345=FACE_OUTER_BOUND('',#3109,.T.);
#2346=FACE_OUTER_BOUND('',#3110,.T.);
#2347=FACE_OUTER_BOUND('',#3111,.T.);
#2348=FACE_OUTER_BOUND('',#3112,.T.);
#2349=FACE_OUTER_BOUND('',#3113,.T.);
#2350=FACE_OUTER_BOUND('',#3114,.T.);
#2351=FACE_OUTER_BOUND('',#3115,.T.);
#2352=FACE_OUTER_BOUND('',#3116,.T.);
#2353=FACE_OUTER_BOUND('',#3117,.T.);
#2354=FACE_OUTER_BOUND('',#3118,.T.);
#2355=FACE_OUTER_BOUND('',#3119,.T.);
#2356=FACE_OUTER_BOUND('',#3120,.T.);
#2357=FACE_OUTER_BOUND('',#3121,.T.);
#2358=FACE_OUTER_BOUND('',#3122,.T.);
#2359=FACE_OUTER_BOUND('',#3123,.T.);
#2360=FACE_OUTER_BOUND('',#3124,.T.);
#2361=FACE_OUTER_BOUND('',#3125,.T.);
#2362=FACE_OUTER_BOUND('',#3126,.T.);
#2363=FACE_OUTER_BOUND('',#3127,.T.);
#2364=FACE_OUTER_BOUND('',#3128,.T.);
#2365=FACE_OUTER_BOUND('',#3129,.T.);
#2366=FACE_OUTER_BOUND('',#3130,.T.);
#2367=FACE_OUTER_BOUND('',#3131,.T.);
#2368=FACE_OUTER_BOUND('',#3132,.T.);
#2369=FACE_OUTER_BOUND('',#3133,.T.);
#2370=FACE_OUTER_BOUND('',#3134,.T.);
#2371=FACE_OUTER_BOUND('',#3135,.T.);
#2372=FACE_OUTER_BOUND('',#3136,.T.);
#2373=FACE_OUTER_BOUND('',#3137,.T.);
#2374=FACE_OUTER_BOUND('',#3138,.T.);
#2375=FACE_OUTER_BOUND('',#3139,.T.);
#2376=FACE_OUTER_BOUND('',#3140,.T.);
#2377=FACE_OUTER_BOUND('',#3141,.T.);
#2378=FACE_OUTER_BOUND('',#3142,.T.);
#2379=FACE_OUTER_BOUND('',#3143,.T.);
#2380=FACE_OUTER_BOUND('',#3144,.T.);
#2381=FACE_OUTER_BOUND('',#3145,.T.);
#2382=FACE_OUTER_BOUND('',#3146,.T.);
#2383=FACE_OUTER_BOUND('',#3147,.T.);
#2384=FACE_OUTER_BOUND('',#3148,.T.);
#2385=FACE_OUTER_BOUND('',#3149,.T.);
#2386=FACE_OUTER_BOUND('',#3150,.T.);
#2387=FACE_OUTER_BOUND('',#3151,.T.);
#2388=FACE_OUTER_BOUND('',#3152,.T.);
#2389=FACE_OUTER_BOUND('',#3153,.T.);
#2390=FACE_OUTER_BOUND('',#3154,.T.);
#2391=FACE_OUTER_BOUND('',#3159,.T.);
#2392=FACE_OUTER_BOUND('',#3160,.T.);
#2393=FACE_OUTER_BOUND('',#3161,.T.);
#2394=FACE_OUTER_BOUND('',#3162,.T.);
#2395=FACE_OUTER_BOUND('',#3163,.T.);
#2396=FACE_OUTER_BOUND('',#3164,.T.);
#2397=FACE_OUTER_BOUND('',#3165,.T.);
#2398=FACE_OUTER_BOUND('',#3166,.T.);
#2399=FACE_OUTER_BOUND('',#3167,.T.);
#2400=FACE_OUTER_BOUND('',#3168,.T.);
#2401=FACE_OUTER_BOUND('',#3169,.T.);
#2402=FACE_OUTER_BOUND('',#3170,.T.);
#2403=FACE_OUTER_BOUND('',#3171,.T.);
#2404=FACE_OUTER_BOUND('',#3172,.T.);
#2405=FACE_OUTER_BOUND('',#3173,.T.);
#2406=FACE_OUTER_BOUND('',#3174,.T.);
#2407=FACE_OUTER_BOUND('',#3175,.T.);
#2408=FACE_OUTER_BOUND('',#3176,.T.);
#3087=EDGE_LOOP('',(#9223,#9224,#9225,#9226));
#3088=EDGE_LOOP('',(#9227,#9228,#9229,#9230));
#3089=EDGE_LOOP('',(#9231,#9232,#9233,#9234));
#3090=EDGE_LOOP('',(#9235,#9236,#9237,#9238));
#3091=EDGE_LOOP('',(#9239,#9240,#9241,#9242));
#3092=EDGE_LOOP('',(#9243,#9244,#9245,#9246));
#3093=EDGE_LOOP('',(#9247,#9248,#9249,#9250));
#3094=EDGE_LOOP('',(#9251,#9252,#9253,#9254));
#3095=EDGE_LOOP('',(#9255,#9256,#9257,#9258));
#3096=EDGE_LOOP('',(#9259,#9260,#9261,#9262));
#3097=EDGE_LOOP('',(#9263,#9264,#9265,#9266));
#3098=EDGE_LOOP('',(#9267,#9268,#9269,#9270));
#3099=EDGE_LOOP('',(#9271,#9272,#9273,#9274));
#3100=EDGE_LOOP('',(#9275,#9276,#9277,#9278));
#3101=EDGE_LOOP('',(#9279,#9280,#9281,#9282));
#3102=EDGE_LOOP('',(#9283,#9284,#9285,#9286));
#3103=EDGE_LOOP('',(#9287,#9288,#9289,#9290));
#3104=EDGE_LOOP('',(#9291,#9292,#9293,#9294));
#3105=EDGE_LOOP('',(#9295,#9296,#9297,#9298));
#3106=EDGE_LOOP('',(#9299,#9300,#9301,#9302));
#3107=EDGE_LOOP('',(#9303,#9304,#9305,#9306));
#3108=EDGE_LOOP('',(#9307,#9308,#9309,#9310));
#3109=EDGE_LOOP('',(#9311,#9312,#9313,#9314));
#3110=EDGE_LOOP('',(#9315,#9316,#9317,#9318));
#3111=EDGE_LOOP('',(#9319,#9320,#9321,#9322));
#3112=EDGE_LOOP('',(#9323,#9324,#9325,#9326));
#3113=EDGE_LOOP('',(#9327,#9328,#9329,#9330));
#3114=EDGE_LOOP('',(#9331,#9332,#9333,#9334));
#3115=EDGE_LOOP('',(#9335,#9336,#9337,#9338));
#3116=EDGE_LOOP('',(#9339,#9340,#9341,#9342));
#3117=EDGE_LOOP('',(#9343,#9344,#9345,#9346));
#3118=EDGE_LOOP('',(#9347,#9348,#9349,#9350));
#3119=EDGE_LOOP('',(#9351,#9352,#9353,#9354));
#3120=EDGE_LOOP('',(#9355,#9356,#9357,#9358));
#3121=EDGE_LOOP('',(#9359,#9360,#9361,#9362));
#3122=EDGE_LOOP('',(#9363,#9364,#9365,#9366));
#3123=EDGE_LOOP('',(#9367,#9368,#9369,#9370));
#3124=EDGE_LOOP('',(#9371,#9372,#9373,#9374));
#3125=EDGE_LOOP('',(#9375,#9376,#9377,#9378));
#3126=EDGE_LOOP('',(#9379,#9380,#9381,#9382));
#3127=EDGE_LOOP('',(#9383,#9384,#9385,#9386));
#3128=EDGE_LOOP('',(#9387,#9388,#9389,#9390));
#3129=EDGE_LOOP('',(#9391,#9392,#9393,#9394));
#3130=EDGE_LOOP('',(#9395,#9396,#9397,#9398));
#3131=EDGE_LOOP('',(#9399,#9400,#9401,#9402));
#3132=EDGE_LOOP('',(#9403,#9404,#9405,#9406));
#3133=EDGE_LOOP('',(#9407,#9408,#9409,#9410));
#3134=EDGE_LOOP('',(#9411,#9412,#9413,#9414));
#3135=EDGE_LOOP('',(#9415,#9416,#9417,#9418));
#3136=EDGE_LOOP('',(#9419,#9420,#9421,#9422));
#3137=EDGE_LOOP('',(#9423,#9424,#9425,#9426));
#3138=EDGE_LOOP('',(#9427,#9428,#9429,#9430));
#3139=EDGE_LOOP('',(#9431,#9432,#9433,#9434));
#3140=EDGE_LOOP('',(#9435,#9436,#9437,#9438));
#3141=EDGE_LOOP('',(#9439,#9440,#9441,#9442));
#3142=EDGE_LOOP('',(#9443,#9444,#9445,#9446));
#3143=EDGE_LOOP('',(#9447,#9448,#9449,#9450));
#3144=EDGE_LOOP('',(#9451,#9452,#9453,#9454));
#3145=EDGE_LOOP('',(#9455,#9456,#9457,#9458));
#3146=EDGE_LOOP('',(#9459,#9460,#9461,#9462));
#3147=EDGE_LOOP('',(#9463,#9464,#9465,#9466));
#3148=EDGE_LOOP('',(#9467,#9468,#9469,#9470));
#3149=EDGE_LOOP('',(#9471,#9472,#9473,#9474));
#3150=EDGE_LOOP('',(#9475,#9476,#9477,#9478));
#3151=EDGE_LOOP('',(#9479,#9480,#9481,#9482));
#3152=EDGE_LOOP('',(#9483,#9484,#9485,#9486,#9487,#9488,#9489,#9490,#9491,
#9492,#9493,#9494,#9495,#9496,#9497,#9498,#9499,#9500,#9501,#9502));
#3153=EDGE_LOOP('',(#9503,#9504,#9505,#9506,#9507,#9508,#9509,#9510,#9511,
#9512,#9513,#9514,#9515,#9516,#9517,#9518,#9519,#9520,#9521,#9522));
#3154=EDGE_LOOP('',(#9523,#9524,#9525,#9526));
#3155=EDGE_LOOP('',(#9527,#9528,#9529,#9530));
#3156=EDGE_LOOP('',(#9531,#9532,#9533,#9534));
#3157=EDGE_LOOP('',(#9535,#9536,#9537,#9538));
#3158=EDGE_LOOP('',(#9539,#9540,#9541,#9542));
#3159=EDGE_LOOP('',(#9543,#9544,#9545,#9546));
#3160=EDGE_LOOP('',(#9547,#9548,#9549,#9550,#9551,#9552,#9553,#9554,#9555,
#9556,#9557,#9558,#9559,#9560,#9561,#9562,#9563,#9564,#9565,#9566));
#3161=EDGE_LOOP('',(#9567,#9568,#9569,#9570,#9571,#9572,#9573,#9574,#9575,
#9576,#9577,#9578,#9579,#9580,#9581,#9582,#9583,#9584,#9585,#9586));
#3162=EDGE_LOOP('',(#9587,#9588,#9589,#9590));
#3163=EDGE_LOOP('',(#9591,#9592,#9593,#9594,#9595,#9596,#9597,#9598,#9599,
#9600,#9601,#9602,#9603,#9604,#9605,#9606,#9607,#9608,#9609,#9610));
#3164=EDGE_LOOP('',(#9611,#9612,#9613,#9614,#9615,#9616,#9617,#9618,#9619,
#9620,#9621,#9622,#9623,#9624,#9625,#9626,#9627,#9628,#9629,#9630));
#3165=EDGE_LOOP('',(#9631,#9632,#9633,#9634));
#3166=EDGE_LOOP('',(#9635,#9636,#9637,#9638,#9639,#9640,#9641,#9642,#9643,
#9644,#9645,#9646,#9647,#9648,#9649,#9650,#9651,#9652,#9653,#9654));
#3167=EDGE_LOOP('',(#9655,#9656,#9657,#9658,#9659,#9660,#9661,#9662,#9663,
#9664,#9665,#9666,#9667,#9668,#9669,#9670,#9671,#9672,#9673,#9674));
#3168=EDGE_LOOP('',(#9675,#9676,#9677,#9678));
#3169=EDGE_LOOP('',(#9679,#9680,#9681,#9682));
#3170=EDGE_LOOP('',(#9683,#9684,#9685,#9686));
#3171=EDGE_LOOP('',(#9687,#9688,#9689,#9690));
#3172=EDGE_LOOP('',(#9691,#9692,#9693,#9694));
#3173=EDGE_LOOP('',(#9695,#9696,#9697,#9698));
#3174=EDGE_LOOP('',(#9699,#9700,#9701,#9702));
#3175=EDGE_LOOP('',(#9703,#9704,#9705,#9706));
#3176=EDGE_LOOP('',(#9707,#9708,#9709,#9710));
#3177=EDGE_LOOP('',(#9711,#9712,#9713,#9714));
#3178=EDGE_LOOP('',(#9715,#9716,#9717,#9718));
#3179=EDGE_LOOP('',(#9719,#9720,#9721,#9722));
#3180=EDGE_LOOP('',(#9723,#9724,#9725,#9726));
#3934=LINE('',#18485,#4770);
#3935=LINE('',#18506,#4771);
#3936=LINE('',#18557,#4772);
#3937=LINE('',#18608,#4773);
#3938=LINE('',#18656,#4774);
#3939=LINE('',#18707,#4775);
#3940=LINE('',#18758,#4776);
#3941=LINE('',#18806,#4777);
#3942=LINE('',#18845,#4778);
#3943=LINE('',#18866,#4779);
#3944=LINE('',#18917,#4780);
#3945=LINE('',#18968,#4781);
#3946=LINE('',#19016,#4782);
#3947=LINE('',#19067,#4783);
#3948=LINE('',#19118,#4784);
#3949=LINE('',#19166,#4785);
#3950=LINE('',#19205,#4786);
#3951=LINE('',#19226,#4787);
#3952=LINE('',#19277,#4788);
#3953=LINE('',#19328,#4789);
#3954=LINE('',#19376,#4790);
#3955=LINE('',#19427,#4791);
#3956=LINE('',#19478,#4792);
#3957=LINE('',#19526,#4793);
#3958=LINE('',#19565,#4794);
#3959=LINE('',#19586,#4795);
#3960=LINE('',#19637,#4796);
#3961=LINE('',#19688,#4797);
#3962=LINE('',#19736,#4798);
#3963=LINE('',#19787,#4799);
#3964=LINE('',#19838,#4800);
#3965=LINE('',#19886,#4801);
#3966=LINE('',#19925,#4802);
#3967=LINE('',#19949,#4803);
#3968=LINE('',#19973,#4804);
#3969=LINE('',#19998,#4805);
#3970=LINE('',#20023,#4806);
#3971=LINE('',#20047,#4807);
#3972=LINE('',#20072,#4808);
#3973=LINE('',#20097,#4809);
#3974=LINE('',#20114,#4810);
#3975=LINE('',#20138,#4811);
#3976=LINE('',#20162,#4812);
#3977=LINE('',#20187,#4813);
#3978=LINE('',#20212,#4814);
#3979=LINE('',#20236,#4815);
#3980=LINE('',#20261,#4816);
#3981=LINE('',#20286,#4817);
#3982=LINE('',#20303,#4818);
#3983=LINE('',#20327,#4819);
#3984=LINE('',#20351,#4820);
#3985=LINE('',#20376,#4821);
#3986=LINE('',#20401,#4822);
#3987=LINE('',#20425,#4823);
#3988=LINE('',#20450,#4824);
#3989=LINE('',#20475,#4825);
#3990=LINE('',#20492,#4826);
#3991=LINE('',#20516,#4827);
#3992=LINE('',#20540,#4828);
#3993=LINE('',#20565,#4829);
#3994=LINE('',#20590,#4830);
#3995=LINE('',#20614,#4831);
#3996=LINE('',#20639,#4832);
#3997=LINE('',#20664,#4833);
#3998=LINE('',#21583,#4834);
#3999=LINE('',#21585,#4835);
#4000=LINE('',#21587,#4836);
#4001=LINE('',#21588,#4837);
#4002=LINE('',#24302,#4838);
#4003=LINE('',#24303,#4839);
#4004=LINE('',#24304,#4840);
#4005=LINE('',#24307,#4841);
#4006=LINE('',#24308,#4842);
#4007=LINE('',#24311,#4843);
#4008=LINE('',#24312,#4844);
#4009=LINE('',#24314,#4845);
#4770=VECTOR('',#15615,4.);
#4771=VECTOR('',#15620,4.);
#4772=VECTOR('',#15623,4.);
#4773=VECTOR('',#15626,4.);
#4774=VECTOR('',#15629,4.);
#4775=VECTOR('',#15632,4.);
#4776=VECTOR('',#15635,4.);
#4777=VECTOR('',#15638,4.);
#4778=VECTOR('',#15643,4.);
#4779=VECTOR('',#15648,4.);
#4780=VECTOR('',#15651,4.);
#4781=VECTOR('',#15654,4.);
#4782=VECTOR('',#15657,4.);
#4783=VECTOR('',#15660,4.);
#4784=VECTOR('',#15663,4.);
#4785=VECTOR('',#15666,4.);
#4786=VECTOR('',#15671,4.);
#4787=VECTOR('',#15676,4.);
#4788=VECTOR('',#15679,4.);
#4789=VECTOR('',#15682,4.);
#4790=VECTOR('',#15685,4.);
#4791=VECTOR('',#15688,4.);
#4792=VECTOR('',#15691,4.);
#4793=VECTOR('',#15694,4.);
#4794=VECTOR('',#15699,4.);
#4795=VECTOR('',#15704,4.);
#4796=VECTOR('',#15707,4.);
#4797=VECTOR('',#15710,4.);
#4798=VECTOR('',#15713,4.);
#4799=VECTOR('',#15716,4.);
#4800=VECTOR('',#15719,4.);
#4801=VECTOR('',#15722,4.);
#4802=VECTOR('',#15727,4.07350000000001);
#4803=VECTOR('',#15732,4.07350000000001);
#4804=VECTOR('',#15735,4.07350000000001);
#4805=VECTOR('',#15738,4.07350000000001);
#4806=VECTOR('',#15741,4.07350000000001);
#4807=VECTOR('',#15744,4.07350000000001);
#4808=VECTOR('',#15747,4.07350000000001);
#4809=VECTOR('',#15750,4.07350000000001);
#4810=VECTOR('',#15755,4.07350000000001);
#4811=VECTOR('',#15760,4.07350000000001);
#4812=VECTOR('',#15763,4.07350000000001);
#4813=VECTOR('',#15766,4.07350000000001);
#4814=VECTOR('',#15769,4.07350000000001);
#4815=VECTOR('',#15772,4.07350000000001);
#4816=VECTOR('',#15775,4.07350000000001);
#4817=VECTOR('',#15778,4.07350000000001);
#4818=VECTOR('',#15783,4.0735);
#4819=VECTOR('',#15788,4.0735);
#4820=VECTOR('',#15791,4.0735);
#4821=VECTOR('',#15794,4.0735);
#4822=VECTOR('',#15797,4.0735);
#4823=VECTOR('',#15800,4.0735);
#4824=VECTOR('',#15803,4.0735);
#4825=VECTOR('',#15806,4.0735);
#4826=VECTOR('',#15811,4.0735);
#4827=VECTOR('',#15816,4.0735);
#4828=VECTOR('',#15819,4.0735);
#4829=VECTOR('',#15822,4.0735);
#4830=VECTOR('',#15825,4.0735);
#4831=VECTOR('',#15828,4.0735);
#4832=VECTOR('',#15831,4.0735);
#4833=VECTOR('',#15834,4.0735);
#4834=VECTOR('',#15841,10.);
#4835=VECTOR('',#15842,10.);
#4836=VECTOR('',#15843,10.);
#4837=VECTOR('',#15844,10.);
#4838=VECTOR('',#15861,10.);
#4839=VECTOR('',#15862,10.);
#4840=VECTOR('',#15863,10.);
#4841=VECTOR('',#15866,10.);
#4842=VECTOR('',#15867,10.);
#4843=VECTOR('',#15870,10.);
#4844=VECTOR('',#15871,10.);
#4845=VECTOR('',#15874,10.);
#5590=VERTEX_POINT('',#18483);
#5591=VERTEX_POINT('',#18484);
#5592=VERTEX_POINT('',#18486);
#5593=VERTEX_POINT('',#18491);
#5594=VERTEX_POINT('',#18504);
#5595=VERTEX_POINT('',#18505);
#5596=VERTEX_POINT('',#18555);
#5597=VERTEX_POINT('',#18556);
#5598=VERTEX_POINT('',#18606);
#5599=VERTEX_POINT('',#18607);
#5600=VERTEX_POINT('',#18654);
#5601=VERTEX_POINT('',#18655);
#5602=VERTEX_POINT('',#18705);
#5603=VERTEX_POINT('',#18706);
#5604=VERTEX_POINT('',#18756);
#5605=VERTEX_POINT('',#18757);
#5606=VERTEX_POINT('',#18804);
#5607=VERTEX_POINT('',#18805);
#5608=VERTEX_POINT('',#18807);
#5609=VERTEX_POINT('',#18821);
#5610=VERTEX_POINT('',#18843);
#5611=VERTEX_POINT('',#18844);
#5612=VERTEX_POINT('',#18846);
#5613=VERTEX_POINT('',#18851);
#5614=VERTEX_POINT('',#18864);
#5615=VERTEX_POINT('',#18865);
#5616=VERTEX_POINT('',#18915);
#5617=VERTEX_POINT('',#18916);
#5618=VERTEX_POINT('',#18966);
#5619=VERTEX_POINT('',#18967);
#5620=VERTEX_POINT('',#19014);
#5621=VERTEX_POINT('',#19015);
#5622=VERTEX_POINT('',#19065);
#5623=VERTEX_POINT('',#19066);
#5624=VERTEX_POINT('',#19116);
#5625=VERTEX_POINT('',#19117);
#5626=VERTEX_POINT('',#19164);
#5627=VERTEX_POINT('',#19165);
#5628=VERTEX_POINT('',#19167);
#5629=VERTEX_POINT('',#19181);
#5630=VERTEX_POINT('',#19203);
#5631=VERTEX_POINT('',#19204);
#5632=VERTEX_POINT('',#19206);
#5633=VERTEX_POINT('',#19211);
#5634=VERTEX_POINT('',#19224);
#5635=VERTEX_POINT('',#19225);
#5636=VERTEX_POINT('',#19275);
#5637=VERTEX_POINT('',#19276);
#5638=VERTEX_POINT('',#19326);
#5639=VERTEX_POINT('',#19327);
#5640=VERTEX_POINT('',#19374);
#5641=VERTEX_POINT('',#19375);
#5642=VERTEX_POINT('',#19425);
#5643=VERTEX_POINT('',#19426);
#5644=VERTEX_POINT('',#19476);
#5645=VERTEX_POINT('',#19477);
#5646=VERTEX_POINT('',#19524);
#5647=VERTEX_POINT('',#19525);
#5648=VERTEX_POINT('',#19527);
#5649=VERTEX_POINT('',#19541);
#5650=VERTEX_POINT('',#19563);
#5651=VERTEX_POINT('',#19564);
#5652=VERTEX_POINT('',#19566);
#5653=VERTEX_POINT('',#19571);
#5654=VERTEX_POINT('',#19584);
#5655=VERTEX_POINT('',#19585);
#5656=VERTEX_POINT('',#19635);
#5657=VERTEX_POINT('',#19636);
#5658=VERTEX_POINT('',#19686);
#5659=VERTEX_POINT('',#19687);
#5660=VERTEX_POINT('',#19734);
#5661=VERTEX_POINT('',#19735);
#5662=VERTEX_POINT('',#19785);
#5663=VERTEX_POINT('',#19786);
#5664=VERTEX_POINT('',#19836);
#5665=VERTEX_POINT('',#19837);
#5666=VERTEX_POINT('',#19884);
#5667=VERTEX_POINT('',#19885);
#5668=VERTEX_POINT('',#19887);
#5669=VERTEX_POINT('',#19901);
#5670=VERTEX_POINT('',#19923);
#5671=VERTEX_POINT('',#19924);
#5672=VERTEX_POINT('',#19926);
#5673=VERTEX_POINT('',#19935);
#5674=VERTEX_POINT('',#19947);
#5675=VERTEX_POINT('',#19948);
#5676=VERTEX_POINT('',#19971);
#5677=VERTEX_POINT('',#19972);
#5678=VERTEX_POINT('',#19996);
#5679=VERTEX_POINT('',#19997);
#5680=VERTEX_POINT('',#20021);
#5681=VERTEX_POINT('',#20022);
#5682=VERTEX_POINT('',#20045);
#5683=VERTEX_POINT('',#20046);
#5684=VERTEX_POINT('',#20070);
#5685=VERTEX_POINT('',#20071);
#5686=VERTEX_POINT('',#20095);
#5687=VERTEX_POINT('',#20096);
#5688=VERTEX_POINT('',#20098);
#5689=VERTEX_POINT('',#20104);
#5690=VERTEX_POINT('',#20112);
#5691=VERTEX_POINT('',#20113);
#5692=VERTEX_POINT('',#20115);
#5693=VERTEX_POINT('',#20124);
#5694=VERTEX_POINT('',#20136);
#5695=VERTEX_POINT('',#20137);
#5696=VERTEX_POINT('',#20160);
#5697=VERTEX_POINT('',#20161);
#5698=VERTEX_POINT('',#20185);
#5699=VERTEX_POINT('',#20186);
#5700=VERTEX_POINT('',#20210);
#5701=VERTEX_POINT('',#20211);
#5702=VERTEX_POINT('',#20234);
#5703=VERTEX_POINT('',#20235);
#5704=VERTEX_POINT('',#20259);
#5705=VERTEX_POINT('',#20260);
#5706=VERTEX_POINT('',#20284);
#5707=VERTEX_POINT('',#20285);
#5708=VERTEX_POINT('',#20287);
#5709=VERTEX_POINT('',#20293);
#5710=VERTEX_POINT('',#20301);
#5711=VERTEX_POINT('',#20302);
#5712=VERTEX_POINT('',#20304);
#5713=VERTEX_POINT('',#20313);
#5714=VERTEX_POINT('',#20325);
#5715=VERTEX_POINT('',#20326);
#5716=VERTEX_POINT('',#20349);
#5717=VERTEX_POINT('',#20350);
#5718=VERTEX_POINT('',#20374);
#5719=VERTEX_POINT('',#20375);
#5720=VERTEX_POINT('',#20399);
#5721=VERTEX_POINT('',#20400);
#5722=VERTEX_POINT('',#20423);
#5723=VERTEX_POINT('',#20424);
#5724=VERTEX_POINT('',#20448);
#5725=VERTEX_POINT('',#20449);
#5726=VERTEX_POINT('',#20473);
#5727=VERTEX_POINT('',#20474);
#5728=VERTEX_POINT('',#20476);
#5729=VERTEX_POINT('',#20482);
#5730=VERTEX_POINT('',#20490);
#5731=VERTEX_POINT('',#20491);
#5732=VERTEX_POINT('',#20493);
#5733=VERTEX_POINT('',#20502);
#5734=VERTEX_POINT('',#20514);
#5735=VERTEX_POINT('',#20515);
#5736=VERTEX_POINT('',#20538);
#5737=VERTEX_POINT('',#20539);
#5738=VERTEX_POINT('',#20563);
#5739=VERTEX_POINT('',#20564);
#5740=VERTEX_POINT('',#20588);
#5741=VERTEX_POINT('',#20589);
#5742=VERTEX_POINT('',#20612);
#5743=VERTEX_POINT('',#20613);
#5744=VERTEX_POINT('',#20637);
#5745=VERTEX_POINT('',#20638);
#5746=VERTEX_POINT('',#20662);
#5747=VERTEX_POINT('',#20663);
#5748=VERTEX_POINT('',#20665);
#5749=VERTEX_POINT('',#20671);
#5750=VERTEX_POINT('',#21581);
#5751=VERTEX_POINT('',#21582);
#5752=VERTEX_POINT('',#21584);
#5753=VERTEX_POINT('',#21586);
#5754=VERTEX_POINT('',#24300);
#5755=VERTEX_POINT('',#24301);
#5756=VERTEX_POINT('',#24306);
#5757=VERTEX_POINT('',#24310);
#7034=EDGE_CURVE('',#5590,#5591,#3934,.T.);
#7035=EDGE_CURVE('',#5591,#5592,#487,.T.);
#7036=EDGE_CURVE('',#5593,#5592,#285,.F.);
#7037=EDGE_CURVE('',#5593,#5590,#488,.T.);
#7038=EDGE_CURVE('',#5594,#5595,#3935,.T.);
#7039=EDGE_CURVE('',#5595,#5591,#489,.T.);
#7040=EDGE_CURVE('',#5590,#5594,#490,.T.);
#7041=EDGE_CURVE('',#5596,#5597,#3936,.T.);
#7042=EDGE_CURVE('',#5597,#5595,#491,.T.);
#7043=EDGE_CURVE('',#5594,#5596,#492,.T.);
#7044=EDGE_CURVE('',#5598,#5599,#3937,.T.);
#7045=EDGE_CURVE('',#5599,#5597,#493,.T.);
#7046=EDGE_CURVE('',#5596,#5598,#494,.T.);
#7047=EDGE_CURVE('',#5600,#5601,#3938,.T.);
#7048=EDGE_CURVE('',#5601,#5599,#495,.T.);
#7049=EDGE_CURVE('',#5598,#5600,#496,.T.);
#7050=EDGE_CURVE('',#5602,#5603,#3939,.T.);
#7051=EDGE_CURVE('',#5603,#5601,#497,.T.);
#7052=EDGE_CURVE('',#5600,#5602,#498,.T.);
#7053=EDGE_CURVE('',#5604,#5605,#3940,.T.);
#7054=EDGE_CURVE('',#5605,#5603,#499,.T.);
#7055=EDGE_CURVE('',#5602,#5604,#500,.T.);
#7056=EDGE_CURVE('',#5606,#5607,#3941,.T.);
#7057=EDGE_CURVE('',#5606,#5608,#501,.T.);
#7058=EDGE_CURVE('',#5609,#5608,#286,.T.);
#7059=EDGE_CURVE('',#5609,#5607,#502,.T.);
#7060=EDGE_CURVE('',#5610,#5611,#3942,.T.);
#7061=EDGE_CURVE('',#5611,#5612,#503,.T.);
#7062=EDGE_CURVE('',#5613,#5612,#287,.F.);
#7063=EDGE_CURVE('',#5613,#5610,#504,.T.);
#7064=EDGE_CURVE('',#5614,#5615,#3943,.T.);
#7065=EDGE_CURVE('',#5615,#5611,#505,.T.);
#7066=EDGE_CURVE('',#5610,#5614,#506,.T.);
#7067=EDGE_CURVE('',#5616,#5617,#3944,.T.);
#7068=EDGE_CURVE('',#5617,#5615,#507,.T.);
#7069=EDGE_CURVE('',#5614,#5616,#508,.T.);
#7070=EDGE_CURVE('',#5618,#5619,#3945,.T.);
#7071=EDGE_CURVE('',#5619,#5617,#509,.T.);
#7072=EDGE_CURVE('',#5616,#5618,#510,.T.);
#7073=EDGE_CURVE('',#5620,#5621,#3946,.T.);
#7074=EDGE_CURVE('',#5621,#5619,#511,.T.);
#7075=EDGE_CURVE('',#5618,#5620,#512,.T.);
#7076=EDGE_CURVE('',#5622,#5623,#3947,.T.);
#7077=EDGE_CURVE('',#5623,#5621,#513,.T.);
#7078=EDGE_CURVE('',#5620,#5622,#514,.T.);
#7079=EDGE_CURVE('',#5624,#5625,#3948,.T.);
#7080=EDGE_CURVE('',#5625,#5623,#515,.T.);
#7081=EDGE_CURVE('',#5622,#5624,#516,.T.);
#7082=EDGE_CURVE('',#5626,#5627,#3949,.T.);
#7083=EDGE_CURVE('',#5626,#5628,#517,.T.);
#7084=EDGE_CURVE('',#5629,#5628,#288,.T.);
#7085=EDGE_CURVE('',#5629,#5627,#518,.T.);
#7086=EDGE_CURVE('',#5630,#5631,#3950,.T.);
#7087=EDGE_CURVE('',#5631,#5632,#519,.T.);
#7088=EDGE_CURVE('',#5633,#5632,#289,.F.);
#7089=EDGE_CURVE('',#5633,#5630,#520,.T.);
#7090=EDGE_CURVE('',#5634,#5635,#3951,.T.);
#7091=EDGE_CURVE('',#5635,#5631,#521,.T.);
#7092=EDGE_CURVE('',#5630,#5634,#522,.T.);
#7093=EDGE_CURVE('',#5636,#5637,#3952,.T.);
#7094=EDGE_CURVE('',#5637,#5635,#523,.T.);
#7095=EDGE_CURVE('',#5634,#5636,#524,.T.);
#7096=EDGE_CURVE('',#5638,#5639,#3953,.T.);
#7097=EDGE_CURVE('',#5639,#5637,#525,.T.);
#7098=EDGE_CURVE('',#5636,#5638,#526,.T.);
#7099=EDGE_CURVE('',#5640,#5641,#3954,.T.);
#7100=EDGE_CURVE('',#5641,#5639,#527,.T.);
#7101=EDGE_CURVE('',#5638,#5640,#528,.T.);
#7102=EDGE_CURVE('',#5642,#5643,#3955,.T.);
#7103=EDGE_CURVE('',#5643,#5641,#529,.T.);
#7104=EDGE_CURVE('',#5640,#5642,#530,.T.);
#7105=EDGE_CURVE('',#5644,#5645,#3956,.T.);
#7106=EDGE_CURVE('',#5645,#5643,#531,.T.);
#7107=EDGE_CURVE('',#5642,#5644,#532,.T.);
#7108=EDGE_CURVE('',#5646,#5647,#3957,.T.);
#7109=EDGE_CURVE('',#5646,#5648,#533,.T.);
#7110=EDGE_CURVE('',#5649,#5648,#290,.T.);
#7111=EDGE_CURVE('',#5649,#5647,#534,.T.);
#7112=EDGE_CURVE('',#5650,#5651,#3958,.T.);
#7113=EDGE_CURVE('',#5651,#5652,#535,.T.);
#7114=EDGE_CURVE('',#5653,#5652,#291,.F.);
#7115=EDGE_CURVE('',#5653,#5650,#536,.T.);
#7116=EDGE_CURVE('',#5654,#5655,#3959,.T.);
#7117=EDGE_CURVE('',#5655,#5651,#537,.T.);
#7118=EDGE_CURVE('',#5650,#5654,#538,.T.);
#7119=EDGE_CURVE('',#5656,#5657,#3960,.T.);
#7120=EDGE_CURVE('',#5657,#5655,#539,.T.);
#7121=EDGE_CURVE('',#5654,#5656,#540,.T.);
#7122=EDGE_CURVE('',#5658,#5659,#3961,.T.);
#7123=EDGE_CURVE('',#5659,#5657,#541,.T.);
#7124=EDGE_CURVE('',#5656,#5658,#542,.T.);
#7125=EDGE_CURVE('',#5660,#5661,#3962,.T.);
#7126=EDGE_CURVE('',#5661,#5659,#543,.T.);
#7127=EDGE_CURVE('',#5658,#5660,#544,.T.);
#7128=EDGE_CURVE('',#5662,#5663,#3963,.T.);
#7129=EDGE_CURVE('',#5663,#5661,#545,.T.);
#7130=EDGE_CURVE('',#5660,#5662,#546,.T.);
#7131=EDGE_CURVE('',#5664,#5665,#3964,.T.);
#7132=EDGE_CURVE('',#5665,#5663,#547,.T.);
#7133=EDGE_CURVE('',#5662,#5664,#548,.T.);
#7134=EDGE_CURVE('',#5666,#5667,#3965,.T.);
#7135=EDGE_CURVE('',#5666,#5668,#549,.T.);
#7136=EDGE_CURVE('',#5669,#5668,#292,.T.);
#7137=EDGE_CURVE('',#5669,#5667,#550,.T.);
#7138=EDGE_CURVE('',#5670,#5671,#3966,.T.);
#7139=EDGE_CURVE('',#5671,#5672,#551,.T.);
#7140=EDGE_CURVE('',#5673,#5672,#293,.T.);
#7141=EDGE_CURVE('',#5670,#5673,#552,.T.);
#7142=EDGE_CURVE('',#5674,#5675,#3967,.T.);
#7143=EDGE_CURVE('',#5675,#5671,#553,.T.);
#7144=EDGE_CURVE('',#5674,#5670,#554,.T.);
#7145=EDGE_CURVE('',#5676,#5677,#3968,.T.);
#7146=EDGE_CURVE('',#5677,#5675,#555,.T.);
#7147=EDGE_CURVE('',#5676,#5674,#556,.T.);
#7148=EDGE_CURVE('',#5678,#5679,#3969,.T.);
#7149=EDGE_CURVE('',#5679,#5677,#557,.T.);
#7150=EDGE_CURVE('',#5678,#5676,#558,.T.);
#7151=EDGE_CURVE('',#5680,#5681,#3970,.T.);
#7152=EDGE_CURVE('',#5681,#5679,#559,.T.);
#7153=EDGE_CURVE('',#5680,#5678,#560,.T.);
#7154=EDGE_CURVE('',#5682,#5683,#3971,.T.);
#7155=EDGE_CURVE('',#5683,#5681,#561,.T.);
#7156=EDGE_CURVE('',#5682,#5680,#562,.T.);
#7157=EDGE_CURVE('',#5684,#5685,#3972,.T.);
#7158=EDGE_CURVE('',#5685,#5683,#563,.T.);
#7159=EDGE_CURVE('',#5684,#5682,#564,.T.);
#7160=EDGE_CURVE('',#5686,#5687,#3973,.T.);
#7161=EDGE_CURVE('',#5688,#5686,#565,.T.);
#7162=EDGE_CURVE('',#5689,#5688,#294,.T.);
#7163=EDGE_CURVE('',#5689,#5687,#566,.T.);
#7164=EDGE_CURVE('',#5690,#5691,#3974,.T.);
#7165=EDGE_CURVE('',#5691,#5692,#567,.T.);
#7166=EDGE_CURVE('',#5693,#5692,#295,.T.);
#7167=EDGE_CURVE('',#5690,#5693,#568,.T.);
#7168=EDGE_CURVE('',#5694,#5695,#3975,.T.);
#7169=EDGE_CURVE('',#5695,#5691,#569,.T.);
#7170=EDGE_CURVE('',#5694,#5690,#570,.T.);
#7171=EDGE_CURVE('',#5696,#5697,#3976,.T.);
#7172=EDGE_CURVE('',#5697,#5695,#571,.T.);
#7173=EDGE_CURVE('',#5696,#5694,#572,.T.);
#7174=EDGE_CURVE('',#5698,#5699,#3977,.T.);
#7175=EDGE_CURVE('',#5699,#5697,#573,.T.);
#7176=EDGE_CURVE('',#5698,#5696,#574,.T.);
#7177=EDGE_CURVE('',#5700,#5701,#3978,.T.);
#7178=EDGE_CURVE('',#5701,#5699,#575,.T.);
#7179=EDGE_CURVE('',#5700,#5698,#576,.T.);
#7180=EDGE_CURVE('',#5702,#5703,#3979,.T.);
#7181=EDGE_CURVE('',#5703,#5701,#577,.T.);
#7182=EDGE_CURVE('',#5702,#5700,#578,.T.);
#7183=EDGE_CURVE('',#5704,#5705,#3980,.T.);
#7184=EDGE_CURVE('',#5705,#5703,#579,.T.);
#7185=EDGE_CURVE('',#5704,#5702,#580,.T.);
#7186=EDGE_CURVE('',#5706,#5707,#3981,.T.);
#7187=EDGE_CURVE('',#5708,#5706,#581,.T.);
#7188=EDGE_CURVE('',#5709,#5708,#296,.T.);
#7189=EDGE_CURVE('',#5709,#5707,#582,.T.);
#7190=EDGE_CURVE('',#5710,#5711,#3982,.T.);
#7191=EDGE_CURVE('',#5711,#5712,#583,.T.);
#7192=EDGE_CURVE('',#5713,#5712,#297,.T.);
#7193=EDGE_CURVE('',#5710,#5713,#584,.T.);
#7194=EDGE_CURVE('',#5714,#5715,#3983,.T.);
#7195=EDGE_CURVE('',#5715,#5711,#585,.T.);
#7196=EDGE_CURVE('',#5714,#5710,#586,.T.);
#7197=EDGE_CURVE('',#5716,#5717,#3984,.T.);
#7198=EDGE_CURVE('',#5717,#5715,#587,.T.);
#7199=EDGE_CURVE('',#5716,#5714,#588,.T.);
#7200=EDGE_CURVE('',#5718,#5719,#3985,.T.);
#7201=EDGE_CURVE('',#5719,#5717,#589,.T.);
#7202=EDGE_CURVE('',#5718,#5716,#590,.T.);
#7203=EDGE_CURVE('',#5720,#5721,#3986,.T.);
#7204=EDGE_CURVE('',#5721,#5719,#591,.T.);
#7205=EDGE_CURVE('',#5720,#5718,#592,.T.);
#7206=EDGE_CURVE('',#5722,#5723,#3987,.T.);
#7207=EDGE_CURVE('',#5723,#5721,#593,.T.);
#7208=EDGE_CURVE('',#5722,#5720,#594,.T.);
#7209=EDGE_CURVE('',#5724,#5725,#3988,.T.);
#7210=EDGE_CURVE('',#5725,#5723,#595,.T.);
#7211=EDGE_CURVE('',#5724,#5722,#596,.T.);
#7212=EDGE_CURVE('',#5726,#5727,#3989,.T.);
#7213=EDGE_CURVE('',#5728,#5726,#597,.T.);
#7214=EDGE_CURVE('',#5729,#5728,#298,.T.);
#7215=EDGE_CURVE('',#5729,#5727,#598,.T.);
#7216=EDGE_CURVE('',#5730,#5731,#3990,.T.);
#7217=EDGE_CURVE('',#5731,#5732,#599,.T.);
#7218=EDGE_CURVE('',#5733,#5732,#299,.T.);
#7219=EDGE_CURVE('',#5730,#5733,#600,.T.);
#7220=EDGE_CURVE('',#5734,#5735,#3991,.T.);
#7221=EDGE_CURVE('',#5735,#5731,#601,.T.);
#7222=EDGE_CURVE('',#5734,#5730,#602,.T.);
#7223=EDGE_CURVE('',#5736,#5737,#3992,.T.);
#7224=EDGE_CURVE('',#5737,#5735,#603,.T.);
#7225=EDGE_CURVE('',#5736,#5734,#604,.T.);
#7226=EDGE_CURVE('',#5738,#5739,#3993,.T.);
#7227=EDGE_CURVE('',#5739,#5737,#605,.T.);
#7228=EDGE_CURVE('',#5738,#5736,#606,.T.);
#7229=EDGE_CURVE('',#5740,#5741,#3994,.T.);
#7230=EDGE_CURVE('',#5741,#5739,#607,.T.);
#7231=EDGE_CURVE('',#5740,#5738,#608,.T.);
#7232=EDGE_CURVE('',#5742,#5743,#3995,.T.);
#7233=EDGE_CURVE('',#5743,#5741,#609,.T.);
#7234=EDGE_CURVE('',#5742,#5740,#610,.T.);
#7235=EDGE_CURVE('',#5744,#5745,#3996,.T.);
#7236=EDGE_CURVE('',#5745,#5743,#611,.T.);
#7237=EDGE_CURVE('',#5744,#5742,#612,.T.);
#7238=EDGE_CURVE('',#5746,#5747,#3997,.T.);
#7239=EDGE_CURVE('',#5748,#5746,#613,.T.);
#7240=EDGE_CURVE('',#5749,#5748,#300,.T.);
#7241=EDGE_CURVE('',#5749,#5747,#614,.T.);
#7242=EDGE_CURVE('',#5747,#5745,#615,.T.);
#7243=EDGE_CURVE('',#5746,#5744,#616,.T.);
#7244=EDGE_CURVE('',#5732,#5653,#617,.T.);
#7245=EDGE_CURVE('',#5668,#5749,#618,.T.);
#7246=EDGE_CURVE('',#5664,#5666,#619,.T.);
#7247=EDGE_CURVE('',#5652,#5733,#620,.T.);
#7248=EDGE_CURVE('',#5667,#5665,#621,.T.);
#7249=EDGE_CURVE('',#5748,#5669,#622,.T.);
#7250=EDGE_CURVE('',#5750,#5751,#3998,.T.);
#7251=EDGE_CURVE('',#5751,#5752,#3999,.T.);
#7252=EDGE_CURVE('',#5752,#5753,#4000,.T.);
#7253=EDGE_CURVE('',#5753,#5750,#4001,.T.);
#7254=EDGE_CURVE('',#5648,#5729,#623,.T.);
#7255=EDGE_CURVE('',#5728,#5649,#624,.T.);
#7256=EDGE_CURVE('',#5628,#5689,#625,.T.);
#7257=EDGE_CURVE('',#5688,#5629,#626,.T.);
#7258=EDGE_CURVE('',#5608,#5709,#627,.T.);
#7259=EDGE_CURVE('',#5708,#5609,#628,.T.);
#7260=EDGE_CURVE('',#5727,#5725,#629,.T.);
#7261=EDGE_CURVE('',#5726,#5724,#630,.T.);
#7262=EDGE_CURVE('',#5712,#5633,#631,.T.);
#7263=EDGE_CURVE('',#5644,#5646,#632,.T.);
#7264=EDGE_CURVE('',#5632,#5713,#633,.T.);
#7265=EDGE_CURVE('',#5647,#5645,#634,.T.);
#7266=EDGE_CURVE('',#5707,#5705,#635,.T.);
#7267=EDGE_CURVE('',#5706,#5704,#636,.T.);
#7268=EDGE_CURVE('',#5692,#5593,#637,.T.);
#7269=EDGE_CURVE('',#5604,#5606,#638,.T.);
#7270=EDGE_CURVE('',#5592,#5693,#639,.T.);
#7271=EDGE_CURVE('',#5607,#5605,#640,.T.);
#7272=EDGE_CURVE('',#5687,#5685,#641,.T.);
#7273=EDGE_CURVE('',#5686,#5684,#642,.T.);
#7274=EDGE_CURVE('',#5672,#5613,#643,.T.);
#7275=EDGE_CURVE('',#5624,#5626,#644,.T.);
#7276=EDGE_CURVE('',#5612,#5673,#645,.T.);
#7277=EDGE_CURVE('',#5627,#5625,#646,.T.);
#7278=EDGE_CURVE('',#5754,#5755,#4002,.T.);
#7279=EDGE_CURVE('',#5755,#5750,#4003,.T.);
#7280=EDGE_CURVE('',#5754,#5753,#4004,.T.);
#7281=EDGE_CURVE('',#5756,#5754,#4005,.T.);
#7282=EDGE_CURVE('',#5756,#5752,#4006,.T.);
#7283=EDGE_CURVE('',#5757,#5756,#4007,.T.);
#7284=EDGE_CURVE('',#5757,#5751,#4008,.T.);
#7285=EDGE_CURVE('',#5755,#5757,#4009,.T.);
#9223=ORIENTED_EDGE('',*,*,#7034,.T.);
#9224=ORIENTED_EDGE('',*,*,#7035,.T.);
#9225=ORIENTED_EDGE('',*,*,#7036,.F.);
#9226=ORIENTED_EDGE('',*,*,#7037,.T.);
#9227=ORIENTED_EDGE('',*,*,#7038,.T.);
#9228=ORIENTED_EDGE('',*,*,#7039,.T.);
#9229=ORIENTED_EDGE('',*,*,#7034,.F.);
#9230=ORIENTED_EDGE('',*,*,#7040,.T.);
#9231=ORIENTED_EDGE('',*,*,#7041,.T.);
#9232=ORIENTED_EDGE('',*,*,#7042,.T.);
#9233=ORIENTED_EDGE('',*,*,#7038,.F.);
#9234=ORIENTED_EDGE('',*,*,#7043,.T.);
#9235=ORIENTED_EDGE('',*,*,#7044,.T.);
#9236=ORIENTED_EDGE('',*,*,#7045,.T.);
#9237=ORIENTED_EDGE('',*,*,#7041,.F.);
#9238=ORIENTED_EDGE('',*,*,#7046,.T.);
#9239=ORIENTED_EDGE('',*,*,#7047,.T.);
#9240=ORIENTED_EDGE('',*,*,#7048,.T.);
#9241=ORIENTED_EDGE('',*,*,#7044,.F.);
#9242=ORIENTED_EDGE('',*,*,#7049,.T.);
#9243=ORIENTED_EDGE('',*,*,#7050,.T.);
#9244=ORIENTED_EDGE('',*,*,#7051,.T.);
#9245=ORIENTED_EDGE('',*,*,#7047,.F.);
#9246=ORIENTED_EDGE('',*,*,#7052,.T.);
#9247=ORIENTED_EDGE('',*,*,#7053,.T.);
#9248=ORIENTED_EDGE('',*,*,#7054,.T.);
#9249=ORIENTED_EDGE('',*,*,#7050,.F.);
#9250=ORIENTED_EDGE('',*,*,#7055,.T.);
#9251=ORIENTED_EDGE('',*,*,#7056,.F.);
#9252=ORIENTED_EDGE('',*,*,#7057,.T.);
#9253=ORIENTED_EDGE('',*,*,#7058,.F.);
#9254=ORIENTED_EDGE('',*,*,#7059,.T.);
#9255=ORIENTED_EDGE('',*,*,#7060,.T.);
#9256=ORIENTED_EDGE('',*,*,#7061,.T.);
#9257=ORIENTED_EDGE('',*,*,#7062,.F.);
#9258=ORIENTED_EDGE('',*,*,#7063,.T.);
#9259=ORIENTED_EDGE('',*,*,#7064,.T.);
#9260=ORIENTED_EDGE('',*,*,#7065,.T.);
#9261=ORIENTED_EDGE('',*,*,#7060,.F.);
#9262=ORIENTED_EDGE('',*,*,#7066,.T.);
#9263=ORIENTED_EDGE('',*,*,#7067,.T.);
#9264=ORIENTED_EDGE('',*,*,#7068,.T.);
#9265=ORIENTED_EDGE('',*,*,#7064,.F.);
#9266=ORIENTED_EDGE('',*,*,#7069,.T.);
#9267=ORIENTED_EDGE('',*,*,#7070,.T.);
#9268=ORIENTED_EDGE('',*,*,#7071,.T.);
#9269=ORIENTED_EDGE('',*,*,#7067,.F.);
#9270=ORIENTED_EDGE('',*,*,#7072,.T.);
#9271=ORIENTED_EDGE('',*,*,#7073,.T.);
#9272=ORIENTED_EDGE('',*,*,#7074,.T.);
#9273=ORIENTED_EDGE('',*,*,#7070,.F.);
#9274=ORIENTED_EDGE('',*,*,#7075,.T.);
#9275=ORIENTED_EDGE('',*,*,#7076,.T.);
#9276=ORIENTED_EDGE('',*,*,#7077,.T.);
#9277=ORIENTED_EDGE('',*,*,#7073,.F.);
#9278=ORIENTED_EDGE('',*,*,#7078,.T.);
#9279=ORIENTED_EDGE('',*,*,#7079,.T.);
#9280=ORIENTED_EDGE('',*,*,#7080,.T.);
#9281=ORIENTED_EDGE('',*,*,#7076,.F.);
#9282=ORIENTED_EDGE('',*,*,#7081,.T.);
#9283=ORIENTED_EDGE('',*,*,#7082,.F.);
#9284=ORIENTED_EDGE('',*,*,#7083,.T.);
#9285=ORIENTED_EDGE('',*,*,#7084,.F.);
#9286=ORIENTED_EDGE('',*,*,#7085,.T.);
#9287=ORIENTED_EDGE('',*,*,#7086,.T.);
#9288=ORIENTED_EDGE('',*,*,#7087,.T.);
#9289=ORIENTED_EDGE('',*,*,#7088,.F.);
#9290=ORIENTED_EDGE('',*,*,#7089,.T.);
#9291=ORIENTED_EDGE('',*,*,#7090,.T.);
#9292=ORIENTED_EDGE('',*,*,#7091,.T.);
#9293=ORIENTED_EDGE('',*,*,#7086,.F.);
#9294=ORIENTED_EDGE('',*,*,#7092,.T.);
#9295=ORIENTED_EDGE('',*,*,#7093,.T.);
#9296=ORIENTED_EDGE('',*,*,#7094,.T.);
#9297=ORIENTED_EDGE('',*,*,#7090,.F.);
#9298=ORIENTED_EDGE('',*,*,#7095,.T.);
#9299=ORIENTED_EDGE('',*,*,#7096,.T.);
#9300=ORIENTED_EDGE('',*,*,#7097,.T.);
#9301=ORIENTED_EDGE('',*,*,#7093,.F.);
#9302=ORIENTED_EDGE('',*,*,#7098,.T.);
#9303=ORIENTED_EDGE('',*,*,#7099,.T.);
#9304=ORIENTED_EDGE('',*,*,#7100,.T.);
#9305=ORIENTED_EDGE('',*,*,#7096,.F.);
#9306=ORIENTED_EDGE('',*,*,#7101,.T.);
#9307=ORIENTED_EDGE('',*,*,#7102,.T.);
#9308=ORIENTED_EDGE('',*,*,#7103,.T.);
#9309=ORIENTED_EDGE('',*,*,#7099,.F.);
#9310=ORIENTED_EDGE('',*,*,#7104,.T.);
#9311=ORIENTED_EDGE('',*,*,#7105,.T.);
#9312=ORIENTED_EDGE('',*,*,#7106,.T.);
#9313=ORIENTED_EDGE('',*,*,#7102,.F.);
#9314=ORIENTED_EDGE('',*,*,#7107,.T.);
#9315=ORIENTED_EDGE('',*,*,#7108,.F.);
#9316=ORIENTED_EDGE('',*,*,#7109,.T.);
#9317=ORIENTED_EDGE('',*,*,#7110,.F.);
#9318=ORIENTED_EDGE('',*,*,#7111,.T.);
#9319=ORIENTED_EDGE('',*,*,#7112,.T.);
#9320=ORIENTED_EDGE('',*,*,#7113,.T.);
#9321=ORIENTED_EDGE('',*,*,#7114,.F.);
#9322=ORIENTED_EDGE('',*,*,#7115,.T.);
#9323=ORIENTED_EDGE('',*,*,#7116,.T.);
#9324=ORIENTED_EDGE('',*,*,#7117,.T.);
#9325=ORIENTED_EDGE('',*,*,#7112,.F.);
#9326=ORIENTED_EDGE('',*,*,#7118,.T.);
#9327=ORIENTED_EDGE('',*,*,#7119,.T.);
#9328=ORIENTED_EDGE('',*,*,#7120,.T.);
#9329=ORIENTED_EDGE('',*,*,#7116,.F.);
#9330=ORIENTED_EDGE('',*,*,#7121,.T.);
#9331=ORIENTED_EDGE('',*,*,#7122,.T.);
#9332=ORIENTED_EDGE('',*,*,#7123,.T.);
#9333=ORIENTED_EDGE('',*,*,#7119,.F.);
#9334=ORIENTED_EDGE('',*,*,#7124,.T.);
#9335=ORIENTED_EDGE('',*,*,#7125,.T.);
#9336=ORIENTED_EDGE('',*,*,#7126,.T.);
#9337=ORIENTED_EDGE('',*,*,#7122,.F.);
#9338=ORIENTED_EDGE('',*,*,#7127,.T.);
#9339=ORIENTED_EDGE('',*,*,#7128,.T.);
#9340=ORIENTED_EDGE('',*,*,#7129,.T.);
#9341=ORIENTED_EDGE('',*,*,#7125,.F.);
#9342=ORIENTED_EDGE('',*,*,#7130,.T.);
#9343=ORIENTED_EDGE('',*,*,#7131,.T.);
#9344=ORIENTED_EDGE('',*,*,#7132,.T.);
#9345=ORIENTED_EDGE('',*,*,#7128,.F.);
#9346=ORIENTED_EDGE('',*,*,#7133,.T.);
#9347=ORIENTED_EDGE('',*,*,#7134,.F.);
#9348=ORIENTED_EDGE('',*,*,#7135,.T.);
#9349=ORIENTED_EDGE('',*,*,#7136,.F.);
#9350=ORIENTED_EDGE('',*,*,#7137,.T.);
#9351=ORIENTED_EDGE('',*,*,#7138,.T.);
#9352=ORIENTED_EDGE('',*,*,#7139,.T.);
#9353=ORIENTED_EDGE('',*,*,#7140,.F.);
#9354=ORIENTED_EDGE('',*,*,#7141,.F.);
#9355=ORIENTED_EDGE('',*,*,#7142,.T.);
#9356=ORIENTED_EDGE('',*,*,#7143,.T.);
#9357=ORIENTED_EDGE('',*,*,#7138,.F.);
#9358=ORIENTED_EDGE('',*,*,#7144,.F.);
#9359=ORIENTED_EDGE('',*,*,#7145,.T.);
#9360=ORIENTED_EDGE('',*,*,#7146,.T.);
#9361=ORIENTED_EDGE('',*,*,#7142,.F.);
#9362=ORIENTED_EDGE('',*,*,#7147,.F.);
#9363=ORIENTED_EDGE('',*,*,#7148,.T.);
#9364=ORIENTED_EDGE('',*,*,#7149,.T.);
#9365=ORIENTED_EDGE('',*,*,#7145,.F.);
#9366=ORIENTED_EDGE('',*,*,#7150,.F.);
#9367=ORIENTED_EDGE('',*,*,#7151,.T.);
#9368=ORIENTED_EDGE('',*,*,#7152,.T.);
#9369=ORIENTED_EDGE('',*,*,#7148,.F.);
#9370=ORIENTED_EDGE('',*,*,#7153,.F.);
#9371=ORIENTED_EDGE('',*,*,#7154,.T.);
#9372=ORIENTED_EDGE('',*,*,#7155,.T.);
#9373=ORIENTED_EDGE('',*,*,#7151,.F.);
#9374=ORIENTED_EDGE('',*,*,#7156,.F.);
#9375=ORIENTED_EDGE('',*,*,#7157,.T.);
#9376=ORIENTED_EDGE('',*,*,#7158,.T.);
#9377=ORIENTED_EDGE('',*,*,#7154,.F.);
#9378=ORIENTED_EDGE('',*,*,#7159,.F.);
#9379=ORIENTED_EDGE('',*,*,#7160,.F.);
#9380=ORIENTED_EDGE('',*,*,#7161,.F.);
#9381=ORIENTED_EDGE('',*,*,#7162,.F.);
#9382=ORIENTED_EDGE('',*,*,#7163,.T.);
#9383=ORIENTED_EDGE('',*,*,#7164,.T.);
#9384=ORIENTED_EDGE('',*,*,#7165,.T.);
#9385=ORIENTED_EDGE('',*,*,#7166,.F.);
#9386=ORIENTED_EDGE('',*,*,#7167,.F.);
#9387=ORIENTED_EDGE('',*,*,#7168,.T.);
#9388=ORIENTED_EDGE('',*,*,#7169,.T.);
#9389=ORIENTED_EDGE('',*,*,#7164,.F.);
#9390=ORIENTED_EDGE('',*,*,#7170,.F.);
#9391=ORIENTED_EDGE('',*,*,#7171,.T.);
#9392=ORIENTED_EDGE('',*,*,#7172,.T.);
#9393=ORIENTED_EDGE('',*,*,#7168,.F.);
#9394=ORIENTED_EDGE('',*,*,#7173,.F.);
#9395=ORIENTED_EDGE('',*,*,#7174,.T.);
#9396=ORIENTED_EDGE('',*,*,#7175,.T.);
#9397=ORIENTED_EDGE('',*,*,#7171,.F.);
#9398=ORIENTED_EDGE('',*,*,#7176,.F.);
#9399=ORIENTED_EDGE('',*,*,#7177,.T.);
#9400=ORIENTED_EDGE('',*,*,#7178,.T.);
#9401=ORIENTED_EDGE('',*,*,#7174,.F.);
#9402=ORIENTED_EDGE('',*,*,#7179,.F.);
#9403=ORIENTED_EDGE('',*,*,#7180,.T.);
#9404=ORIENTED_EDGE('',*,*,#7181,.T.);
#9405=ORIENTED_EDGE('',*,*,#7177,.F.);
#9406=ORIENTED_EDGE('',*,*,#7182,.F.);
#9407=ORIENTED_EDGE('',*,*,#7183,.T.);
#9408=ORIENTED_EDGE('',*,*,#7184,.T.);
#9409=ORIENTED_EDGE('',*,*,#7180,.F.);
#9410=ORIENTED_EDGE('',*,*,#7185,.F.);
#9411=ORIENTED_EDGE('',*,*,#7186,.F.);
#9412=ORIENTED_EDGE('',*,*,#7187,.F.);
#9413=ORIENTED_EDGE('',*,*,#7188,.F.);
#9414=ORIENTED_EDGE('',*,*,#7189,.T.);
#9415=ORIENTED_EDGE('',*,*,#7190,.T.);
#9416=ORIENTED_EDGE('',*,*,#7191,.T.);
#9417=ORIENTED_EDGE('',*,*,#7192,.F.);
#9418=ORIENTED_EDGE('',*,*,#7193,.F.);
#9419=ORIENTED_EDGE('',*,*,#7194,.T.);
#9420=ORIENTED_EDGE('',*,*,#7195,.T.);
#9421=ORIENTED_EDGE('',*,*,#7190,.F.);
#9422=ORIENTED_EDGE('',*,*,#7196,.F.);
#9423=ORIENTED_EDGE('',*,*,#7197,.T.);
#9424=ORIENTED_EDGE('',*,*,#7198,.T.);
#9425=ORIENTED_EDGE('',*,*,#7194,.F.);
#9426=ORIENTED_EDGE('',*,*,#7199,.F.);
#9427=ORIENTED_EDGE('',*,*,#7200,.T.);
#9428=ORIENTED_EDGE('',*,*,#7201,.T.);
#9429=ORIENTED_EDGE('',*,*,#7197,.F.);
#9430=ORIENTED_EDGE('',*,*,#7202,.F.);
#9431=ORIENTED_EDGE('',*,*,#7203,.T.);
#9432=ORIENTED_EDGE('',*,*,#7204,.T.);
#9433=ORIENTED_EDGE('',*,*,#7200,.F.);
#9434=ORIENTED_EDGE('',*,*,#7205,.F.);
#9435=ORIENTED_EDGE('',*,*,#7206,.T.);
#9436=ORIENTED_EDGE('',*,*,#7207,.T.);
#9437=ORIENTED_EDGE('',*,*,#7203,.F.);
#9438=ORIENTED_EDGE('',*,*,#7208,.F.);
#9439=ORIENTED_EDGE('',*,*,#7209,.T.);
#9440=ORIENTED_EDGE('',*,*,#7210,.T.);
#9441=ORIENTED_EDGE('',*,*,#7206,.F.);
#9442=ORIENTED_EDGE('',*,*,#7211,.F.);
#9443=ORIENTED_EDGE('',*,*,#7212,.F.);
#9444=ORIENTED_EDGE('',*,*,#7213,.F.);
#9445=ORIENTED_EDGE('',*,*,#7214,.F.);
#9446=ORIENTED_EDGE('',*,*,#7215,.T.);
#9447=ORIENTED_EDGE('',*,*,#7216,.T.);
#9448=ORIENTED_EDGE('',*,*,#7217,.T.);
#9449=ORIENTED_EDGE('',*,*,#7218,.F.);
#9450=ORIENTED_EDGE('',*,*,#7219,.F.);
#9451=ORIENTED_EDGE('',*,*,#7220,.T.);
#9452=ORIENTED_EDGE('',*,*,#7221,.T.);
#9453=ORIENTED_EDGE('',*,*,#7216,.F.);
#9454=ORIENTED_EDGE('',*,*,#7222,.F.);
#9455=ORIENTED_EDGE('',*,*,#7223,.T.);
#9456=ORIENTED_EDGE('',*,*,#7224,.T.);
#9457=ORIENTED_EDGE('',*,*,#7220,.F.);
#9458=ORIENTED_EDGE('',*,*,#7225,.F.);
#9459=ORIENTED_EDGE('',*,*,#7226,.T.);
#9460=ORIENTED_EDGE('',*,*,#7227,.T.);
#9461=ORIENTED_EDGE('',*,*,#7223,.F.);
#9462=ORIENTED_EDGE('',*,*,#7228,.F.);
#9463=ORIENTED_EDGE('',*,*,#7229,.T.);
#9464=ORIENTED_EDGE('',*,*,#7230,.T.);
#9465=ORIENTED_EDGE('',*,*,#7226,.F.);
#9466=ORIENTED_EDGE('',*,*,#7231,.F.);
#9467=ORIENTED_EDGE('',*,*,#7232,.T.);
#9468=ORIENTED_EDGE('',*,*,#7233,.T.);
#9469=ORIENTED_EDGE('',*,*,#7229,.F.);
#9470=ORIENTED_EDGE('',*,*,#7234,.F.);
#9471=ORIENTED_EDGE('',*,*,#7235,.T.);
#9472=ORIENTED_EDGE('',*,*,#7236,.T.);
#9473=ORIENTED_EDGE('',*,*,#7232,.F.);
#9474=ORIENTED_EDGE('',*,*,#7237,.F.);
#9475=ORIENTED_EDGE('',*,*,#7238,.F.);
#9476=ORIENTED_EDGE('',*,*,#7239,.F.);
#9477=ORIENTED_EDGE('',*,*,#7240,.F.);
#9478=ORIENTED_EDGE('',*,*,#7241,.T.);
#9479=ORIENTED_EDGE('',*,*,#7238,.T.);
#9480=ORIENTED_EDGE('',*,*,#7242,.T.);
#9481=ORIENTED_EDGE('',*,*,#7235,.F.);
#9482=ORIENTED_EDGE('',*,*,#7243,.F.);
#9483=ORIENTED_EDGE('',*,*,#7244,.F.);
#9484=ORIENTED_EDGE('',*,*,#7217,.F.);
#9485=ORIENTED_EDGE('',*,*,#7221,.F.);
#9486=ORIENTED_EDGE('',*,*,#7224,.F.);
#9487=ORIENTED_EDGE('',*,*,#7227,.F.);
#9488=ORIENTED_EDGE('',*,*,#7230,.F.);
#9489=ORIENTED_EDGE('',*,*,#7233,.F.);
#9490=ORIENTED_EDGE('',*,*,#7236,.F.);
#9491=ORIENTED_EDGE('',*,*,#7242,.F.);
#9492=ORIENTED_EDGE('',*,*,#7241,.F.);
#9493=ORIENTED_EDGE('',*,*,#7245,.F.);
#9494=ORIENTED_EDGE('',*,*,#7135,.F.);
#9495=ORIENTED_EDGE('',*,*,#7246,.F.);
#9496=ORIENTED_EDGE('',*,*,#7133,.F.);
#9497=ORIENTED_EDGE('',*,*,#7130,.F.);
#9498=ORIENTED_EDGE('',*,*,#7127,.F.);
#9499=ORIENTED_EDGE('',*,*,#7124,.F.);
#9500=ORIENTED_EDGE('',*,*,#7121,.F.);
#9501=ORIENTED_EDGE('',*,*,#7118,.F.);
#9502=ORIENTED_EDGE('',*,*,#7115,.F.);
#9503=ORIENTED_EDGE('',*,*,#7247,.F.);
#9504=ORIENTED_EDGE('',*,*,#7113,.F.);
#9505=ORIENTED_EDGE('',*,*,#7117,.F.);
#9506=ORIENTED_EDGE('',*,*,#7120,.F.);
#9507=ORIENTED_EDGE('',*,*,#7123,.F.);
#9508=ORIENTED_EDGE('',*,*,#7126,.F.);
#9509=ORIENTED_EDGE('',*,*,#7129,.F.);
#9510=ORIENTED_EDGE('',*,*,#7132,.F.);
#9511=ORIENTED_EDGE('',*,*,#7248,.F.);
#9512=ORIENTED_EDGE('',*,*,#7137,.F.);
#9513=ORIENTED_EDGE('',*,*,#7249,.F.);
#9514=ORIENTED_EDGE('',*,*,#7239,.T.);
#9515=ORIENTED_EDGE('',*,*,#7243,.T.);
#9516=ORIENTED_EDGE('',*,*,#7237,.T.);
#9517=ORIENTED_EDGE('',*,*,#7234,.T.);
#9518=ORIENTED_EDGE('',*,*,#7231,.T.);
#9519=ORIENTED_EDGE('',*,*,#7228,.T.);
#9520=ORIENTED_EDGE('',*,*,#7225,.T.);
#9521=ORIENTED_EDGE('',*,*,#7222,.T.);
#9522=ORIENTED_EDGE('',*,*,#7219,.T.);
#9523=ORIENTED_EDGE('',*,*,#7250,.T.);
#9524=ORIENTED_EDGE('',*,*,#7251,.T.);
#9525=ORIENTED_EDGE('',*,*,#7252,.T.);
#9526=ORIENTED_EDGE('',*,*,#7253,.T.);
#9527=ORIENTED_EDGE('',*,*,#7245,.T.);
#9528=ORIENTED_EDGE('',*,*,#7240,.T.);
#9529=ORIENTED_EDGE('',*,*,#7249,.T.);
#9530=ORIENTED_EDGE('',*,*,#7136,.T.);
#9531=ORIENTED_EDGE('',*,*,#7254,.T.);
#9532=ORIENTED_EDGE('',*,*,#7214,.T.);
#9533=ORIENTED_EDGE('',*,*,#7255,.T.);
#9534=ORIENTED_EDGE('',*,*,#7110,.T.);
#9535=ORIENTED_EDGE('',*,*,#7256,.T.);
#9536=ORIENTED_EDGE('',*,*,#7162,.T.);
#9537=ORIENTED_EDGE('',*,*,#7257,.T.);
#9538=ORIENTED_EDGE('',*,*,#7084,.T.);
#9539=ORIENTED_EDGE('',*,*,#7258,.T.);
#9540=ORIENTED_EDGE('',*,*,#7188,.T.);
#9541=ORIENTED_EDGE('',*,*,#7259,.T.);
#9542=ORIENTED_EDGE('',*,*,#7058,.T.);
#9543=ORIENTED_EDGE('',*,*,#7212,.T.);
#9544=ORIENTED_EDGE('',*,*,#7260,.T.);
#9545=ORIENTED_EDGE('',*,*,#7209,.F.);
#9546=ORIENTED_EDGE('',*,*,#7261,.F.);
#9547=ORIENTED_EDGE('',*,*,#7262,.F.);
#9548=ORIENTED_EDGE('',*,*,#7191,.F.);
#9549=ORIENTED_EDGE('',*,*,#7195,.F.);
#9550=ORIENTED_EDGE('',*,*,#7198,.F.);
#9551=ORIENTED_EDGE('',*,*,#7201,.F.);
#9552=ORIENTED_EDGE('',*,*,#7204,.F.);
#9553=ORIENTED_EDGE('',*,*,#7207,.F.);
#9554=ORIENTED_EDGE('',*,*,#7210,.F.);
#9555=ORIENTED_EDGE('',*,*,#7260,.F.);
#9556=ORIENTED_EDGE('',*,*,#7215,.F.);
#9557=ORIENTED_EDGE('',*,*,#7254,.F.);
#9558=ORIENTED_EDGE('',*,*,#7109,.F.);
#9559=ORIENTED_EDGE('',*,*,#7263,.F.);
#9560=ORIENTED_EDGE('',*,*,#7107,.F.);
#9561=ORIENTED_EDGE('',*,*,#7104,.F.);
#9562=ORIENTED_EDGE('',*,*,#7101,.F.);
#9563=ORIENTED_EDGE('',*,*,#7098,.F.);
#9564=ORIENTED_EDGE('',*,*,#7095,.F.);
#9565=ORIENTED_EDGE('',*,*,#7092,.F.);
#9566=ORIENTED_EDGE('',*,*,#7089,.F.);
#9567=ORIENTED_EDGE('',*,*,#7264,.F.);
#9568=ORIENTED_EDGE('',*,*,#7087,.F.);
#9569=ORIENTED_EDGE('',*,*,#7091,.F.);
#9570=ORIENTED_EDGE('',*,*,#7094,.F.);
#9571=ORIENTED_EDGE('',*,*,#7097,.F.);
#9572=ORIENTED_EDGE('',*,*,#7100,.F.);
#9573=ORIENTED_EDGE('',*,*,#7103,.F.);
#9574=ORIENTED_EDGE('',*,*,#7106,.F.);
#9575=ORIENTED_EDGE('',*,*,#7265,.F.);
#9576=ORIENTED_EDGE('',*,*,#7111,.F.);
#9577=ORIENTED_EDGE('',*,*,#7255,.F.);
#9578=ORIENTED_EDGE('',*,*,#7213,.T.);
#9579=ORIENTED_EDGE('',*,*,#7261,.T.);
#9580=ORIENTED_EDGE('',*,*,#7211,.T.);
#9581=ORIENTED_EDGE('',*,*,#7208,.T.);
#9582=ORIENTED_EDGE('',*,*,#7205,.T.);
#9583=ORIENTED_EDGE('',*,*,#7202,.T.);
#9584=ORIENTED_EDGE('',*,*,#7199,.T.);
#9585=ORIENTED_EDGE('',*,*,#7196,.T.);
#9586=ORIENTED_EDGE('',*,*,#7193,.T.);
#9587=ORIENTED_EDGE('',*,*,#7186,.T.);
#9588=ORIENTED_EDGE('',*,*,#7266,.T.);
#9589=ORIENTED_EDGE('',*,*,#7183,.F.);
#9590=ORIENTED_EDGE('',*,*,#7267,.F.);
#9591=ORIENTED_EDGE('',*,*,#7268,.F.);
#9592=ORIENTED_EDGE('',*,*,#7165,.F.);
#9593=ORIENTED_EDGE('',*,*,#7169,.F.);
#9594=ORIENTED_EDGE('',*,*,#7172,.F.);
#9595=ORIENTED_EDGE('',*,*,#7175,.F.);
#9596=ORIENTED_EDGE('',*,*,#7178,.F.);
#9597=ORIENTED_EDGE('',*,*,#7181,.F.);
#9598=ORIENTED_EDGE('',*,*,#7184,.F.);
#9599=ORIENTED_EDGE('',*,*,#7266,.F.);
#9600=ORIENTED_EDGE('',*,*,#7189,.F.);
#9601=ORIENTED_EDGE('',*,*,#7258,.F.);
#9602=ORIENTED_EDGE('',*,*,#7057,.F.);
#9603=ORIENTED_EDGE('',*,*,#7269,.F.);
#9604=ORIENTED_EDGE('',*,*,#7055,.F.);
#9605=ORIENTED_EDGE('',*,*,#7052,.F.);
#9606=ORIENTED_EDGE('',*,*,#7049,.F.);
#9607=ORIENTED_EDGE('',*,*,#7046,.F.);
#9608=ORIENTED_EDGE('',*,*,#7043,.F.);
#9609=ORIENTED_EDGE('',*,*,#7040,.F.);
#9610=ORIENTED_EDGE('',*,*,#7037,.F.);
#9611=ORIENTED_EDGE('',*,*,#7270,.F.);
#9612=ORIENTED_EDGE('',*,*,#7035,.F.);
#9613=ORIENTED_EDGE('',*,*,#7039,.F.);
#9614=ORIENTED_EDGE('',*,*,#7042,.F.);
#9615=ORIENTED_EDGE('',*,*,#7045,.F.);
#9616=ORIENTED_EDGE('',*,*,#7048,.F.);
#9617=ORIENTED_EDGE('',*,*,#7051,.F.);
#9618=ORIENTED_EDGE('',*,*,#7054,.F.);
#9619=ORIENTED_EDGE('',*,*,#7271,.F.);
#9620=ORIENTED_EDGE('',*,*,#7059,.F.);
#9621=ORIENTED_EDGE('',*,*,#7259,.F.);
#9622=ORIENTED_EDGE('',*,*,#7187,.T.);
#9623=ORIENTED_EDGE('',*,*,#7267,.T.);
#9624=ORIENTED_EDGE('',*,*,#7185,.T.);
#9625=ORIENTED_EDGE('',*,*,#7182,.T.);
#9626=ORIENTED_EDGE('',*,*,#7179,.T.);
#9627=ORIENTED_EDGE('',*,*,#7176,.T.);
#9628=ORIENTED_EDGE('',*,*,#7173,.T.);
#9629=ORIENTED_EDGE('',*,*,#7170,.T.);
#9630=ORIENTED_EDGE('',*,*,#7167,.T.);
#9631=ORIENTED_EDGE('',*,*,#7160,.T.);
#9632=ORIENTED_EDGE('',*,*,#7272,.T.);
#9633=ORIENTED_EDGE('',*,*,#7157,.F.);
#9634=ORIENTED_EDGE('',*,*,#7273,.F.);
#9635=ORIENTED_EDGE('',*,*,#7274,.F.);
#9636=ORIENTED_EDGE('',*,*,#7139,.F.);
#9637=ORIENTED_EDGE('',*,*,#7143,.F.);
#9638=ORIENTED_EDGE('',*,*,#7146,.F.);
#9639=ORIENTED_EDGE('',*,*,#7149,.F.);
#9640=ORIENTED_EDGE('',*,*,#7152,.F.);
#9641=ORIENTED_EDGE('',*,*,#7155,.F.);
#9642=ORIENTED_EDGE('',*,*,#7158,.F.);
#9643=ORIENTED_EDGE('',*,*,#7272,.F.);
#9644=ORIENTED_EDGE('',*,*,#7163,.F.);
#9645=ORIENTED_EDGE('',*,*,#7256,.F.);
#9646=ORIENTED_EDGE('',*,*,#7083,.F.);
#9647=ORIENTED_EDGE('',*,*,#7275,.F.);
#9648=ORIENTED_EDGE('',*,*,#7081,.F.);
#9649=ORIENTED_EDGE('',*,*,#7078,.F.);
#9650=ORIENTED_EDGE('',*,*,#7075,.F.);
#9651=ORIENTED_EDGE('',*,*,#7072,.F.);
#9652=ORIENTED_EDGE('',*,*,#7069,.F.);
#9653=ORIENTED_EDGE('',*,*,#7066,.F.);
#9654=ORIENTED_EDGE('',*,*,#7063,.F.);
#9655=ORIENTED_EDGE('',*,*,#7276,.F.);
#9656=ORIENTED_EDGE('',*,*,#7061,.F.);
#9657=ORIENTED_EDGE('',*,*,#7065,.F.);
#9658=ORIENTED_EDGE('',*,*,#7068,.F.);
#9659=ORIENTED_EDGE('',*,*,#7071,.F.);
#9660=ORIENTED_EDGE('',*,*,#7074,.F.);
#9661=ORIENTED_EDGE('',*,*,#7077,.F.);
#9662=ORIENTED_EDGE('',*,*,#7080,.F.);
#9663=ORIENTED_EDGE('',*,*,#7277,.F.);
#9664=ORIENTED_EDGE('',*,*,#7085,.F.);
#9665=ORIENTED_EDGE('',*,*,#7257,.F.);
#9666=ORIENTED_EDGE('',*,*,#7161,.T.);
#9667=ORIENTED_EDGE('',*,*,#7273,.T.);
#9668=ORIENTED_EDGE('',*,*,#7159,.T.);
#9669=ORIENTED_EDGE('',*,*,#7156,.T.);
#9670=ORIENTED_EDGE('',*,*,#7153,.T.);
#9671=ORIENTED_EDGE('',*,*,#7150,.T.);
#9672=ORIENTED_EDGE('',*,*,#7147,.T.);
#9673=ORIENTED_EDGE('',*,*,#7144,.T.);
#9674=ORIENTED_EDGE('',*,*,#7141,.T.);
#9675=ORIENTED_EDGE('',*,*,#7134,.T.);
#9676=ORIENTED_EDGE('',*,*,#7248,.T.);
#9677=ORIENTED_EDGE('',*,*,#7131,.F.);
#9678=ORIENTED_EDGE('',*,*,#7246,.T.);
#9679=ORIENTED_EDGE('',*,*,#7108,.T.);
#9680=ORIENTED_EDGE('',*,*,#7265,.T.);
#9681=ORIENTED_EDGE('',*,*,#7105,.F.);
#9682=ORIENTED_EDGE('',*,*,#7263,.T.);
#9683=ORIENTED_EDGE('',*,*,#7082,.T.);
#9684=ORIENTED_EDGE('',*,*,#7277,.T.);
#9685=ORIENTED_EDGE('',*,*,#7079,.F.);
#9686=ORIENTED_EDGE('',*,*,#7275,.T.);
#9687=ORIENTED_EDGE('',*,*,#7056,.T.);
#9688=ORIENTED_EDGE('',*,*,#7271,.T.);
#9689=ORIENTED_EDGE('',*,*,#7053,.F.);
#9690=ORIENTED_EDGE('',*,*,#7269,.T.);
#9691=ORIENTED_EDGE('',*,*,#7278,.T.);
#9692=ORIENTED_EDGE('',*,*,#7279,.T.);
#9693=ORIENTED_EDGE('',*,*,#7253,.F.);
#9694=ORIENTED_EDGE('',*,*,#7280,.F.);
#9695=ORIENTED_EDGE('',*,*,#7281,.T.);
#9696=ORIENTED_EDGE('',*,*,#7280,.T.);
#9697=ORIENTED_EDGE('',*,*,#7252,.F.);
#9698=ORIENTED_EDGE('',*,*,#7282,.F.);
#9699=ORIENTED_EDGE('',*,*,#7283,.T.);
#9700=ORIENTED_EDGE('',*,*,#7282,.T.);
#9701=ORIENTED_EDGE('',*,*,#7251,.F.);
#9702=ORIENTED_EDGE('',*,*,#7284,.F.);
#9703=ORIENTED_EDGE('',*,*,#7285,.T.);
#9704=ORIENTED_EDGE('',*,*,#7284,.T.);
#9705=ORIENTED_EDGE('',*,*,#7250,.F.);
#9706=ORIENTED_EDGE('',*,*,#7279,.F.);
#9707=ORIENTED_EDGE('',*,*,#7285,.F.);
#9708=ORIENTED_EDGE('',*,*,#7278,.F.);
#9709=ORIENTED_EDGE('',*,*,#7281,.F.);
#9710=ORIENTED_EDGE('',*,*,#7283,.F.);
#9711=ORIENTED_EDGE('',*,*,#7244,.T.);
#9712=ORIENTED_EDGE('',*,*,#7114,.T.);
#9713=ORIENTED_EDGE('',*,*,#7247,.T.);
#9714=ORIENTED_EDGE('',*,*,#7218,.T.);
#9715=ORIENTED_EDGE('',*,*,#7262,.T.);
#9716=ORIENTED_EDGE('',*,*,#7088,.T.);
#9717=ORIENTED_EDGE('',*,*,#7264,.T.);
#9718=ORIENTED_EDGE('',*,*,#7192,.T.);
#9719=ORIENTED_EDGE('',*,*,#7268,.T.);
#9720=ORIENTED_EDGE('',*,*,#7036,.T.);
#9721=ORIENTED_EDGE('',*,*,#7270,.T.);
#9722=ORIENTED_EDGE('',*,*,#7166,.T.);
#9723=ORIENTED_EDGE('',*,*,#7274,.T.);
#9724=ORIENTED_EDGE('',*,*,#7062,.T.);
#9725=ORIENTED_EDGE('',*,*,#7276,.T.);
#9726=ORIENTED_EDGE('',*,*,#7140,.T.);
#13429=PLANE('',#14608);
#13430=PLANE('',#14616);
#13431=PLANE('',#14617);
#13432=PLANE('',#14618);
#13433=PLANE('',#14619);
#13434=PLANE('',#14620);
#13569=ADVANCED_FACE('',(#2323),#1590,.F.);
#13570=ADVANCED_FACE('',(#2324),#1591,.F.);
#13571=ADVANCED_FACE('',(#2325),#1592,.F.);
#13572=ADVANCED_FACE('',(#2326),#1593,.F.);
#13573=ADVANCED_FACE('',(#2327),#1594,.F.);
#13574=ADVANCED_FACE('',(#2328),#1595,.F.);
#13575=ADVANCED_FACE('',(#2329),#1596,.F.);
#13576=ADVANCED_FACE('',(#2330),#1597,.F.);
#13577=ADVANCED_FACE('',(#2331),#1598,.F.);
#13578=ADVANCED_FACE('',(#2332),#1599,.F.);
#13579=ADVANCED_FACE('',(#2333),#1600,.F.);
#13580=ADVANCED_FACE('',(#2334),#1601,.F.);
#13581=ADVANCED_FACE('',(#2335),#1602,.F.);
#13582=ADVANCED_FACE('',(#2336),#1603,.F.);
#13583=ADVANCED_FACE('',(#2337),#1604,.F.);
#13584=ADVANCED_FACE('',(#2338),#1605,.F.);
#13585=ADVANCED_FACE('',(#2339),#1606,.F.);
#13586=ADVANCED_FACE('',(#2340),#1607,.F.);
#13587=ADVANCED_FACE('',(#2341),#1608,.F.);
#13588=ADVANCED_FACE('',(#2342),#1609,.F.);
#13589=ADVANCED_FACE('',(#2343),#1610,.F.);
#13590=ADVANCED_FACE('',(#2344),#1611,.F.);
#13591=ADVANCED_FACE('',(#2345),#1612,.F.);
#13592=ADVANCED_FACE('',(#2346),#1613,.F.);
#13593=ADVANCED_FACE('',(#2347),#1614,.F.);
#13594=ADVANCED_FACE('',(#2348),#1615,.F.);
#13595=ADVANCED_FACE('',(#2349),#1616,.F.);
#13596=ADVANCED_FACE('',(#2350),#1617,.F.);
#13597=ADVANCED_FACE('',(#2351),#1618,.F.);
#13598=ADVANCED_FACE('',(#2352),#1619,.F.);
#13599=ADVANCED_FACE('',(#2353),#1620,.F.);
#13600=ADVANCED_FACE('',(#2354),#1621,.F.);
#13601=ADVANCED_FACE('',(#2355),#1622,.F.);
#13602=ADVANCED_FACE('',(#2356),#1623,.F.);
#13603=ADVANCED_FACE('',(#2357),#1624,.F.);
#13604=ADVANCED_FACE('',(#2358),#1625,.F.);
#13605=ADVANCED_FACE('',(#2359),#1626,.F.);
#13606=ADVANCED_FACE('',(#2360),#1627,.F.);
#13607=ADVANCED_FACE('',(#2361),#1628,.F.);
#13608=ADVANCED_FACE('',(#2362),#1629,.F.);
#13609=ADVANCED_FACE('',(#2363),#1630,.F.);
#13610=ADVANCED_FACE('',(#2364),#1631,.F.);
#13611=ADVANCED_FACE('',(#2365),#1632,.F.);
#13612=ADVANCED_FACE('',(#2366),#1633,.F.);
#13613=ADVANCED_FACE('',(#2367),#1634,.F.);
#13614=ADVANCED_FACE('',(#2368),#1635,.F.);
#13615=ADVANCED_FACE('',(#2369),#1636,.F.);
#13616=ADVANCED_FACE('',(#2370),#1637,.F.);
#13617=ADVANCED_FACE('',(#2371),#1638,.F.);
#13618=ADVANCED_FACE('',(#2372),#1639,.F.);
#13619=ADVANCED_FACE('',(#2373),#1640,.F.);
#13620=ADVANCED_FACE('',(#2374),#1641,.F.);
#13621=ADVANCED_FACE('',(#2375),#1642,.F.);
#13622=ADVANCED_FACE('',(#2376),#1643,.F.);
#13623=ADVANCED_FACE('',(#2377),#1644,.F.);
#13624=ADVANCED_FACE('',(#2378),#1645,.F.);
#13625=ADVANCED_FACE('',(#2379),#1646,.F.);
#13626=ADVANCED_FACE('',(#2380),#1647,.F.);
#13627=ADVANCED_FACE('',(#2381),#1648,.F.);
#13628=ADVANCED_FACE('',(#2382),#1649,.F.);
#13629=ADVANCED_FACE('',(#2383),#1650,.F.);
#13630=ADVANCED_FACE('',(#2384),#1651,.F.);
#13631=ADVANCED_FACE('',(#2385),#1652,.F.);
#13632=ADVANCED_FACE('',(#2386),#1653,.F.);
#13633=ADVANCED_FACE('',(#2387),#1654,.F.);
#13634=ADVANCED_FACE('',(#2388),#257,.F.);
#13635=ADVANCED_FACE('',(#2389),#258,.F.);
#13636=ADVANCED_FACE('',(#2390,#2244,#2245,#2246,#2247),#13429,.T.);
#13637=ADVANCED_FACE('',(#2391),#1655,.F.);
#13638=ADVANCED_FACE('',(#2392),#259,.F.);
#13639=ADVANCED_FACE('',(#2393),#260,.F.);
#13640=ADVANCED_FACE('',(#2394),#1656,.F.);
#13641=ADVANCED_FACE('',(#2395),#261,.F.);
#13642=ADVANCED_FACE('',(#2396),#262,.F.);
#13643=ADVANCED_FACE('',(#2397),#1657,.F.);
#13644=ADVANCED_FACE('',(#2398),#263,.F.);
#13645=ADVANCED_FACE('',(#2399),#264,.F.);
#13646=ADVANCED_FACE('',(#2400),#1658,.F.);
#13647=ADVANCED_FACE('',(#2401),#1659,.F.);
#13648=ADVANCED_FACE('',(#2402),#1660,.F.);
#13649=ADVANCED_FACE('',(#2403),#1661,.F.);
#13650=ADVANCED_FACE('',(#2404),#13430,.T.);
#13651=ADVANCED_FACE('',(#2405),#13431,.T.);
#13652=ADVANCED_FACE('',(#2406),#13432,.T.);
#13653=ADVANCED_FACE('',(#2407),#13433,.T.);
#13654=ADVANCED_FACE('',(#2408,#2248,#2249,#2250,#2251),#13434,.F.);
#14311=CLOSED_SHELL('',(#13569,#13570,#13571,#13572,#13573,#13574,#13575,
#13576,#13577,#13578,#13579,#13580,#13581,#13582,#13583,#13584,#13585,#13586,
#13587,#13588,#13589,#13590,#13591,#13592,#13593,#13594,#13595,#13596,#13597,
#13598,#13599,#13600,#13601,#13602,#13603,#13604,#13605,#13606,#13607,#13608,
#13609,#13610,#13611,#13612,#13613,#13614,#13615,#13616,#13617,#13618,#13619,
#13620,#13621,#13622,#13623,#13624,#13625,#13626,#13627,#13628,#13629,#13630,
#13631,#13632,#13633,#13634,#13635,#13636,#13637,#13638,#13639,#13640,#13641,
#13642,#13643,#13644,#13645,#13646,#13647,#13648,#13649,#13650,#13651,#13652,
#13653,#13654));
#14526=AXIS2_PLACEMENT_3D('',#18481,#15611,#15612);
#14527=AXIS2_PLACEMENT_3D('',#18482,#15613,#15614);
#14528=AXIS2_PLACEMENT_3D('',#18492,#15616,#15617);
#14529=AXIS2_PLACEMENT_3D('',#18503,#15618,#15619);
#14530=AXIS2_PLACEMENT_3D('',#18554,#15621,#15622);
#14531=AXIS2_PLACEMENT_3D('',#18605,#15624,#15625);
#14532=AXIS2_PLACEMENT_3D('',#18653,#15627,#15628);
#14533=AXIS2_PLACEMENT_3D('',#18704,#15630,#15631);
#14534=AXIS2_PLACEMENT_3D('',#18755,#15633,#15634);
#14535=AXIS2_PLACEMENT_3D('',#18803,#15636,#15637);
#14536=AXIS2_PLACEMENT_3D('',#18822,#15639,#15640);
#14537=AXIS2_PLACEMENT_3D('',#18842,#15641,#15642);
#14538=AXIS2_PLACEMENT_3D('',#18852,#15644,#15645);
#14539=AXIS2_PLACEMENT_3D('',#18863,#15646,#15647);
#14540=AXIS2_PLACEMENT_3D('',#18914,#15649,#15650);
#14541=AXIS2_PLACEMENT_3D('',#18965,#15652,#15653);
#14542=AXIS2_PLACEMENT_3D('',#19013,#15655,#15656);
#14543=AXIS2_PLACEMENT_3D('',#19064,#15658,#15659);
#14544=AXIS2_PLACEMENT_3D('',#19115,#15661,#15662);
#14545=AXIS2_PLACEMENT_3D('',#19163,#15664,#15665);
#14546=AXIS2_PLACEMENT_3D('',#19182,#15667,#15668);
#14547=AXIS2_PLACEMENT_3D('',#19202,#15669,#15670);
#14548=AXIS2_PLACEMENT_3D('',#19212,#15672,#15673);
#14549=AXIS2_PLACEMENT_3D('',#19223,#15674,#15675);
#14550=AXIS2_PLACEMENT_3D('',#19274,#15677,#15678);
#14551=AXIS2_PLACEMENT_3D('',#19325,#15680,#15681);
#14552=AXIS2_PLACEMENT_3D('',#19373,#15683,#15684);
#14553=AXIS2_PLACEMENT_3D('',#19424,#15686,#15687);
#14554=AXIS2_PLACEMENT_3D('',#19475,#15689,#15690);
#14555=AXIS2_PLACEMENT_3D('',#19523,#15692,#15693);
#14556=AXIS2_PLACEMENT_3D('',#19542,#15695,#15696);
#14557=AXIS2_PLACEMENT_3D('',#19562,#15697,#15698);
#14558=AXIS2_PLACEMENT_3D('',#19572,#15700,#15701);
#14559=AXIS2_PLACEMENT_3D('',#19583,#15702,#15703);
#14560=AXIS2_PLACEMENT_3D('',#19634,#15705,#15706);
#14561=AXIS2_PLACEMENT_3D('',#19685,#15708,#15709);
#14562=AXIS2_PLACEMENT_3D('',#19733,#15711,#15712);
#14563=AXIS2_PLACEMENT_3D('',#19784,#15714,#15715);
#14564=AXIS2_PLACEMENT_3D('',#19835,#15717,#15718);
#14565=AXIS2_PLACEMENT_3D('',#19883,#15720,#15721);
#14566=AXIS2_PLACEMENT_3D('',#19902,#15723,#15724);
#14567=AXIS2_PLACEMENT_3D('',#19922,#15725,#15726);
#14568=AXIS2_PLACEMENT_3D('',#19936,#15728,#15729);
#14569=AXIS2_PLACEMENT_3D('',#19946,#15730,#15731);
#14570=AXIS2_PLACEMENT_3D('',#19970,#15733,#15734);
#14571=AXIS2_PLACEMENT_3D('',#19995,#15736,#15737);
#14572=AXIS2_PLACEMENT_3D('',#20020,#15739,#15740);
#14573=AXIS2_PLACEMENT_3D('',#20044,#15742,#15743);
#14574=AXIS2_PLACEMENT_3D('',#20069,#15745,#15746);
#14575=AXIS2_PLACEMENT_3D('',#20094,#15748,#15749);
#14576=AXIS2_PLACEMENT_3D('',#20105,#15751,#15752);
#14577=AXIS2_PLACEMENT_3D('',#20111,#15753,#15754);
#14578=AXIS2_PLACEMENT_3D('',#20125,#15756,#15757);
#14579=AXIS2_PLACEMENT_3D('',#20135,#15758,#15759);
#14580=AXIS2_PLACEMENT_3D('',#20159,#15761,#15762);
#14581=AXIS2_PLACEMENT_3D('',#20184,#15764,#15765);
#14582=AXIS2_PLACEMENT_3D('',#20209,#15767,#15768);
#14583=AXIS2_PLACEMENT_3D('',#20233,#15770,#15771);
#14584=AXIS2_PLACEMENT_3D('',#20258,#15773,#15774);
#14585=AXIS2_PLACEMENT_3D('',#20283,#15776,#15777);
#14586=AXIS2_PLACEMENT_3D('',#20294,#15779,#15780);
#14587=AXIS2_PLACEMENT_3D('',#20300,#15781,#15782);
#14588=AXIS2_PLACEMENT_3D('',#20314,#15784,#15785);
#14589=AXIS2_PLACEMENT_3D('',#20324,#15786,#15787);
#14590=AXIS2_PLACEMENT_3D('',#20348,#15789,#15790);
#14591=AXIS2_PLACEMENT_3D('',#20373,#15792,#15793);
#14592=AXIS2_PLACEMENT_3D('',#20398,#15795,#15796);
#14593=AXIS2_PLACEMENT_3D('',#20422,#15798,#15799);
#14594=AXIS2_PLACEMENT_3D('',#20447,#15801,#15802);
#14595=AXIS2_PLACEMENT_3D('',#20472,#15804,#15805);
#14596=AXIS2_PLACEMENT_3D('',#20483,#15807,#15808);
#14597=AXIS2_PLACEMENT_3D('',#20489,#15809,#15810);
#14598=AXIS2_PLACEMENT_3D('',#20503,#15812,#15813);
#14599=AXIS2_PLACEMENT_3D('',#20513,#15814,#15815);
#14600=AXIS2_PLACEMENT_3D('',#20537,#15817,#15818);
#14601=AXIS2_PLACEMENT_3D('',#20562,#15820,#15821);
#14602=AXIS2_PLACEMENT_3D('',#20587,#15823,#15824);
#14603=AXIS2_PLACEMENT_3D('',#20611,#15826,#15827);
#14604=AXIS2_PLACEMENT_3D('',#20636,#15829,#15830);
#14605=AXIS2_PLACEMENT_3D('',#20661,#15832,#15833);
#14606=AXIS2_PLACEMENT_3D('',#20672,#15835,#15836);
#14607=AXIS2_PLACEMENT_3D('',#20678,#15837,#15838);
#14608=AXIS2_PLACEMENT_3D('',#21580,#15839,#15840);
#14609=AXIS2_PLACEMENT_3D('',#22162,#15845,#15846);
#14610=AXIS2_PLACEMENT_3D('',#22873,#15847,#15848);
#14611=AXIS2_PLACEMENT_3D('',#23584,#15849,#15850);
#14612=AXIS2_PLACEMENT_3D('',#24295,#15851,#15852);
#14613=AXIS2_PLACEMENT_3D('',#24296,#15853,#15854);
#14614=AXIS2_PLACEMENT_3D('',#24297,#15855,#15856);
#14615=AXIS2_PLACEMENT_3D('',#24298,#15857,#15858);
#14616=AXIS2_PLACEMENT_3D('',#24299,#15859,#15860);
#14617=AXIS2_PLACEMENT_3D('',#24305,#15864,#15865);
#14618=AXIS2_PLACEMENT_3D('',#24309,#15868,#15869);
#14619=AXIS2_PLACEMENT_3D('',#24313,#15872,#15873);
#14620=AXIS2_PLACEMENT_3D('',#24315,#15875,#15876);
#15611=DIRECTION('axis',(0.,0.,1.));
#15612=DIRECTION('refdir',(1.,0.,0.));
#15613=DIRECTION('center_axis',(0.,0.,-1.));
#15614=DIRECTION('ref_axis',(-0.34687556303371,0.9379111598494,0.));
#15615=DIRECTION('',(0.,0.,-1.));
#15616=DIRECTION('center_axis',(0.,0.,-1.));
#15617=DIRECTION('ref_axis',(1.,0.,0.));
#15618=DIRECTION('center_axis',(0.,0.,-1.));
#15619=DIRECTION('ref_axis',(1.,0.,0.));
#15620=DIRECTION('',(0.,0.,-1.));
#15621=DIRECTION('center_axis',(0.,0.,-1.));
#15622=DIRECTION('ref_axis',(1.,0.,0.));
#15623=DIRECTION('',(0.,0.,-1.));
#15624=DIRECTION('center_axis',(0.,0.,-1.));
#15625=DIRECTION('ref_axis',(1.,0.,0.));
#15626=DIRECTION('',(0.,0.,-1.));
#15627=DIRECTION('center_axis',(0.,0.,-1.));
#15628=DIRECTION('ref_axis',(1.,0.,0.));
#15629=DIRECTION('',(0.,0.,-1.));
#15630=DIRECTION('center_axis',(0.,0.,-1.));
#15631=DIRECTION('ref_axis',(1.,0.,0.));
#15632=DIRECTION('',(0.,0.,-1.));
#15633=DIRECTION('center_axis',(0.,0.,-1.));
#15634=DIRECTION('ref_axis',(1.,0.,0.));
#15635=DIRECTION('',(0.,0.,-1.));
#15636=DIRECTION('center_axis',(0.,0.,-1.));
#15637=DIRECTION('ref_axis',(0.938001830644068,-0.346630301197656,0.));
#15638=DIRECTION('',(0.,0.,-1.));
#15639=DIRECTION('center_axis',(0.,0.,-1.));
#15640=DIRECTION('ref_axis',(1.,0.,0.));
#15641=DIRECTION('center_axis',(0.,0.,-1.));
#15642=DIRECTION('ref_axis',(-0.346875820911814,0.937911064476134,0.));
#15643=DIRECTION('',(0.,0.,-1.));
#15644=DIRECTION('center_axis',(0.,0.,-1.));
#15645=DIRECTION('ref_axis',(1.,0.,0.));
#15646=DIRECTION('center_axis',(0.,0.,-1.));
#15647=DIRECTION('ref_axis',(1.,0.,0.));
#15648=DIRECTION('',(0.,0.,-1.));
#15649=DIRECTION('center_axis',(0.,0.,-1.));
#15650=DIRECTION('ref_axis',(1.,0.,0.));
#15651=DIRECTION('',(0.,0.,-1.));
#15652=DIRECTION('center_axis',(0.,0.,-1.));
#15653=DIRECTION('ref_axis',(1.,0.,0.));
#15654=DIRECTION('',(0.,0.,-1.));
#15655=DIRECTION('center_axis',(0.,0.,-1.));
#15656=DIRECTION('ref_axis',(1.,0.,0.));
#15657=DIRECTION('',(0.,0.,-1.));
#15658=DIRECTION('center_axis',(0.,0.,-1.));
#15659=DIRECTION('ref_axis',(1.,0.,0.));
#15660=DIRECTION('',(0.,0.,-1.));
#15661=DIRECTION('center_axis',(0.,0.,-1.));
#15662=DIRECTION('ref_axis',(1.,0.,0.));
#15663=DIRECTION('',(0.,0.,-1.));
#15664=DIRECTION('center_axis',(0.,0.,-1.));
#15665=DIRECTION('ref_axis',(0.938001844837498,-0.346630262789403,0.));
#15666=DIRECTION('',(0.,0.,-1.));
#15667=DIRECTION('center_axis',(0.,0.,-1.));
#15668=DIRECTION('ref_axis',(1.,0.,0.));
#15669=DIRECTION('center_axis',(0.,0.,-1.));
#15670=DIRECTION('ref_axis',(-0.346875921807931,0.937911027160838,0.));
#15671=DIRECTION('',(0.,0.,-1.));
#15672=DIRECTION('center_axis',(0.,0.,-1.));
#15673=DIRECTION('ref_axis',(1.,0.,0.));
#15674=DIRECTION('center_axis',(0.,0.,-1.));
#15675=DIRECTION('ref_axis',(1.,0.,0.));
#15676=DIRECTION('',(0.,0.,-1.));
#15677=DIRECTION('center_axis',(0.,0.,-1.));
#15678=DIRECTION('ref_axis',(1.,0.,0.));
#15679=DIRECTION('',(0.,0.,-1.));
#15680=DIRECTION('center_axis',(0.,0.,-1.));
#15681=DIRECTION('ref_axis',(1.,0.,0.));
#15682=DIRECTION('',(0.,0.,-1.));
#15683=DIRECTION('center_axis',(0.,0.,-1.));
#15684=DIRECTION('ref_axis',(1.,0.,0.));
#15685=DIRECTION('',(0.,0.,-1.));
#15686=DIRECTION('center_axis',(0.,0.,-1.));
#15687=DIRECTION('ref_axis',(1.,0.,0.));
#15688=DIRECTION('',(0.,0.,-1.));
#15689=DIRECTION('center_axis',(0.,0.,-1.));
#15690=DIRECTION('ref_axis',(1.,0.,0.));
#15691=DIRECTION('',(0.,0.,-1.));
#15692=DIRECTION('center_axis',(0.,0.,-1.));
#15693=DIRECTION('ref_axis',(0.93800185687022,-0.346630230228148,0.));
#15694=DIRECTION('',(0.,0.,-1.));
#15695=DIRECTION('center_axis',(0.,0.,-1.));
#15696=DIRECTION('ref_axis',(1.,0.,0.));
#15697=DIRECTION('center_axis',(0.,0.,-1.));
#15698=DIRECTION('ref_axis',(-0.346875444642522,0.937911203634999,0.));
#15699=DIRECTION('',(0.,0.,-1.));
#15700=DIRECTION('center_axis',(0.,0.,-1.));
#15701=DIRECTION('ref_axis',(1.,0.,0.));
#15702=DIRECTION('center_axis',(0.,0.,-1.));
#15703=DIRECTION('ref_axis',(1.,0.,0.));
#15704=DIRECTION('',(0.,0.,-1.));
#15705=DIRECTION('center_axis',(0.,0.,-1.));
#15706=DIRECTION('ref_axis',(1.,0.,0.));
#15707=DIRECTION('',(0.,0.,-1.));
#15708=DIRECTION('center_axis',(0.,0.,-1.));
#15709=DIRECTION('ref_axis',(1.,0.,0.));
#15710=DIRECTION('',(0.,0.,-1.));
#15711=DIRECTION('center_axis',(0.,0.,-1.));
#15712=DIRECTION('ref_axis',(1.,0.,0.));
#15713=DIRECTION('',(0.,0.,-1.));
#15714=DIRECTION('center_axis',(0.,0.,-1.));
#15715=DIRECTION('ref_axis',(1.,0.,0.));
#15716=DIRECTION('',(0.,0.,-1.));
#15717=DIRECTION('center_axis',(0.,0.,-1.));
#15718=DIRECTION('ref_axis',(1.,0.,0.));
#15719=DIRECTION('',(0.,0.,-1.));
#15720=DIRECTION('center_axis',(0.,0.,-1.));
#15721=DIRECTION('ref_axis',(0.938001817986921,-0.346630335448631,0.));
#15722=DIRECTION('',(0.,0.,-1.));
#15723=DIRECTION('center_axis',(0.,0.,-1.));
#15724=DIRECTION('ref_axis',(1.,0.,0.));
#15725=DIRECTION('center_axis',(0.,0.,-1.));
#15726=DIRECTION('ref_axis',(0.793238775227928,0.608910704023913,0.));
#15727=DIRECTION('',(1.22464679914735E-16,-2.81870473344804E-30,-1.));
#15728=DIRECTION('center_axis',(0.,0.,1.));
#15729=DIRECTION('ref_axis',(1.,-2.28940061540476E-14,0.));
#15730=DIRECTION('center_axis',(0.,0.,-1.));
#15731=DIRECTION('ref_axis',(1.,-2.28940061540476E-14,0.));
#15732=DIRECTION('',(1.22464679914735E-16,-2.81870473344804E-30,-1.));
#15733=DIRECTION('center_axis',(0.,0.,-1.));
#15734=DIRECTION('ref_axis',(1.,-2.28940061540476E-14,0.));
#15735=DIRECTION('',(1.22464679914735E-16,-2.81870473344804E-30,-1.));
#15736=DIRECTION('center_axis',(0.,0.,-1.));
#15737=DIRECTION('ref_axis',(1.,-2.28940061540476E-14,0.));
#15738=DIRECTION('',(1.22464679914735E-16,-2.81870473344804E-30,-1.));
#15739=DIRECTION('center_axis',(0.,0.,-1.));
#15740=DIRECTION('ref_axis',(1.,-2.28940061540476E-14,0.));
#15741=DIRECTION('',(1.22464679914735E-16,-2.81870473344804E-30,-1.));
#15742=DIRECTION('center_axis',(0.,0.,-1.));
#15743=DIRECTION('ref_axis',(1.,-2.28940061540476E-14,0.));
#15744=DIRECTION('',(1.22464679914735E-16,-2.81870473344804E-30,-1.));
#15745=DIRECTION('center_axis',(0.,0.,-1.));
#15746=DIRECTION('ref_axis',(1.,-2.28940061540476E-14,0.));
#15747=DIRECTION('',(1.22464679914735E-16,-2.81870473344804E-30,-1.));
#15748=DIRECTION('center_axis',(0.,0.,-1.));
#15749=DIRECTION('ref_axis',(-0.609093973761813,-0.793098058960582,0.));
#15750=DIRECTION('',(1.22464679914735E-16,-2.81870473344804E-30,-1.));
#15751=DIRECTION('center_axis',(0.,0.,-1.));
#15752=DIRECTION('ref_axis',(1.,-2.28940061540476E-14,0.));
#15753=DIRECTION('center_axis',(0.,0.,-1.));
#15754=DIRECTION('ref_axis',(0.793238729919907,0.608910763047471,0.));
#15755=DIRECTION('',(1.22464679914735E-16,-2.551685006246E-30,-1.));
#15756=DIRECTION('center_axis',(0.,0.,1.));
#15757=DIRECTION('ref_axis',(1.,-2.07136246155669E-14,0.));
#15758=DIRECTION('center_axis',(0.,0.,-1.));
#15759=DIRECTION('ref_axis',(1.,-2.07136246155669E-14,0.));
#15760=DIRECTION('',(1.22464679914735E-16,-2.551685006246E-30,-1.));
#15761=DIRECTION('center_axis',(0.,0.,-1.));
#15762=DIRECTION('ref_axis',(1.,-2.07136246155669E-14,0.));
#15763=DIRECTION('',(1.22464679914735E-16,-2.551685006246E-30,-1.));
#15764=DIRECTION('center_axis',(0.,0.,-1.));
#15765=DIRECTION('ref_axis',(1.,-2.07136246155669E-14,0.));
#15766=DIRECTION('',(1.22464679914735E-16,-2.551685006246E-30,-1.));
#15767=DIRECTION('center_axis',(0.,0.,-1.));
#15768=DIRECTION('ref_axis',(1.,-2.07136246155669E-14,0.));
#15769=DIRECTION('',(1.22464679914735E-16,-2.551685006246E-30,-1.));
#15770=DIRECTION('center_axis',(0.,0.,-1.));
#15771=DIRECTION('ref_axis',(1.,-2.07136246155669E-14,0.));
#15772=DIRECTION('',(1.22464679914735E-16,-2.551685006246E-30,-1.));
#15773=DIRECTION('center_axis',(0.,0.,-1.));
#15774=DIRECTION('ref_axis',(1.,-2.07136246155669E-14,0.));
#15775=DIRECTION('',(1.22464679914735E-16,-2.551685006246E-30,-1.));
#15776=DIRECTION('center_axis',(0.,0.,-1.));
#15777=DIRECTION('ref_axis',(-0.609093922666122,-0.793098098201727,0.));
#15778=DIRECTION('',(1.22464679914735E-16,-2.551685006246E-30,-1.));
#15779=DIRECTION('center_axis',(0.,0.,-1.));
#15780=DIRECTION('ref_axis',(1.,-2.07136246155669E-14,0.));
#15781=DIRECTION('center_axis',(0.,0.,-1.));
#15782=DIRECTION('ref_axis',(0.793238788726965,0.608910686438477,0.));
#15783=DIRECTION('',(1.22464679914735E-16,-2.55168500624601E-30,-1.));
#15784=DIRECTION('center_axis',(0.,0.,1.));
#15785=DIRECTION('ref_axis',(1.,-2.0713624615567E-14,0.));
#15786=DIRECTION('center_axis',(0.,0.,-1.));
#15787=DIRECTION('ref_axis',(1.,-2.0713624615567E-14,0.));
#15788=DIRECTION('',(1.22464679914735E-16,-2.55168500624601E-30,-1.));
#15789=DIRECTION('center_axis',(0.,0.,-1.));
#15790=DIRECTION('ref_axis',(1.,-2.0713624615567E-14,0.));
#15791=DIRECTION('',(1.22464679914735E-16,-2.55168500624601E-30,-1.));
#15792=DIRECTION('center_axis',(0.,0.,-1.));
#15793=DIRECTION('ref_axis',(1.,-2.0713624615567E-14,0.));
#15794=DIRECTION('',(1.22464679914735E-16,-2.55168500624601E-30,-1.));
#15795=DIRECTION('center_axis',(0.,0.,-1.));
#15796=DIRECTION('ref_axis',(1.,-2.0713624615567E-14,0.));
#15797=DIRECTION('',(1.22464679914735E-16,-2.55168500624601E-30,-1.));
#15798=DIRECTION('center_axis',(0.,0.,-1.));
#15799=DIRECTION('ref_axis',(1.,-2.0713624615567E-14,0.));
#15800=DIRECTION('',(1.22464679914735E-16,-2.55168500624601E-30,-1.));
#15801=DIRECTION('center_axis',(0.,0.,-1.));
#15802=DIRECTION('ref_axis',(1.,-2.0713624615567E-14,0.));
#15803=DIRECTION('',(1.22464679914735E-16,-2.55168500624601E-30,-1.));
#15804=DIRECTION('center_axis',(0.,0.,-1.));
#15805=DIRECTION('ref_axis',(-0.609093953553475,-0.79309807448045,0.));
#15806=DIRECTION('',(1.22464679914735E-16,-2.55168500624601E-30,-1.));
#15807=DIRECTION('center_axis',(0.,0.,-1.));
#15808=DIRECTION('ref_axis',(1.,-2.0713624615567E-14,0.));
#15809=DIRECTION('center_axis',(0.,0.,-1.));
#15810=DIRECTION('ref_axis',(0.79323871288191,0.608910785243167,0.));
#15811=DIRECTION('',(1.22464679914735E-16,-2.55168500624601E-30,-1.));
#15812=DIRECTION('center_axis',(0.,0.,1.));
#15813=DIRECTION('ref_axis',(1.,-2.0713624615567E-14,0.));
#15814=DIRECTION('center_axis',(0.,0.,-1.));
#15815=DIRECTION('ref_axis',(1.,-2.0713624615567E-14,0.));
#15816=DIRECTION('',(1.22464679914735E-16,-2.55168500624601E-30,-1.));
#15817=DIRECTION('center_axis',(0.,0.,-1.));
#15818=DIRECTION('ref_axis',(1.,-2.0713624615567E-14,0.));
#15819=DIRECTION('',(1.22464679914735E-16,-2.55168500624601E-30,-1.));
#15820=DIRECTION('center_axis',(0.,0.,-1.));
#15821=DIRECTION('ref_axis',(1.,-2.0713624615567E-14,0.));
#15822=DIRECTION('',(1.22464679914735E-16,-2.55168500624601E-30,-1.));
#15823=DIRECTION('center_axis',(0.,0.,-1.));
#15824=DIRECTION('ref_axis',(1.,-2.0713624615567E-14,0.));
#15825=DIRECTION('',(1.22464679914735E-16,-2.55168500624601E-30,-1.));
#15826=DIRECTION('center_axis',(0.,0.,-1.));
#15827=DIRECTION('ref_axis',(1.,-2.0713624615567E-14,0.));
#15828=DIRECTION('',(1.22464679914735E-16,-2.55168500624601E-30,-1.));
#15829=DIRECTION('center_axis',(0.,0.,-1.));
#15830=DIRECTION('ref_axis',(1.,-2.0713624615567E-14,0.));
#15831=DIRECTION('',(1.22464679914735E-16,-2.55168500624601E-30,-1.));
#15832=DIRECTION('center_axis',(0.,0.,-1.));
#15833=DIRECTION('ref_axis',(-0.609093936537935,-0.793098087548269,0.));
#15834=DIRECTION('',(1.22464679914735E-16,-2.55168500624601E-30,-1.));
#15835=DIRECTION('center_axis',(0.,0.,-1.));
#15836=DIRECTION('ref_axis',(1.,-2.0713624615567E-14,0.));
#15837=DIRECTION('center_axis',(0.,0.,-1.));
#15838=DIRECTION('ref_axis',(1.,-2.0713624615567E-14,0.));
#15839=DIRECTION('center_axis',(0.,0.,1.));
#15840=DIRECTION('ref_axis',(1.,0.,0.));
#15841=DIRECTION('',(0.,-1.,0.));
#15842=DIRECTION('',(1.,0.,0.));
#15843=DIRECTION('',(0.,1.,0.));
#15844=DIRECTION('',(-1.,0.,0.));
#15845=DIRECTION('center_axis',(0.,0.,-1.));
#15846=DIRECTION('ref_axis',(1.,-2.0713624615567E-14,0.));
#15847=DIRECTION('center_axis',(0.,0.,-1.));
#15848=DIRECTION('ref_axis',(1.,-2.07136246155669E-14,0.));
#15849=DIRECTION('center_axis',(0.,0.,-1.));
#15850=DIRECTION('ref_axis',(1.,-2.28940061540476E-14,0.));
#15851=DIRECTION('center_axis',(0.,0.,-1.));
#15852=DIRECTION('ref_axis',(1.,0.,0.));
#15853=DIRECTION('center_axis',(0.,0.,-1.));
#15854=DIRECTION('ref_axis',(1.,0.,0.));
#15855=DIRECTION('center_axis',(0.,0.,-1.));
#15856=DIRECTION('ref_axis',(1.,0.,0.));
#15857=DIRECTION('center_axis',(0.,0.,-1.));
#15858=DIRECTION('ref_axis',(1.,0.,0.));
#15859=DIRECTION('center_axis',(0.,1.,0.));
#15860=DIRECTION('ref_axis',(-1.,0.,0.));
#15861=DIRECTION('',(-1.,0.,0.));
#15862=DIRECTION('',(0.,0.,1.));
#15863=DIRECTION('',(0.,0.,1.));
#15864=DIRECTION('center_axis',(1.,0.,0.));
#15865=DIRECTION('ref_axis',(0.,1.,0.));
#15866=DIRECTION('',(0.,1.,0.));
#15867=DIRECTION('',(0.,0.,1.));
#15868=DIRECTION('center_axis',(0.,-1.,0.));
#15869=DIRECTION('ref_axis',(1.,0.,0.));
#15870=DIRECTION('',(1.,0.,0.));
#15871=DIRECTION('',(0.,0.,1.));
#15872=DIRECTION('center_axis',(-1.,0.,0.));
#15873=DIRECTION('ref_axis',(0.,-1.,0.));
#15874=DIRECTION('',(0.,-1.,0.));
#15875=DIRECTION('center_axis',(0.,0.,1.));
#15876=DIRECTION('ref_axis',(1.,0.,0.));
#18481=CARTESIAN_POINT('',(0.,0.,0.));
#18482=CARTESIAN_POINT('Origin',(35.,35.,4.));
#18483=CARTESIAN_POINT('',(31.4879724201494,34.9998624352662,0.387416697508018));
#18484=CARTESIAN_POINT('',(31.4848003100606,34.9953496614248,0.112583302491981));
#18485=CARTESIAN_POINT('',(31.4825,35.,4.));
#18486=CARTESIAN_POINT('',(32.3264680662286,37.2858331630075,0.));
#18487=CARTESIAN_POINT('Ctrl Pts',(31.4848003100606,34.9953496614248,0.112583302491981));
#18488=CARTESIAN_POINT('Ctrl Pts',(31.491976688325,35.8232723665277,0.0750555349946529));
#18489=CARTESIAN_POINT('Ctrl Pts',(31.7874825103136,36.6554305951821,0.0375277674973252));
#18490=CARTESIAN_POINT('Ctrl Pts',(32.3264680662287,37.2858331630075,-2.22044604925031E-15));
#18491=CARTESIAN_POINT('',(37.6785012740241,37.2890246412443,7.00840805882243E-15));
#18492=CARTESIAN_POINT('Origin',(35.,35.,0.));
#18493=CARTESIAN_POINT('Ctrl Pts',(37.6785244495407,37.2890395253442,4.78783679369599E-15));
#18494=CARTESIAN_POINT('Ctrl Pts',(36.9607517209778,38.1233243316157,0.0499978774624456));
#18495=CARTESIAN_POINT('Ctrl Pts',(35.818670130213,38.598920544762,0.0999957549248864));
#18496=CARTESIAN_POINT('Ctrl Pts',(34.7217021974699,38.5118549254553,0.149993632387327));
#18497=CARTESIAN_POINT('Ctrl Pts',(33.5734927541699,38.4207223013458,0.202327008171411));
#18498=CARTESIAN_POINT('Ctrl Pts',(32.4747101009944,37.7131340510847,0.254660383955495));
#18499=CARTESIAN_POINT('Ctrl Pts',(31.9173289273845,36.7055535968161,0.306993759739579));
#18500=CARTESIAN_POINT('Ctrl Pts',(31.6318117612872,36.1894229315936,0.333801405662392));
#18501=CARTESIAN_POINT('Ctrl Pts',(31.4883570437126,35.5945750322157,0.360609051585205));
#18502=CARTESIAN_POINT('Ctrl Pts',(31.4879724201494,34.9998624352662,0.387416697508018));
#18503=CARTESIAN_POINT('Origin',(35.,35.,4.));
#18504=CARTESIAN_POINT('',(31.4787691259179,34.9978480355345,1.38741669750802));
#18505=CARTESIAN_POINT('',(31.4779837004207,35.0016823853973,1.11258330249198));
#18506=CARTESIAN_POINT('',(31.4825,35.,4.));
#18507=CARTESIAN_POINT('Ctrl Pts',(31.4779837004207,35.0016823853973,1.11258330249198));
#18508=CARTESIAN_POINT('Ctrl Pts',(31.4773936874682,35.1013890235937,1.10805583214991));
#18509=CARTESIAN_POINT('Ctrl Pts',(31.4812693590031,35.201048825548,1.10352836180784));
#18510=CARTESIAN_POINT('Ctrl Pts',(31.4897612702936,35.3003133216161,1.09900089146578));
#18511=CARTESIAN_POINT('Ctrl Pts',(31.5879199220602,36.4477192198909,1.04666751568169));
#18512=CARTESIAN_POINT('Ctrl Pts',(32.3028647460417,37.5423074099748,0.994334139897606));
#18513=CARTESIAN_POINT('Ctrl Pts',(33.3140597553874,38.0934397445863,0.942000764113521));
#18514=CARTESIAN_POINT('Ctrl Pts',(34.3252547647332,38.6445720791978,0.889667388329437));
#18515=CARTESIAN_POINT('Ctrl Pts',(35.632699959443,38.652248558337,0.837334012545353));
#18516=CARTESIAN_POINT('Ctrl Pts',(36.6501699298679,38.1127741860318,0.785000636761269));
#18517=CARTESIAN_POINT('Ctrl Pts',(37.6676399002927,37.5732998137267,0.732667260977184));
#18518=CARTESIAN_POINT('Ctrl Pts',(38.3951346464326,36.4866745899774,0.680333885193099));
#18519=CARTESIAN_POINT('Ctrl Pts',(38.5065308772508,35.3406022936711,0.628000509409014));
#18520=CARTESIAN_POINT('Ctrl Pts',(38.617927108069,34.1945299973649,0.57566713362493));
#18521=CARTESIAN_POINT('Ctrl Pts',(38.1132248235656,32.9890106285018,0.523333757840846));
#18522=CARTESIAN_POINT('Ctrl Pts',(37.2186051779362,32.2635143561234,0.471000382056762));
#18523=CARTESIAN_POINT('Ctrl Pts',(36.3239855323068,31.538018083745,0.418667006272677));
#18524=CARTESIAN_POINT('Ctrl Pts',(35.0394485255514,31.2925449078513,0.366333630488592));
#18525=CARTESIAN_POINT('Ctrl Pts',(33.9411234140671,31.6392615363868,0.314000254704508));
#18526=CARTESIAN_POINT('Ctrl Pts',(32.8427983025828,31.9859781649222,0.261666878920424));
#18527=CARTESIAN_POINT('Ctrl Pts',(31.9306850863697,32.9248845978868,0.20933350313634));
#18528=CARTESIAN_POINT('Ctrl Pts',(31.6136954419349,34.0300704557469,0.157000127352256));
#18529=CARTESIAN_POINT('Ctrl Pts',(31.5240160655112,34.3427380154138,0.142194519065497));
#18530=CARTESIAN_POINT('Ctrl Pts',(31.481969055963,34.6687142103727,0.127388910778739));
#18531=CARTESIAN_POINT('Ctrl Pts',(31.4848003100606,34.9953496614248,0.112583302491981));
#18532=CARTESIAN_POINT('Ctrl Pts',(31.4879724201494,34.9998624352662,0.387416697508018));
#18533=CARTESIAN_POINT('Ctrl Pts',(31.4876061889182,34.4335884275247,0.41294242736929));
#18534=CARTESIAN_POINT('Ctrl Pts',(31.6169542536305,33.8674370915364,0.438468157230561));
#18535=CARTESIAN_POINT('Ctrl Pts',(31.8768865080858,33.3694813094911,0.463993887091832));
#18536=CARTESIAN_POINT('Ctrl Pts',(32.4098049564414,32.3485621347107,0.516327262875917));
#18537=CARTESIAN_POINT('Ctrl Pts',(33.4916215471969,31.6142964434261,0.568660638660002));
#18538=CARTESIAN_POINT('Ctrl Pts',(34.6371338346999,31.4957027110504,0.620994014444087));
#18539=CARTESIAN_POINT('Ctrl Pts',(35.7826461222029,31.3771089786747,0.673327390228171));
#18540=CARTESIAN_POINT('Ctrl Pts',(36.9918541064533,31.8741872052079,0.725660766012256));
#18541=CARTESIAN_POINT('Ctrl Pts',(37.7226853676378,32.7641657941898,0.77799414179634));
#18542=CARTESIAN_POINT('Ctrl Pts',(38.4535166288223,33.6541443831717,0.830327517580425));
#18543=CARTESIAN_POINT('Ctrl Pts',(38.7059711669407,34.9370233346023,0.882660893364508));
#18544=CARTESIAN_POINT('Ctrl Pts',(38.3668191926393,36.0375701678912,0.934994269148593));
#18545=CARTESIAN_POINT('Ctrl Pts',(38.0276672183379,37.13811700118,0.987327644932677));
#18546=CARTESIAN_POINT('Ctrl Pts',(37.0969087316166,38.0563317163271,1.03966102071676));
#18547=CARTESIAN_POINT('Ctrl Pts',(35.9918739069821,38.3805519391724,1.09199439650085));
#18548=CARTESIAN_POINT('Ctrl Pts',(34.8868390823475,38.7047721620176,1.14432777228493));
#18549=CARTESIAN_POINT('Ctrl Pts',(33.6075279197997,38.4349978925611,1.19666114806902));
#18550=CARTESIAN_POINT('Ctrl Pts',(32.727515719297,37.6921720072953,1.2489945238531));
#18551=CARTESIAN_POINT('Ctrl Pts',(31.9516360834601,37.0372453176186,1.29513524840474));
#18552=CARTESIAN_POINT('Ctrl Pts',(31.4861477200874,36.0145964274628,1.34127597295638));
#18553=CARTESIAN_POINT('Ctrl Pts',(31.4787691259179,34.9978480355345,1.38741669750802));
#18554=CARTESIAN_POINT('Origin',(35.,35.,4.));
#18555=CARTESIAN_POINT('',(31.4830373600778,35.0030273041289,2.38741669750802));
#18556=CARTESIAN_POINT('',(31.4877387493273,35.0007919718047,2.11258330249198));
#18557=CARTESIAN_POINT('',(31.4825,35.,4.));
#18558=CARTESIAN_POINT('Ctrl Pts',(31.4877387493273,35.0007919718047,2.11258330249198));
#18559=CARTESIAN_POINT('Ctrl Pts',(31.4866495532798,35.5300199293211,2.08872275352109));
#18560=CARTESIAN_POINT('Ctrl Pts',(31.5990326814287,36.0588086783673,2.06486220455019));
#18561=CARTESIAN_POINT('Ctrl Pts',(31.8273024854561,36.5316518026084,2.0410016555793));
#18562=CARTESIAN_POINT('Ctrl Pts',(32.3279669692824,37.5687392953569,1.98866827979521));
#18563=CARTESIAN_POINT('Ctrl Pts',(33.3861125458452,38.3366963827873,1.93633490401113));
#18564=CARTESIAN_POINT('Ctrl Pts',(34.5273147643209,38.4912077048459,1.88400152822704));
#18565=CARTESIAN_POINT('Ctrl Pts',(35.6685169827965,38.6457190269045,1.83166815244296));
#18566=CARTESIAN_POINT('Ctrl Pts',(36.8927758431849,38.1867845835912,1.77933477665887));
#18567=CARTESIAN_POINT('Ctrl Pts',(37.6511886219643,37.3201660399649,1.72700140087479));
#18568=CARTESIAN_POINT('Ctrl Pts',(38.4096014007438,36.4535474963386,1.6746680250907));
#18569=CARTESIAN_POINT('Ctrl Pts',(38.7021680979142,35.1792448523993,1.62233464930662));
#18570=CARTESIAN_POINT('Ctrl Pts',(38.3977158188189,34.0686054522412,1.57000127352253));
#18571=CARTESIAN_POINT('Ctrl Pts',(38.0932635397237,32.9579660520831,1.51766789773845));
#18572=CARTESIAN_POINT('Ctrl Pts',(37.1917922843629,32.0109898957062,1.46533452195437));
#18573=CARTESIAN_POINT('Ctrl Pts',(36.0974794284194,31.6522428960312,1.41300114617028));
#18574=CARTESIAN_POINT('Ctrl Pts',(35.0031665724759,31.2934958963563,1.3606677703862));
#18575=CARTESIAN_POINT('Ctrl Pts',(33.7160121159498,31.5229780533832,1.30833439460211));
#18576=CARTESIAN_POINT('Ctrl Pts',(32.8131211274626,32.2378309351295,1.25600101881803));
#18577=CARTESIAN_POINT('Ctrl Pts',(31.9883411362357,32.8908403914793,1.20819511337601));
#18578=CARTESIAN_POINT('Ctrl Pts',(31.4842136922894,33.9488723706596,1.160389207934));
#18579=CARTESIAN_POINT('Ctrl Pts',(31.4779837004207,35.0016823853973,1.11258330249198));
#18580=CARTESIAN_POINT('Ctrl Pts',(31.4787691259179,34.9978480355345,1.38741669750802));
#18581=CARTESIAN_POINT('Ctrl Pts',(31.4777788280689,34.86138792912,1.39360934874046));
#18582=CARTESIAN_POINT('Ctrl Pts',(31.4850404305936,34.725034107982,1.39980199997291));
#18583=CARTESIAN_POINT('Ctrl Pts',(31.5009110513053,34.5896898261078,1.40599465120535));
#18584=CARTESIAN_POINT('Ctrl Pts',(31.6350318222736,33.445911031261,1.45832802698944));
#18585=CARTESIAN_POINT('Ctrl Pts',(32.3839866026675,32.3742309426426,1.51066140277352));
#18586=CARTESIAN_POINT('Ctrl Pts',(33.411975462032,31.855139584126,1.56299477855761));
#18587=CARTESIAN_POINT('Ctrl Pts',(34.4399643213965,31.3360482256093,1.61532815434169));
#18588=CARTESIAN_POINT('Ctrl Pts',(35.7469872597314,31.3695455971944,1.66766153012578));
#18589=CARTESIAN_POINT('Ctrl Pts',(36.7470354950296,31.9406144231743,1.71999490590986));
#18590=CARTESIAN_POINT('Ctrl Pts',(37.7470837303277,32.5116832491543,1.77232828169395));
#18591=CARTESIAN_POINT('Ctrl Pts',(38.4401572625891,33.620323529529,1.82466165747803));
#18592=CARTESIAN_POINT('Ctrl Pts',(38.5155126426898,34.7694703662421,1.87699503326212));
#18593=CARTESIAN_POINT('Ctrl Pts',(38.5908680227905,35.9186172029552,1.9293284090462));
#18594=CARTESIAN_POINT('Ctrl Pts',(38.0485052507305,37.1082705960066,1.98166178483028));
#18595=CARTESIAN_POINT('Ctrl Pts',(37.1315955779125,37.8050440926957,2.03399516061437));
#18596=CARTESIAN_POINT('Ctrl Pts',(36.2146859050945,38.5018175893848,2.08632853639845));
#18597=CARTESIAN_POINT('Ctrl Pts',(34.9232293315183,38.7057111897115,2.13866191218254));
#18598=CARTESIAN_POINT('Ctrl Pts',(33.836256457425,38.3253080449544,2.19099528796662));
#18599=CARTESIAN_POINT('Ctrl Pts',(32.7492835833317,37.9449049001973,2.24332866375071));
#18600=CARTESIAN_POINT('Ctrl Pts',(31.8667944087212,36.9802050103563,2.29566203953479));
#18601=CARTESIAN_POINT('Ctrl Pts',(31.5844572622636,35.8637362853384,2.34799541531888));
#18602=CARTESIAN_POINT('Ctrl Pts',(31.5135650119789,35.583401298313,2.36113584271526));
#18603=CARTESIAN_POINT('Ctrl Pts',(31.4805102901148,35.2934978064005,2.37427627011164));
#18604=CARTESIAN_POINT('Ctrl Pts',(31.4830373600778,35.0030273041289,2.38741669750802));
#18605=CARTESIAN_POINT('Origin',(35.,35.,4.));
#18606=CARTESIAN_POINT('',(31.4866348863052,34.9979909502101,3.38741669750802));
#18607=CARTESIAN_POINT('',(31.48047694743,34.9972296622465,3.11258330249198));
#18608=CARTESIAN_POINT('',(31.4825,35.,4.));
#18609=CARTESIAN_POINT('Ctrl Pts',(31.48047694743,34.9972296622465,3.11258330249198));
#18610=CARTESIAN_POINT('Ctrl Pts',(31.4887007318231,35.9502403897084,3.06938967489226));
#18611=CARTESIAN_POINT('Ctrl Pts',(31.8903810058125,36.9093635615769,3.02619604729254));
#18612=CARTESIAN_POINT('Ctrl Pts',(32.5815433671812,37.5618418521763,2.98300241969282));
#18613=CARTESIAN_POINT('Ctrl Pts',(33.4189553095288,38.352384195351,2.93066904390873));
#18614=CARTESIAN_POINT('Ctrl Pts',(34.6813192114488,38.6927800566904,2.87833566812465));
#18615=CARTESIAN_POINT('Ctrl Pts',(35.8026481651385,38.4304113471867,2.82600229234057));
#18616=CARTESIAN_POINT('Ctrl Pts',(36.9239771188282,38.1680426376829,2.77366891655648));
#18617=CARTESIAN_POINT('Ctrl Pts',(37.9042711242876,37.3029093573359,2.7213355407724));
#18618=CARTESIAN_POINT('Ctrl Pts',(38.3040106560533,36.2228981053939,2.66900216498831));
#18619=CARTESIAN_POINT('Ctrl Pts',(38.703750187819,35.1428868534519,2.61666878920423));
#18620=CARTESIAN_POINT('Ctrl Pts',(38.5229352458909,33.8479976299149,2.56433541342014));
#18621=CARTESIAN_POINT('Ctrl Pts',(37.8426350886114,32.9188003439573,2.51200203763606));
#18622=CARTESIAN_POINT('Ctrl Pts',(37.1623349313319,31.9896030579996,2.45966866185197));
#18623=CARTESIAN_POINT('Ctrl Pts',(35.9825495587008,31.4260977096214,2.40733528606789));
#18624=CARTESIAN_POINT('Ctrl Pts',(34.8322413779487,31.4809343941795,2.3550019102838));
#18625=CARTESIAN_POINT('Ctrl Pts',(33.6819331971966,31.5357710787376,2.30266853449972));
#18626=CARTESIAN_POINT('Ctrl Pts',(32.5611022083236,32.208949796232,2.25033515871564));
#18627=CARTESIAN_POINT('Ctrl Pts',(31.9722784094319,33.1986481040126,2.19800178293155));
#18628=CARTESIAN_POINT('Ctrl Pts',(31.6519192161228,33.7371096133752,2.16952895611836));
#18629=CARTESIAN_POINT('Ctrl Pts',(31.4890384885104,34.3692635020513,2.14105612930517));
#18630=CARTESIAN_POINT('Ctrl Pts',(31.4877387493273,35.0007919718047,2.11258330249198));
#18631=CARTESIAN_POINT('Ctrl Pts',(31.4830373600778,35.0030273041289,2.38741669750802));
#18632=CARTESIAN_POINT('Ctrl Pts',(31.4905746584961,34.1366631395343,2.42660964589572));
#18633=CARTESIAN_POINT('Ctrl Pts',(31.8146491184789,33.2652548262212,2.46580259428343));
#18634=CARTESIAN_POINT('Ctrl Pts',(32.3954080438652,32.6276439552295,2.50499554267113));
#18635=CARTESIAN_POINT('Ctrl Pts',(33.1708810902294,31.7762579103332,2.55732891845521));
#18636=CARTESIAN_POINT('Ctrl Pts',(34.4040123012624,31.3417233807355,2.6096622942393));
#18637=CARTESIAN_POINT('Ctrl Pts',(35.5419214016919,31.5188660285384,2.66199567002338));
#18638=CARTESIAN_POINT('Ctrl Pts',(36.6798305021214,31.6960086763413,2.71432904580747));
#18639=CARTESIAN_POINT('Ctrl Pts',(37.7225174919474,32.4848285015448,2.76666242159155));
#18640=CARTESIAN_POINT('Ctrl Pts',(38.2024886486778,33.5316543411059,2.81899579737563));
#18641=CARTESIAN_POINT('Ctrl Pts',(38.6824598054083,34.5784801806669,2.87132917315972));
#18642=CARTESIAN_POINT('Ctrl Pts',(38.5997151290432,35.8833120345855,2.9236625489438));
#18643=CARTESIAN_POINT('Ctrl Pts',(37.9913535966355,36.8611222874319,2.97599592472789));
#18644=CARTESIAN_POINT('Ctrl Pts',(37.3829920642279,37.8389325402782,3.02832930051197));
#18645=CARTESIAN_POINT('Ctrl Pts',(36.2490136757777,38.4897211920522,3.08066267629606));
#18646=CARTESIAN_POINT('Ctrl Pts',(35.0978430789634,38.5217040264218,3.13299605208014));
#18647=CARTESIAN_POINT('Ctrl Pts',(33.946672482149,38.5536868607913,3.18532942786423));
#18648=CARTESIAN_POINT('Ctrl Pts',(32.7783096769706,37.9668638777563,3.23766280364831));
#18649=CARTESIAN_POINT('Ctrl Pts',(32.1165957326192,37.0243399779266,3.2899961794324));
#18650=CARTESIAN_POINT('Ctrl Pts',(31.7059940575521,36.4394922573,3.3224696854576));
#18651=CARTESIAN_POINT('Ctrl Pts',(31.4904702191063,35.7176870288261,3.35494319148281));
#18652=CARTESIAN_POINT('Ctrl Pts',(31.4866348863052,34.9979909502101,3.38741669750802));
#18653=CARTESIAN_POINT('Origin',(35.,35.,4.));
#18654=CARTESIAN_POINT('',(31.4769533103746,34.9997936499005,4.38741669750802));
#18655=CARTESIAN_POINT('',(31.4811433043907,35.0029051520383,4.11258330249198));
#18656=CARTESIAN_POINT('',(31.4825,35.,4.));
#18657=CARTESIAN_POINT('Ctrl Pts',(31.4811433043907,35.0029051520383,4.11258330249198));
#18658=CARTESIAN_POINT('Ctrl Pts',(31.4791554024968,35.227917919132,4.10238997204752));
#18659=CARTESIAN_POINT('Ctrl Pts',(31.4989360215654,35.4525827818457,4.09219664160306));
#18660=CARTESIAN_POINT('Ctrl Pts',(31.5417697834626,35.6727628942377,4.08200331115859));
#18661=CARTESIAN_POINT('Ctrl Pts',(31.761681751374,36.8031852448886,4.02966993537451));
#18662=CARTESIAN_POINT('Ctrl Pts',(32.5892464227109,37.815395051703,3.97733655959042));
#18663=CARTESIAN_POINT('Ctrl Pts',(33.6534212074435,38.2555631921955,3.92500318380634));
#18664=CARTESIAN_POINT('Ctrl Pts',(34.7175959921761,38.6957313326879,3.87266980802225));
#18665=CARTESIAN_POINT('Ctrl Pts',(36.0183808903044,38.5638578068583,3.82033643223817));
#18666=CARTESIAN_POINT('Ctrl Pts',(36.9725627531969,37.9190687430238,3.76800305645409));
#18667=CARTESIAN_POINT('Ctrl Pts',(37.9267446160893,37.2742796791893,3.71566968067));
#18668=CARTESIAN_POINT('Ctrl Pts',(38.5343234437459,36.1165750773498,3.66333630488592));
#18669=CARTESIAN_POINT('Ctrl Pts',(38.5228883542836,34.965017348136,3.61100292910183));
#18670=CARTESIAN_POINT('Ctrl Pts',(38.5114532648213,33.8134596189221,3.55866955331775));
#18671=CARTESIAN_POINT('Ctrl Pts',(37.8810042582401,32.6680487623339,3.50633617753366));
#18672=CARTESIAN_POINT('Ctrl Pts',(36.9142061709404,32.0423352319303,3.45400280174958));
#18673=CARTESIAN_POINT('Ctrl Pts',(35.9474080836407,31.4166217015266,3.40166942596549));
#18674=CARTESIAN_POINT('Ctrl Pts',(34.6442609156224,31.3106054973076,3.34933605018141));
#18675=CARTESIAN_POINT('Ctrl Pts',(33.5890369502264,31.7718194895137,3.29700267439732));
#18676=CARTESIAN_POINT('Ctrl Pts',(32.5338129848304,32.2330334817198,3.24466929861324));
#18677=CARTESIAN_POINT('Ctrl Pts',(31.7265122220568,33.2614776703508,3.19233592282916));
#18678=CARTESIAN_POINT('Ctrl Pts',(31.5290918320576,34.3960441771713,3.14000254704507));
#18679=CARTESIAN_POINT('Ctrl Pts',(31.4946134017248,34.5941902362662,3.13086279886071));
#18680=CARTESIAN_POINT('Ctrl Pts',(31.4787367991106,34.7955731089531,3.12172305067635));
#18681=CARTESIAN_POINT('Ctrl Pts',(31.48047694743,34.9972296622465,3.11258330249198));
#18682=CARTESIAN_POINT('Ctrl Pts',(31.4866348863052,34.9979909502101,3.38741669750802));
#18683=CARTESIAN_POINT('Ctrl Pts',(31.4842893061927,34.5578453627213,3.4072765672669));
#18684=CARTESIAN_POINT('Ctrl Pts',(31.5611193891505,34.1184886387468,3.42713643702577));
#18685=CARTESIAN_POINT('Ctrl Pts',(31.7209246555095,33.7117308512332,3.44699630678465));
#18686=CARTESIAN_POINT('Ctrl Pts',(32.1420326062756,32.6398704409937,3.49932968256873));
#18687=CARTESIAN_POINT('Ctrl Pts',(33.1393135913321,31.7943744371391,3.55166305835282));
#18688=CARTESIAN_POINT('Ctrl Pts',(34.2656318975588,31.5543250290031,3.6039964341369));
#18689=CARTESIAN_POINT('Ctrl Pts',(35.3919502037855,31.3142756208671,3.65632980992098));
#18690=CARTESIAN_POINT('Ctrl Pts',(36.6473058311824,31.6796728084497,3.70866318570507));
#18691=CARTESIAN_POINT('Ctrl Pts',(37.4688540624077,32.4866890097577,3.76099656148916));
#18692=CARTESIAN_POINT('Ctrl Pts',(38.2904022936331,33.2937052110658,3.81332993727324));
#18693=CARTESIAN_POINT('Ctrl Pts',(38.6781431286869,34.5423404260991,3.86566331305732));
#18694=CARTESIAN_POINT('Ctrl Pts',(38.4582311043207,35.6727630669474,3.91799668884141));
#18695=CARTESIAN_POINT('Ctrl Pts',(38.2383190799545,36.8031857077956,3.97033006462549));
#18696=CARTESIAN_POINT('Ctrl Pts',(37.4107541961682,37.8153957744587,4.02266344040958));
#18697=CARTESIAN_POINT('Ctrl Pts',(36.3465791382448,38.2555640279499,4.07499681619366));
#18698=CARTESIAN_POINT('Ctrl Pts',(35.2824040803214,38.6957322814412,4.12733019197775));
#18699=CARTESIAN_POINT('Ctrl Pts',(33.9816188482609,38.5638587217606,4.17966356776183));
#18700=CARTESIAN_POINT('Ctrl Pts',(33.0274367404146,37.9190694923971,4.23199694354592));
#18701=CARTESIAN_POINT('Ctrl Pts',(32.0828594910996,37.2807707529301,4.28380352819995));
#18702=CARTESIAN_POINT('Ctrl Pts',(31.4779426270586,36.1398304565742,4.33561011285398));
#18703=CARTESIAN_POINT('Ctrl Pts',(31.4769533103746,34.9997936499005,4.38741669750802));
#18704=CARTESIAN_POINT('Origin',(35.,35.,4.));
#18705=CARTESIAN_POINT('',(31.4861926565527,35.0022702467704,5.38741669750802));
#18706=CARTESIAN_POINT('',(31.4875431178521,34.9988611670469,5.11258330249198));
#18707=CARTESIAN_POINT('',(31.4825,35.,4.));
#18708=CARTESIAN_POINT('Ctrl Pts',(31.4875431178521,34.9988611670469,5.11258330249198));
#18709=CARTESIAN_POINT('Ctrl Pts',(31.4894883427227,35.6536666001145,5.08305689341869));
#18710=CARTESIAN_POINT('Ctrl Pts',(31.6654106307538,36.3094429302072,5.0535304843454));
#18711=CARTESIAN_POINT('Ctrl Pts',(32.0086471712983,36.8611218096429,5.02400407527211));
#18712=CARTESIAN_POINT('Ctrl Pts',(32.6170085475347,37.8389318114614,4.97167069948803));
#18713=CARTESIAN_POINT('Ctrl Pts',(33.7509866448637,38.4897202961854,4.91933732370394));
#18714=CARTESIAN_POINT('Ctrl Pts',(34.9021569461515,38.5217031223488,4.86700394791986));
#18715=CARTESIAN_POINT('Ctrl Pts',(36.0533272474394,38.5536859485121,4.81467057213577));
#18716=CARTESIAN_POINT('Ctrl Pts',(37.2216897526861,37.9668631161147,4.76233719635169));
#18717=CARTESIAN_POINT('Ctrl Pts',(37.8834035271664,37.0243394582438,4.71000382056761));
#18718=CARTESIAN_POINT('Ctrl Pts',(38.5451173016466,36.0818158003729,4.65767044478352));
#18719=CARTESIAN_POINT('Ctrl Pts',(38.7001823453603,34.7835913170285,4.60533706899944));
#18720=CARTESIAN_POINT('Ctrl Pts',(38.2790745026986,33.7117311819539,4.55300369321535));
#18721=CARTESIAN_POINT('Ctrl Pts',(37.857966660037,32.6398710468792,4.50067031743127));
#18722=CARTESIAN_POINT('Ctrl Pts',(36.860685931,31.7943752600742,4.44833694164718));
#18723=CARTESIAN_POINT('Ctrl Pts',(35.7343679139176,31.5543259135622,4.3960035658631));
#18724=CARTESIAN_POINT('Ctrl Pts',(34.6080498968352,31.3142765670502,4.34367019007902));
#18725=CARTESIAN_POINT('Ctrl Pts',(33.3526945917074,31.6796736608312,4.29133681429493));
#18726=CARTESIAN_POINT('Ctrl Pts',(32.5311465713864,32.4866896549654,4.23900343851085));
#18727=CARTESIAN_POINT('Ctrl Pts',(31.8696170922289,33.1365176103207,4.19686339317123));
#18728=CARTESIAN_POINT('Ctrl Pts',(31.4893614502066,34.0726843317691,4.15472334783161));
#18729=CARTESIAN_POINT('Ctrl Pts',(31.4811433043907,35.0029051520383,4.11258330249198));
#18730=CARTESIAN_POINT('Ctrl Pts',(31.4769533103746,34.9997936499005,4.38741669750802));
#18731=CARTESIAN_POINT('Ctrl Pts',(31.4769432505867,34.9882012764272,4.38794348863807));
#18732=CARTESIAN_POINT('Ctrl Pts',(31.476995634958,34.9766089963718,4.38847027976812));
#18733=CARTESIAN_POINT('Ctrl Pts',(31.4771107413343,34.9650173391525,4.38899707089817));
#18734=CARTESIAN_POINT('Ctrl Pts',(31.4885458337323,33.8134593143178,4.44133044668225));
#18735=CARTESIAN_POINT('Ctrl Pts',(32.1189950021604,32.6680481636951,4.49366382246634));
#18736=CARTESIAN_POINT('Ctrl Pts',(33.0857933376524,32.0423344726558,4.54599719825042));
#18737=CARTESIAN_POINT('Ctrl Pts',(34.0525916731444,31.4166207816165,4.59833057403451));
#18738=CARTESIAN_POINT('Ctrl Pts',(35.3557391757004,31.3106045501606,4.65066394981859));
#18739=CARTESIAN_POINT('Ctrl Pts',(36.4109634119899,31.7718186607773,4.70299732560267));
#18740=CARTESIAN_POINT('Ctrl Pts',(37.4661876482795,32.233032771394,4.75533070138676));
#18741=CARTESIAN_POINT('Ctrl Pts',(38.2734886183026,33.2614772240832,4.80766407717084));
#18742=CARTESIAN_POINT('Ctrl Pts',(38.4709090589814,34.3960440221467,4.85999745295493));
#18743=CARTESIAN_POINT('Ctrl Pts',(38.6683294996601,35.5306108202102,4.91233082873901));
#18744=CARTESIAN_POINT('Ctrl Pts',(38.2558694109946,36.771299963648,4.9646642045231));
#18745=CARTESIAN_POINT('Ctrl Pts',(37.4184572536729,37.5618425098028,5.01699758030718));
#18746=CARTESIAN_POINT('Ctrl Pts',(36.5810450963513,38.3523850559575,5.06933095609127));
#18747=CARTESIAN_POINT('Ctrl Pts',(35.3186808703736,38.6927810048293,5.12166433187535));
#18748=CARTESIAN_POINT('Ctrl Pts',(34.1973516288142,38.4304122279041,5.17399770765944));
#18749=CARTESIAN_POINT('Ctrl Pts',(33.0760223872548,38.168043450979,5.22633108344352));
#18750=CARTESIAN_POINT('Ctrl Pts',(32.0957281301138,37.302909948257,5.2786644592276));
#18751=CARTESIAN_POINT('Ctrl Pts',(31.6959884957425,36.2228984191863,5.33099783501169));
#18752=CARTESIAN_POINT('Ctrl Pts',(31.5523398513352,35.834790313921,5.34980412251047));
#18753=CARTESIAN_POINT('Ctrl Pts',(31.4836619352111,35.4189336360054,5.36861041000924));
#18754=CARTESIAN_POINT('Ctrl Pts',(31.4861926565527,35.0022702467704,5.38741669750802));
#18755=CARTESIAN_POINT('Origin',(35.,35.,4.));
#18756=CARTESIAN_POINT('',(31.4836963557363,34.997016753135,6.38741669750802));
#18757=CARTESIAN_POINT('',(31.4775764275568,34.998690818207,6.11258330249198));
#18758=CARTESIAN_POINT('',(31.4825,35.,4.));
#18759=CARTESIAN_POINT('Ctrl Pts',(31.4775764275568,34.998690818207,6.11258330249198));
#18760=CARTESIAN_POINT('Ctrl Pts',(31.4827872982739,36.074383472183,6.06372381478987));
#18761=CARTESIAN_POINT('Ctrl Pts',(32.0123599558151,37.1545218488605,6.01486432708775));
#18762=CARTESIAN_POINT('Ctrl Pts',(32.8684049695572,37.8050433721304,5.96600483938563));
#18763=CARTESIAN_POINT('Ctrl Pts',(33.7853144071958,38.5018166895356,5.91367146360154));
#18764=CARTESIAN_POINT('Ctrl Pts',(35.0767706487491,38.7057102384231,5.86133808781746));
#18765=CARTESIAN_POINT('Ctrl Pts',(36.1637432436869,38.3253071915374,5.80900471203338));
#18766=CARTESIAN_POINT('Ctrl Pts',(37.2507158386246,37.9449041446517,5.75667133624929));
#18767=CARTESIAN_POINT('Ctrl Pts',(38.1332047869467,36.9802045019929,5.70433796046521));
#18768=CARTESIAN_POINT('Ctrl Pts',(38.4155418609846,35.8637360634774,5.65200458468113));
#18769=CARTESIAN_POINT('Ctrl Pts',(38.6978789350226,34.7472676249618,5.59967120889704));
#18770=CARTESIAN_POINT('Ctrl Pts',(38.3800641347763,33.4790303905896,5.54733783311296));
#18771=CARTESIAN_POINT('Ctrl Pts',(37.604591287456,32.6276445643168,5.49500445732887));
#18772=CARTESIAN_POINT('Ctrl Pts',(36.8291184401356,31.7762587380439,5.44267108154479));
#18773=CARTESIAN_POINT('Ctrl Pts',(35.595987545741,31.3417243198703,5.3903377057607));
#18774=CARTESIAN_POINT('Ctrl Pts',(34.4580787374483,31.5188669221671,5.33800432997662));
#18775=CARTESIAN_POINT('Ctrl Pts',(33.3201699291557,31.6960095244639,5.28567095419254));
#18776=CARTESIAN_POINT('Ctrl Pts',(32.277483206965,32.4848291472311,5.23333757840845));
#18777=CARTESIAN_POINT('Ctrl Pts',(31.7975121734416,33.5316547180712,5.18100420262437));
#18778=CARTESIAN_POINT('Ctrl Pts',(31.5883400491575,33.9878629329714,5.15819723591357));
#18779=CARTESIAN_POINT('Ctrl Pts',(31.4860405755429,34.4930724110572,5.13539026920278));
#18780=CARTESIAN_POINT('Ctrl Pts',(31.4875431178521,34.9988611670469,5.11258330249198));
#18781=CARTESIAN_POINT('Ctrl Pts',(31.4861926565527,35.0022702467704,5.38741669750802));
#18782=CARTESIAN_POINT('Ctrl Pts',(31.4907043241454,34.2594596183014,5.42094378579333));
#18783=CARTESIAN_POINT('Ctrl Pts',(31.7215335296905,33.5140850744687,5.45447087407864));
#18784=CARTESIAN_POINT('Ctrl Pts',(32.1573641816635,32.9187998099572,5.48799796236395));
#18785=CARTESIAN_POINT('Ctrl Pts',(32.8376645135573,31.9896022852182,5.54033133814803));
#18786=CARTESIAN_POINT('Ctrl Pts',(34.0174501889464,31.4260967911598,5.59266471393211));
#18787=CARTESIAN_POINT('Ctrl Pts',(35.1677586650642,31.4809334902507,5.64499808971619));
#18788=CARTESIAN_POINT('Ctrl Pts',(36.318067141182,31.5357701893416,5.69733146550028));
#18789=CARTESIAN_POINT('Ctrl Pts',(37.4388984180285,32.2089490815819,5.74966484128437));
#18790=CARTESIAN_POINT('Ctrl Pts',(38.027722367947,33.1986476425792,5.80199821706845));
#18791=CARTESIAN_POINT('Ctrl Pts',(38.6165463178655,34.1883462035765,5.85433159285254));
#18792=CARTESIAN_POINT('Ctrl Pts',(38.6733629408561,35.4945644333309,5.90666496863662));
#18793=CARTESIAN_POINT('Ctrl Pts',(38.1726983287836,36.5316521939121,5.9589983444207));
#18794=CARTESIAN_POINT('Ctrl Pts',(37.6720337167111,37.5687399544933,6.01133172020479));
#18795=CARTESIAN_POINT('Ctrl Pts',(36.6138878695757,38.3366972459014,6.06366509598887));
#18796=CARTESIAN_POINT('Ctrl Pts',(35.4726853575398,38.491208604665,6.11599847177296));
#18797=CARTESIAN_POINT('Ctrl Pts',(34.3314828455038,38.6457199634287,6.16833184755704));
#18798=CARTESIAN_POINT('Ctrl Pts',(33.1072236685675,38.1867853895479,6.22066522334113));
#18799=CARTESIAN_POINT('Ctrl Pts',(32.3488106963438,37.3201666288988,6.27299859912521));
#18800=CARTESIAN_POINT('Ctrl Pts',(31.7960966856348,36.6885947168973,6.31113796525281));
#18801=CARTESIAN_POINT('Ctrl Pts',(31.490801080199,35.8404951819918,6.34927733138042));
#18802=CARTESIAN_POINT('Ctrl Pts',(31.4836963557363,34.997016753135,6.38741669750802));
#18803=CARTESIAN_POINT('Origin',(35.,35.,4.));
#18804=CARTESIAN_POINT('',(31.47826034488,35.0017653187145,7.38741669750802));
#18805=CARTESIAN_POINT('',(31.4846882532079,35.0028111988253,7.11258330249198));
#18806=CARTESIAN_POINT('',(31.4825,35.,4.));
#18807=CARTESIAN_POINT('',(37.6735319337713,37.2858331630075,8.));
#18808=CARTESIAN_POINT('Ctrl Pts',(31.47826034488,35.0017653187145,7.38741669750802));
#18809=CARTESIAN_POINT('Ctrl Pts',(31.4849539836961,33.9623976729958,7.43461100431976));
#18810=CARTESIAN_POINT('Ctrl Pts',(31.9746240526108,32.9177662403339,7.4818053111315));
#18811=CARTESIAN_POINT('Ctrl Pts',(32.7813938443113,32.2635129435208,7.52899961794324));
#18812=CARTESIAN_POINT('Ctrl Pts',(33.6760141816485,31.5380168836533,7.58133299372733));
#18813=CARTESIAN_POINT('Ctrl Pts',(34.9605532865631,31.292545720314,7.63366636951141));
#18814=CARTESIAN_POINT('Ctrl Pts',(36.0588773921206,31.639261394405,7.68599974529549));
#18815=CARTESIAN_POINT('Ctrl Pts',(37.1572014976782,31.985977068496,7.73833312107957));
#18816=CARTESIAN_POINT('Ctrl Pts',(38.0693106038786,32.9248795800174,7.79066649686366));
#18817=CARTESIAN_POINT('Ctrl Pts',(38.3863002982481,34.0300657119841,7.84299987264775));
#18818=CARTESIAN_POINT('Ctrl Pts',(38.7032899926177,35.1352518439507,7.89533324843183));
#18819=CARTESIAN_POINT('Ctrl Pts',(38.4251602751564,36.4067215963626,7.94766662421592));
#18820=CARTESIAN_POINT('Ctrl Pts',(37.6735319337713,37.2858331630076,8.));
#18821=CARTESIAN_POINT('',(32.321499452735,37.2890251664065,7.99999999999999));
#18822=CARTESIAN_POINT('Origin',(35.,35.,8.));
#18823=CARTESIAN_POINT('Ctrl Pts',(32.321476328717,37.2890400220486,8.));
#18824=CARTESIAN_POINT('Ctrl Pts',(33.0392492598742,38.1233257780545,7.95000212253755));
#18825=CARTESIAN_POINT('Ctrl Pts',(34.1813302937714,38.5989193684354,7.90000424507511));
#18826=CARTESIAN_POINT('Ctrl Pts',(35.278297796919,38.5118532074872,7.85000636761267));
#18827=CARTESIAN_POINT('Ctrl Pts',(36.4265067905564,38.4207200164352,7.79767299182859));
#18828=CARTESIAN_POINT('Ctrl Pts',(37.5252891335093,37.7131334793234,7.74533961604451));
#18829=CARTESIAN_POINT('Ctrl Pts',(38.0826702008662,36.7055536192858,7.69300624026042));
#18830=CARTESIAN_POINT('Ctrl Pts',(38.6400512682231,35.6979737592483,7.64067286447634));
#18831=CARTESIAN_POINT('Ctrl Pts',(38.6560310599838,34.390400576285,7.58833948869225));
#18832=CARTESIAN_POINT('Ctrl Pts',(38.1231127521292,33.3694814726124,7.53600611290816));
#18833=CARTESIAN_POINT('Ctrl Pts',(37.5901944442746,32.3485623689397,7.48367273712408));
#18834=CARTESIAN_POINT('Ctrl Pts',(36.5083780368047,31.6142973445577,7.43133936134));
#18835=CARTESIAN_POINT('Ctrl Pts',(35.3628660305036,31.4957037502949,7.37900598555592));
#18836=CARTESIAN_POINT('Ctrl Pts',(34.2173540242026,31.3771101560321,7.32667260977183));
#18837=CARTESIAN_POINT('Ctrl Pts',(33.0081464190704,31.8741879918886,7.27433923398774));
#18838=CARTESIAN_POINT('Ctrl Pts',(32.2773153573829,32.7641662925145,7.22200585820366));
#18839=CARTESIAN_POINT('Ctrl Pts',(31.7679565185591,33.3844441344804,7.18553167296643));
#18840=CARTESIAN_POINT('Ctrl Pts',(31.4909695616634,34.1955737681155,7.14905748772921));
#18841=CARTESIAN_POINT('Ctrl Pts',(31.4846882532079,35.0028111988253,7.11258330249198));
#18842=CARTESIAN_POINT('Origin',(-35.,35.,4.));
#18843=CARTESIAN_POINT('',(-38.5120268522747,34.9998626667344,0.387416697508021));
#18844=CARTESIAN_POINT('',(-38.5151985683976,34.9953484440209,0.112583302491983));
#18845=CARTESIAN_POINT('',(-38.5175,35.,4.));
#18846=CARTESIAN_POINT('',(-37.6735319337713,37.2858331630075,0.));
#18847=CARTESIAN_POINT('Ctrl Pts',(-38.5151985683976,34.9953484440209,0.112583302491983));
#18848=CARTESIAN_POINT('Ctrl Pts',(-38.508022599206,35.8232716101844,0.0750555349946553));
#18849=CARTESIAN_POINT('Ctrl Pts',(-38.2125174896864,36.6554305951821,0.0375277674973274));
#18850=CARTESIAN_POINT('Ctrl Pts',(-37.6735319337713,37.2858331630075,0.));
#18851=CARTESIAN_POINT('',(-32.3214993158099,37.289025066123,6.74947782880687E-15));
#18852=CARTESIAN_POINT('Origin',(-35.,35.,0.));
#18853=CARTESIAN_POINT('Ctrl Pts',(-32.3214761820288,37.2890399271607,4.52762827229947E-15));
#18854=CARTESIAN_POINT('Ctrl Pts',(-33.0392490750158,38.123325504421,0.0499978774624455));
#18855=CARTESIAN_POINT('Ctrl Pts',(-34.1813302139117,38.5989195898449,0.0999957549248864));
#18856=CARTESIAN_POINT('Ctrl Pts',(-35.2782977979761,38.5118535311589,0.149993632387327));
#18857=CARTESIAN_POINT('Ctrl Pts',(-36.42650687631,38.420720447146,0.202327008171411));
#18858=CARTESIAN_POINT('Ctrl Pts',(-37.5252892775753,37.7131335867401,0.254660383955495));
#18859=CARTESIAN_POINT('Ctrl Pts',(-38.0826703648835,36.7055536147166,0.30699375973958));
#18860=CARTESIAN_POINT('Ctrl Pts',(-38.368187486773,36.189423196523,0.333801405662393));
#18861=CARTESIAN_POINT('Ctrl Pts',(-38.511642203595,35.5945753060192,0.360609051585207));
#18862=CARTESIAN_POINT('Ctrl Pts',(-38.5120268522747,34.9998626667344,0.387416697508021));
#18863=CARTESIAN_POINT('Origin',(-35.,35.,4.));
#18864=CARTESIAN_POINT('',(-38.5212301417031,34.9978480330234,1.38741669750802));
#18865=CARTESIAN_POINT('',(-38.5220165881118,35.0016823567161,1.11258330249198));
#18866=CARTESIAN_POINT('',(-38.5175,35.,4.));
#18867=CARTESIAN_POINT('Ctrl Pts',(-38.5220165881118,35.0016823567161,1.11258330249198));
#18868=CARTESIAN_POINT('Ctrl Pts',(-38.5226066014871,35.1013890040059,1.10805583214991));
#18869=CARTESIAN_POINT('Ctrl Pts',(-38.5187309301454,35.2010488154761,1.10352836180785));
#18870=CARTESIAN_POINT('Ctrl Pts',(-38.5102390188272,35.3003133215195,1.09900089146578));
#18871=CARTESIAN_POINT('Ctrl Pts',(-38.4120803667407,36.4477193350987,1.04666751568169));
#18872=CARTESIAN_POINT('Ctrl Pts',(-37.6971355129363,37.5423077018709,0.994334139897609));
#18873=CARTESIAN_POINT('Ctrl Pts',(-36.6859404016511,38.0934400513324,0.942000764113524));
#18874=CARTESIAN_POINT('Ctrl Pts',(-35.6747452903659,38.6445724007939,0.88966738832944));
#18875=CARTESIAN_POINT('Ctrl Pts',(-34.3672999215998,38.6522487329447,0.837334012545356));
#18876=CARTESIAN_POINT('Ctrl Pts',(-33.3498298999919,38.1127743676805,0.785000636761271));
#18877=CARTESIAN_POINT('Ctrl Pts',(-32.332359878384,37.5733000024162,0.732667260977186));
#18878=CARTESIAN_POINT('Ctrl Pts',(-31.6048652039344,36.4866749397369,0.680333885193101));
#18879=CARTESIAN_POINT('Ctrl Pts',(-31.4934688910568,35.3406024624848,0.628000509409016));
#18880=CARTESIAN_POINT('Ctrl Pts',(-31.3820725781792,34.1945299852327,0.575667133624932));
#18881=CARTESIAN_POINT('Ctrl Pts',(-31.8867746268736,32.9890100934079,0.523333757840848));
#18882=CARTESIAN_POINT('Ctrl Pts',(-32.7813945002955,32.26351389125,0.471000382056763));
#18883=CARTESIAN_POINT('Ctrl Pts',(-33.6760143737173,31.5380176890922,0.418667006272678));
#18884=CARTESIAN_POINT('Ctrl Pts',(-34.9605520718666,31.2925451766014,0.366333630488594));
#18885=CARTESIAN_POINT('Ctrl Pts',(-36.0588768524004,31.6392614911932,0.31400025470451));
#18886=CARTESIAN_POINT('Ctrl Pts',(-37.1572016329341,31.9859778057849,0.261666878920425));
#18887=CARTESIAN_POINT('Ctrl Pts',(-38.0693134958523,32.9248829474593,0.209333503136341));
#18888=CARTESIAN_POINT('Ctrl Pts',(-38.3863031564079,34.0300688951037,0.157000127352256));
#18889=CARTESIAN_POINT('Ctrl Pts',(-38.4759825373922,34.3427364801714,0.142194519065498));
#18890=CARTESIAN_POINT('Ctrl Pts',(-38.5180296611061,34.6687128110693,0.127388910778741));
#18891=CARTESIAN_POINT('Ctrl Pts',(-38.5151985683976,34.9953484440209,0.112583302491983));
#18892=CARTESIAN_POINT('Ctrl Pts',(-38.5120268522747,34.9998626667344,0.387416697508021));
#18893=CARTESIAN_POINT('Ctrl Pts',(-38.5123931074215,34.4335886186821,0.412942427369291));
#18894=CARTESIAN_POINT('Ctrl Pts',(-38.3830450900788,33.8674371959539,0.438468157230563));
#18895=CARTESIAN_POINT('Ctrl Pts',(-38.1231128912653,33.3694814421284,0.463993887091834));
#18896=CARTESIAN_POINT('Ctrl Pts',(-37.5901945569878,32.348562325205,0.516327262875918));
#18897=CARTESIAN_POINT('Ctrl Pts',(-36.5083781150815,31.6142971749993,0.568660638660002));
#18898=CARTESIAN_POINT('Ctrl Pts',(-35.3628660558844,31.4957035546786,0.620994014444087));
#18899=CARTESIAN_POINT('Ctrl Pts',(-34.2173539966873,31.3771099343579,0.673327390228171));
#18900=CARTESIAN_POINT('Ctrl Pts',(-33.0081463201995,31.8741878439222,0.725660766012255));
#18901=CARTESIAN_POINT('Ctrl Pts',(-32.2773152209783,32.7641661988384,0.77799414179634));
#18902=CARTESIAN_POINT('Ctrl Pts',(-31.5464841217571,33.6541445537545,0.830327517580424));
#18903=CARTESIAN_POINT('Ctrl Pts',(-31.2940295998026,34.9370233540225,0.882660893364509));
#18904=CARTESIAN_POINT('Ctrl Pts',(-31.6331814964185,36.0375699846378,0.934994269148593));
#18905=CARTESIAN_POINT('Ctrl Pts',(-31.9723333930344,37.1381166152532,0.987327644932678));
#18906=CARTESIAN_POINT('Ctrl Pts',(-32.9030917082208,38.0563310762161,1.03966102071676));
#18907=CARTESIAN_POINT('Ctrl Pts',(-34.0081263071124,38.3805512169411,1.09199439650085));
#18908=CARTESIAN_POINT('Ctrl Pts',(-35.1131609060039,38.7047713576661,1.14432777228493));
#18909=CARTESIAN_POINT('Ctrl Pts',(-36.3924717886008,38.4349971781534,1.19666114806902));
#18910=CARTESIAN_POINT('Ctrl Pts',(-37.2724838028734,37.6921714555696,1.2489945238531));
#18911=CARTESIAN_POINT('Ctrl Pts',(-38.0483632745171,37.0372449093246,1.29513524840474));
#18912=CARTESIAN_POINT('Ctrl Pts',(-38.5138515465497,36.0145962191428,1.34127597295638));
#18913=CARTESIAN_POINT('Ctrl Pts',(-38.5212301417031,34.9978480330234,1.38741669750802));
#18914=CARTESIAN_POINT('Origin',(-35.,35.,4.));
#18915=CARTESIAN_POINT('',(-38.516961906974,35.0030273033746,2.38741669750802));
#18916=CARTESIAN_POINT('',(-38.512261546942,35.0007919713519,2.11258330249198));
#18917=CARTESIAN_POINT('',(-38.5175,35.,4.));
#18918=CARTESIAN_POINT('Ctrl Pts',(-38.512261546942,35.0007919713519,2.11258330249198));
#18919=CARTESIAN_POINT('Ctrl Pts',(-38.513350743052,35.5300199732952,2.08872275352109));
#18920=CARTESIAN_POINT('Ctrl Pts',(-38.400967605409,36.0588087668393,2.06486220455019));
#18921=CARTESIAN_POINT('Ctrl Pts',(-38.1726977821637,36.5316519312173,2.0410016555793));
#18922=CARTESIAN_POINT('Ctrl Pts',(-37.6720332561867,37.568739511998,1.98866827979521));
#18923=CARTESIAN_POINT('Ctrl Pts',(-36.6138875906958,38.3366966664809,1.93633490401113));
#18924=CARTESIAN_POINT('Ctrl Pts',(-35.472685275733,38.4912080005995,1.88400152822705));
#18925=CARTESIAN_POINT('Ctrl Pts',(-34.3314829607702,38.6457193347182,1.83166815244296));
#18926=CARTESIAN_POINT('Ctrl Pts',(-33.1072239963354,38.1867848484726,1.77933477665888));
#18927=CARTESIAN_POINT('Ctrl Pts',(-32.3488111539779,37.3201662335233,1.72700140087479));
#18928=CARTESIAN_POINT('Ctrl Pts',(-31.5903983116205,36.453547618574,1.67466802509071));
#18929=CARTESIAN_POINT('Ctrl Pts',(-31.2978315913404,35.179244874921,1.62233464930662));
#18930=CARTESIAN_POINT('Ctrl Pts',(-31.6022838952552,34.0686053777681,1.57000127352254));
#18931=CARTESIAN_POINT('Ctrl Pts',(-31.90673619917,32.9579658806151,1.51766789773845));
#18932=CARTESIAN_POINT('Ctrl Pts',(-32.8082075272796,32.0109896299622,1.46533452195437));
#18933=CARTESIAN_POINT('Ctrl Pts',(-33.9025204773781,31.6522426059455,1.41300114617028));
#18934=CARTESIAN_POINT('Ctrl Pts',(-34.9968334274766,31.2934955819288,1.3606677703862));
#18935=CARTESIAN_POINT('Ctrl Pts',(-36.283987999564,31.5229777845482,1.30833439460212));
#18936=CARTESIAN_POINT('Ctrl Pts',(-37.1868790604233,32.2378307160511,1.25600101881803));
#18937=CARTESIAN_POINT('Ctrl Pts',(-38.0116591177612,32.8908402178529,1.20819511337602));
#18938=CARTESIAN_POINT('Ctrl Pts',(-38.5157865917788,33.94887224596,1.160389207934));
#18939=CARTESIAN_POINT('Ctrl Pts',(-38.5220165881118,35.0016823567161,1.11258330249198));
#18940=CARTESIAN_POINT('Ctrl Pts',(-38.5212301417031,34.9978480330234,1.38741669750802));
#18941=CARTESIAN_POINT('Ctrl Pts',(-38.5222204396842,34.8613879542309,1.39360934874046));
#18942=CARTESIAN_POINT('Ctrl Pts',(-38.5149588389545,34.7250341608202,1.39980199997291));
#18943=CARTESIAN_POINT('Ctrl Pts',(-38.499088221748,34.5896899066556,1.40599465120535));
#18944=CARTESIAN_POINT('Ctrl Pts',(-38.3649674804015,33.4459113459803,1.45832802698944));
#18945=CARTESIAN_POINT('Ctrl Pts',(-37.6160128517601,32.3742314902846,1.51066140277352));
#18946=CARTESIAN_POINT('Ctrl Pts',(-36.5880242056904,31.8551402422105,1.56299477855761));
#18947=CARTESIAN_POINT('Ctrl Pts',(-35.5600355596207,31.3360489941365,1.61532815434169));
#18948=CARTESIAN_POINT('Ctrl Pts',(-34.2530128961227,31.3695463536841,1.66766153012578));
#18949=CARTESIAN_POINT('Ctrl Pts',(-33.2529648698024,31.9406150594439,1.71999490590986));
#18950=CARTESIAN_POINT('Ctrl Pts',(-32.2529168434821,32.5116837652037,1.77232828169395));
#18951=CARTESIAN_POINT('Ctrl Pts',(-31.5598434543395,33.6203238171756,1.82466165747803));
#18952=CARTESIAN_POINT('Ctrl Pts',(-31.4844880896413,34.7694704150121,1.87699503326211));
#18953=CARTESIAN_POINT('Ctrl Pts',(-31.4091327249431,35.9186170128485,1.9293284090462));
#18954=CARTESIAN_POINT('Ctrl Pts',(-31.9514953846893,37.1082701565493,1.98166178483028));
#18955=CARTESIAN_POINT('Ctrl Pts',(-32.8684048665688,37.8050435076812,2.03399516061437));
#18956=CARTESIAN_POINT('Ctrl Pts',(-33.7853143484484,38.5018168588132,2.08632853639845));
#18957=CARTESIAN_POINT('Ctrl Pts',(-35.0767706524612,38.7057104173762,2.13866191218254));
#18958=CARTESIAN_POINT('Ctrl Pts',(-36.1637432999128,38.325307352079,2.19099528796662));
#18959=CARTESIAN_POINT('Ctrl Pts',(-37.2507159473644,37.9449042867818,2.24332866375071));
#18960=CARTESIAN_POINT('Ctrl Pts',(-38.1332049382548,36.9802045976245,2.29566203953479));
#18961=CARTESIAN_POINT('Ctrl Pts',(-38.4155420259161,35.8637361052132,2.34799541531887));
#18962=CARTESIAN_POINT('Ctrl Pts',(-38.4864342614375,35.5834011765932,2.36113584271526));
#18963=CARTESIAN_POINT('Ctrl Pts',(-38.5194889764144,35.2934977450987,2.37427627011164));
#18964=CARTESIAN_POINT('Ctrl Pts',(-38.516961906974,35.0030273033746,2.38741669750802));
#18965=CARTESIAN_POINT('Origin',(-35.,35.,4.));
#18966=CARTESIAN_POINT('',(-38.5133643814276,34.9979909506281,3.38741669750802));
#18967=CARTESIAN_POINT('',(-38.5195233495341,34.9972296620149,3.11258330249199));
#18968=CARTESIAN_POINT('',(-38.5175,35.,4.));
#18969=CARTESIAN_POINT('Ctrl Pts',(-38.5195233495341,34.9972296620149,3.11258330249199));
#18970=CARTESIAN_POINT('Ctrl Pts',(-38.5112995644464,35.9502404698791,3.06938967489226));
#18971=CARTESIAN_POINT('Ctrl Pts',(-38.1096192565637,36.9093637226591,3.02619604729254));
#18972=CARTESIAN_POINT('Ctrl Pts',(-37.4184568368782,37.5618420683218,2.98300241969282));
#18973=CARTESIAN_POINT('Ctrl Pts',(-36.581044823874,38.3523844782111,2.93066904390873));
#18974=CARTESIAN_POINT('Ctrl Pts',(-35.3186808154442,38.6927803683205,2.87833566812465));
#18975=CARTESIAN_POINT('Ctrl Pts',(-34.1973517671389,38.4304116366569,2.82600229234057));
#18976=CARTESIAN_POINT('Ctrl Pts',(-33.0760227188335,38.1680429049932,2.77366891655648));
#18977=CARTESIAN_POINT('Ctrl Pts',(-32.0957286306525,37.3029095515566,2.7213355407724));
#18978=CARTESIAN_POINT('Ctrl Pts',(-31.6959890651629,36.2228982085294,2.66900216498831));
#18979=CARTESIAN_POINT('Ctrl Pts',(-31.2962494996734,35.1428868655023,2.61666878920423));
#18980=CARTESIAN_POINT('Ctrl Pts',(-31.4770644568753,33.8479975328846,2.56433541342014));
#18981=CARTESIAN_POINT('Ctrl Pts',(-32.1573646715461,32.9188001684451,2.51200203763606));
#18982=CARTESIAN_POINT('Ctrl Pts',(-32.837664886217,31.9896028040056,2.45966866185197));
#18983=CARTESIAN_POINT('Ctrl Pts',(-34.0174503583568,31.4260974077442,2.40733528606789));
#18984=CARTESIAN_POINT('Ctrl Pts',(-35.1677586361884,31.4809340970796,2.3550019102838));
#18985=CARTESIAN_POINT('Ctrl Pts',(-36.3180669140201,31.535770786415,2.30266853449972));
#18986=CARTESIAN_POINT('Ctrl Pts',(-37.4388979975435,32.2089495613471,2.25033515871564));
#18987=CARTESIAN_POINT('Ctrl Pts',(-38.0277218460737,33.1986479523525,2.19800178293155));
#18988=CARTESIAN_POINT('Ctrl Pts',(-38.3480810663893,33.737109506995,2.16952895611836));
#18989=CARTESIAN_POINT('Ctrl Pts',(-38.5109618076844,34.3692634485841,2.14105612930517));
#18990=CARTESIAN_POINT('Ctrl Pts',(-38.512261546942,35.0007919713519,2.11258330249198));
#18991=CARTESIAN_POINT('Ctrl Pts',(-38.516961906974,35.0030273033746,2.38741669750802));
#18992=CARTESIAN_POINT('Ctrl Pts',(-38.5094246101142,34.1366633193706,2.42660964589572));
#18993=CARTESIAN_POINT('Ctrl Pts',(-38.1853502176079,33.2652551878002,2.46580259428343));
#18994=CARTESIAN_POINT('Ctrl Pts',(-37.6045914132455,32.6276444497373,2.50499554267113));
#18995=CARTESIAN_POINT('Ctrl Pts',(-36.8291185284818,31.7762585823377,2.55732891845521));
#18996=CARTESIAN_POINT('Ctrl Pts',(-35.5959875745222,31.3417241432036,2.6096622942393));
#18997=CARTESIAN_POINT('Ctrl Pts',(-34.4580787112737,31.5188667540608,2.66199567002338));
#18998=CARTESIAN_POINT('Ctrl Pts',(-33.3201698480253,31.6960093649181,2.71432904580747));
#18999=CARTESIAN_POINT('Ctrl Pts',(-32.277483075488,32.4848290257668,2.76666242159155));
#19000=CARTESIAN_POINT('Ctrl Pts',(-31.7975120187873,33.5316546471577,2.81899579737563));
#19001=CARTESIAN_POINT('Ctrl Pts',(-31.3175409620866,34.5784802685486,2.87132917315972));
#19002=CARTESIAN_POINT('Ctrl Pts',(-31.4002856212225,35.8833118504819,2.9236625489438));
#19003=CARTESIAN_POINT('Ctrl Pts',(-32.0086470268372,36.8611218995229,2.97599592472789));
#19004=CARTESIAN_POINT('Ctrl Pts',(-32.617008432452,37.8389319485639,3.02832930051197));
#19005=CARTESIAN_POINT('Ctrl Pts',(-33.7509865845457,38.4897204647128,3.08066267629606));
#19006=CARTESIAN_POINT('Ctrl Pts',(-34.902156941427,38.5217032924198,3.13299605208014));
#19007=CARTESIAN_POINT('Ctrl Pts',(-36.0533272983083,38.5536861201269,3.18532942786423));
#19008=CARTESIAN_POINT('Ctrl Pts',(-37.2216898599771,37.9668632593921,3.23766280364831));
#19009=CARTESIAN_POINT('Ctrl Pts',(-37.8834036664129,37.0243395560048,3.2899961794324));
#19010=CARTESIAN_POINT('Ctrl Pts',(-38.2940052559017,36.439491957273,3.3224696854576));
#19011=CARTESIAN_POINT('Ctrl Pts',(-38.5095290494265,35.7176868792413,3.35494319148281));
#19012=CARTESIAN_POINT('Ctrl Pts',(-38.5133643814276,34.9979909506281,3.38741669750802));
#19013=CARTESIAN_POINT('Origin',(-35.,35.,4.));
#19014=CARTESIAN_POINT('',(-38.5230459553398,34.9997936499459,4.38741669750802));
#19015=CARTESIAN_POINT('',(-38.5188569925171,35.0029051522836,4.11258330249198));
#19016=CARTESIAN_POINT('',(-38.5175,35.,4.));
#19017=CARTESIAN_POINT('Ctrl Pts',(-38.5188569925171,35.0029051522836,4.11258330249198));
#19018=CARTESIAN_POINT('Ctrl Pts',(-38.5208448945788,35.2279179383631,4.10238997204752));
#19019=CARTESIAN_POINT('Ctrl Pts',(-38.5010642738412,35.4525828200332,4.09219664160306));
#19020=CARTESIAN_POINT('Ctrl Pts',(-38.4582305083298,35.6727629510031,4.08200331115859));
#19021=CARTESIAN_POINT('Ctrl Pts',(-38.2383185218631,36.8031853970347,4.02966993537451));
#19022=CARTESIAN_POINT('Ctrl Pts',(-37.4107537806994,37.8153952892549,3.97733655959042));
#19023=CARTESIAN_POINT('Ctrl Pts',(-36.3465789061757,38.2555634668873,3.92500318380634));
#19024=CARTESIAN_POINT('Ctrl Pts',(-35.282404031652,38.6957316445196,3.87266980802226));
#19025=CARTESIAN_POINT('Ctrl Pts',(-33.9816190237685,38.5638581075641,3.82033643223817));
#19026=CARTESIAN_POINT('Ctrl Pts',(-33.0274370803658,37.9190689893243,3.76800305645409));
#19027=CARTESIAN_POINT('Ctrl Pts',(-32.0732551369631,37.2742798710845,3.71566968067));
#19028=CARTESIAN_POINT('Ctrl Pts',(-31.4656762580412,36.1165751715604,3.66333630488592));
#19029=CARTESIAN_POINT('Ctrl Pts',(-31.4771113484684,34.9650173451833,3.61100292910183));
#19030=CARTESIAN_POINT('Ctrl Pts',(-31.4885464388956,33.8134595188062,3.55866955331775));
#19031=CARTESIAN_POINT('Ctrl Pts',(-32.1189954986718,32.6680485655762,3.50633617753366));
#19032=CARTESIAN_POINT('Ctrl Pts',(-33.0857936675462,32.0423349823756,3.45400280174958));
#19033=CARTESIAN_POINT('Ctrl Pts',(-34.0525918364206,31.4166213991749,3.40166942596549));
#19034=CARTESIAN_POINT('Ctrl Pts',(-35.3557391143932,31.3106051860038,3.34933605018141));
#19035=CARTESIAN_POINT('Ctrl Pts',(-36.4109631688252,31.7718192171285,3.29700267439732));
#19036=CARTESIAN_POINT('Ctrl Pts',(-37.4661872232571,32.2330332482532,3.24466929861324));
#19037=CARTESIAN_POINT('Ctrl Pts',(-38.2734880541485,33.2614775236738,3.19233592282916));
#19038=CARTESIAN_POINT('Ctrl Pts',(-38.4709084608049,34.3960441262186,3.14000254704507));
#19039=CARTESIAN_POINT('Ctrl Pts',(-38.5053868940467,34.5941902020313,3.13086279886071));
#19040=CARTESIAN_POINT('Ctrl Pts',(-38.5212634980004,34.7955730917084,3.12172305067635));
#19041=CARTESIAN_POINT('Ctrl Pts',(-38.5195233495341,34.9972296620149,3.11258330249199));
#19042=CARTESIAN_POINT('Ctrl Pts',(-38.5133643814276,34.9979909506281,3.38741669750802));
#19043=CARTESIAN_POINT('Ctrl Pts',(-38.5157099610507,34.5578454548766,3.4072765672669));
#19044=CARTESIAN_POINT('Ctrl Pts',(-38.4388798941057,34.1184888224752,3.42713643702577));
#19045=CARTESIAN_POINT('Ctrl Pts',(-38.2790746610536,33.7117311197398,3.44699630678465));
#19046=CARTESIAN_POINT('Ctrl Pts',(-37.8579667980557,32.6398709329021,3.49932968256873));
#19047=CARTESIAN_POINT('Ctrl Pts',(-36.8606860208572,31.7943751052665,3.55166305835282));
#19048=CARTESIAN_POINT('Ctrl Pts',(-35.734367949382,31.554325747162,3.6039964341369));
#19049=CARTESIAN_POINT('Ctrl Pts',(-34.6080498779068,31.3142763890575,3.65632980992099));
#19050=CARTESIAN_POINT('Ctrl Pts',(-33.3526945121549,31.6796735004841,3.70866318570507));
#19051=CARTESIAN_POINT('Ctrl Pts',(-32.5311464521593,32.4866895335911,3.76099656148916));
#19052=CARTESIAN_POINT('Ctrl Pts',(-31.7095983921637,33.2937055666981,3.81332993727324));
#19053=CARTESIAN_POINT('Ctrl Pts',(-31.3218576379244,34.5423405214855,3.86566331305732));
#19054=CARTESIAN_POINT('Ctrl Pts',(-31.5417696164559,35.6727629267273,3.91799668884141));
#19055=CARTESIAN_POINT('Ctrl Pts',(-31.7616815949873,36.8031853319691,3.97033006462549));
#19056=CARTESIAN_POINT('Ctrl Pts',(-32.5892463062895,37.8153951876653,4.02266344040958));
#19057=CARTESIAN_POINT('Ctrl Pts',(-33.6534211424138,38.2555633494147,4.07499681619366));
#19058=CARTESIAN_POINT('Ctrl Pts',(-34.7175959785381,38.6957315111641,4.12733019197775));
#19059=CARTESIAN_POINT('Ctrl Pts',(-36.0183809394846,38.5638579789666,4.17966356776183));
#19060=CARTESIAN_POINT('Ctrl Pts',(-36.9725628484569,37.9190688839933,4.23199694354592));
#19061=CARTESIAN_POINT('Ctrl Pts',(-37.9171399008999,37.2807702775639,4.28380352819995));
#19062=CARTESIAN_POINT('Ctrl Pts',(-38.5220566388619,36.1398302190111,4.33561011285399));
#19063=CARTESIAN_POINT('Ctrl Pts',(-38.5230459553398,34.9997936499459,4.38741669750802));
#19064=CARTESIAN_POINT('Origin',(-35.,35.,4.));
#19065=CARTESIAN_POINT('',(-38.5138066110977,35.0022702462197,5.38741669750802));
#19066=CARTESIAN_POINT('',(-38.5124571785126,34.9988611669454,5.11258330249198));
#19067=CARTESIAN_POINT('',(-38.5175,35.,4.));
#19068=CARTESIAN_POINT('Ctrl Pts',(-38.5124571785126,34.9988611669454,5.11258330249198));
#19069=CARTESIAN_POINT('Ctrl Pts',(-38.5105119534794,35.6536666552656,5.08305689341869));
#19070=CARTESIAN_POINT('Ctrl Pts',(-38.3345896506072,36.3094430406945,5.0535304843454));
#19071=CARTESIAN_POINT('Ctrl Pts',(-37.9913530811025,36.8611219666803,5.02400407527211));
#19072=CARTESIAN_POINT('Ctrl Pts',(-37.3829916535365,37.8389320510055,4.97167069948803));
#19073=CARTESIAN_POINT('Ctrl Pts',(-36.2490134605232,38.4897205906347,4.91933732370395));
#19074=CARTESIAN_POINT('Ctrl Pts',(-35.0978430621031,38.5217034194952,4.86700394791986));
#19075=CARTESIAN_POINT('Ctrl Pts',(-33.946672663683,38.5536862483557,4.81467057213578));
#19076=CARTESIAN_POINT('Ctrl Pts',(-32.7783100598561,37.9668633664475,4.76233719635169));
#19077=CARTESIAN_POINT('Ctrl Pts',(-32.1165962295435,37.0243396290507,4.71000382056761));
#19078=CARTESIAN_POINT('Ctrl Pts',(-31.4548823992308,36.081815891654,4.65767044478352));
#19079=CARTESIAN_POINT('Ctrl Pts',(-31.2998173424323,34.7835912987687,4.60533706899944));
#19080=CARTESIAN_POINT('Ctrl Pts',(-31.7209252206252,33.7117310732541,4.55300369321535));
#19081=CARTESIAN_POINT('Ctrl Pts',(-32.1420330988181,32.6398708477396,4.50067031743127));
#19082=CARTESIAN_POINT('Ctrl Pts',(-33.1393139120024,31.7943749895958,4.44833694164718));
#19083=CARTESIAN_POINT('Ctrl Pts',(-34.2656320241194,31.5543256228295,4.3960035658631));
#19084=CARTESIAN_POINT('Ctrl Pts',(-35.3919501362363,31.3142762560632,4.34367019007901));
#19085=CARTESIAN_POINT('Ctrl Pts',(-36.647305547286,31.6796733806745,4.29133681429493));
#19086=CARTESIAN_POINT('Ctrl Pts',(-37.4688536369261,32.4866894429016,4.23900343851085));
#19087=CARTESIAN_POINT('Ctrl Pts',(-38.1303831719009,33.1365174530869,4.19686339317123));
#19088=CARTESIAN_POINT('Ctrl Pts',(-38.5106388460078,34.0726842535258,4.15472334783161));
#19089=CARTESIAN_POINT('Ctrl Pts',(-38.5188569925171,35.0029051522836,4.11258330249198));
#19090=CARTESIAN_POINT('Ctrl Pts',(-38.5230459553398,34.9997936499459,4.38741669750802));
#19091=CARTESIAN_POINT('Ctrl Pts',(-38.5230560151256,34.9882012788887,4.38794348863807));
#19092=CARTESIAN_POINT('Ctrl Pts',(-38.5230036307651,34.9766090012494,4.38847027976812));
#19093=CARTESIAN_POINT('Ctrl Pts',(-38.5228885244128,34.9650173464461,4.38899707089817));
#19094=CARTESIAN_POINT('Ctrl Pts',(-38.5114534343983,33.813459561621,4.44133044668225));
#19095=CARTESIAN_POINT('Ctrl Pts',(-37.881004397371,32.66804864972,4.49366382246634));
#19096=CARTESIAN_POINT('Ctrl Pts',(-36.9142062633822,32.0423350890982,4.54599719825042));
#19097=CARTESIAN_POINT('Ctrl Pts',(-35.9474081293934,31.4166215284763,4.59833057403451));
#19098=CARTESIAN_POINT('Ctrl Pts',(-34.6442608984431,31.3106053191336,4.65066394981859));
#19099=CARTESIAN_POINT('Ctrl Pts',(-33.5890368820876,31.7718193336147,4.70299732560267));
#19100=CARTESIAN_POINT('Ctrl Pts',(-32.533812865732,32.2330333480957,4.75533070138676));
#19101=CARTESIAN_POINT('Ctrl Pts',(-31.7265120639713,33.2614775864005,4.80766407717084));
#19102=CARTESIAN_POINT('Ctrl Pts',(-31.5290916644384,34.3960441480086,4.85999745295493));
#19103=CARTESIAN_POINT('Ctrl Pts',(-31.3316712649055,35.5306107096167,4.91233082873901));
#19104=CARTESIAN_POINT('Ctrl Pts',(-31.7441312676005,36.771299594528,4.9646642045231));
#19105=CARTESIAN_POINT('Ctrl Pts',(-32.5815432503882,37.5618419758867,5.01699758030718));
#19106=CARTESIAN_POINT('Ctrl Pts',(-33.418955233176,38.3523843572453,5.06933095609127));
#19107=CARTESIAN_POINT('Ctrl Pts',(-34.6813191960565,38.6927802350512,5.12166433187535));
#19108=CARTESIAN_POINT('Ctrl Pts',(-35.8026482038993,38.4304115128643,5.17399770765944));
#19109=CARTESIAN_POINT('Ctrl Pts',(-36.9239772117421,38.1680427906774,5.22633108344352));
#19110=CARTESIAN_POINT('Ctrl Pts',(-37.9042712645471,37.3029094684976,5.2786644592276));
#19111=CARTESIAN_POINT('Ctrl Pts',(-38.3040108156146,36.2228981644233,5.33099783501169));
#19112=CARTESIAN_POINT('Ctrl Pts',(-38.4476594300862,35.8347901400117,5.34980412251047));
#19113=CARTESIAN_POINT('Ctrl Pts',(-38.5163373319043,35.4189335486904,5.36861041000924));
#19114=CARTESIAN_POINT('Ctrl Pts',(-38.5138066110977,35.0022702462197,5.38741669750802));
#19115=CARTESIAN_POINT('Origin',(-35.,35.,4.));
#19116=CARTESIAN_POINT('',(-38.5163029138352,34.997016742257,6.38741669750802));
#19117=CARTESIAN_POINT('',(-38.5224238694764,34.9986908177615,6.11258330249199));
#19118=CARTESIAN_POINT('',(-38.5175,35.,4.));
#19119=CARTESIAN_POINT('Ctrl Pts',(-38.5224238694764,34.9986908177615,6.11258330249199));
#19120=CARTESIAN_POINT('Ctrl Pts',(-38.5172129982537,36.0743835623573,6.06372381478987));
#19121=CARTESIAN_POINT('Ctrl Pts',(-37.9876402962914,37.154522030678,6.01486432708775));
#19122=CARTESIAN_POINT('Ctrl Pts',(-37.1315952103829,37.8050436089632,5.96600483938563));
#19123=CARTESIAN_POINT('Ctrl Pts',(-36.2146856954469,38.5018169852953,5.91367146360155));
#19124=CARTESIAN_POINT('Ctrl Pts',(-34.9232293447652,38.705710551088,5.86133808781746));
#19125=CARTESIAN_POINT('Ctrl Pts',(-33.8362566580758,38.325307472034,5.80900471203338));
#19126=CARTESIAN_POINT('Ctrl Pts',(-32.7492839713864,37.9449043929801,5.75667133624929));
#19127=CARTESIAN_POINT('Ctrl Pts',(-31.8667949486893,36.9802046690794,5.70433796046521));
#19128=CARTESIAN_POINT('Ctrl Pts',(-31.5844578508488,35.8637361363978,5.65200458468113));
#19129=CARTESIAN_POINT('Ctrl Pts',(-31.3021207530084,34.7472676037162,5.59967120889704));
#19130=CARTESIAN_POINT('Ctrl Pts',(-31.6199355800247,33.4790302622538,5.54733783311296));
#19131=CARTESIAN_POINT('Ctrl Pts',(-32.3954084927658,32.6276443641247,5.49500445732887));
#19132=CARTESIAN_POINT('Ctrl Pts',(-33.1708814055069,31.7762584659956,5.44267108154479));
#19133=CARTESIAN_POINT('Ctrl Pts',(-34.4040124039728,31.3417240112,5.39033770576071));
#19134=CARTESIAN_POINT('Ctrl Pts',(-35.5419213082836,31.5188666284535,5.33800432997662));
#19135=CARTESIAN_POINT('Ctrl Pts',(-36.6798302125945,31.6960092457071,5.28567095419254));
#19136=CARTESIAN_POINT('Ctrl Pts',(-37.7225170227502,32.4848289350099,5.23333757840845));
#19137=CARTESIAN_POINT('Ctrl Pts',(-38.2024880967687,33.5316545941719,5.18100420262437));
#19138=CARTESIAN_POINT('Ctrl Pts',(-38.4116602387006,33.987862847563,5.15819723591357));
#19139=CARTESIAN_POINT('Ctrl Pts',(-38.5139597209473,34.4930723682773,5.13539026920278));
#19140=CARTESIAN_POINT('Ctrl Pts',(-38.5124571785126,34.9988611669454,5.11258330249198));
#19141=CARTESIAN_POINT('Ctrl Pts',(-38.5138066110977,35.0022702462197,5.38741669750802));
#19142=CARTESIAN_POINT('Ctrl Pts',(-38.5092949444589,34.2594597724306,5.42094378579333));
#19143=CARTESIAN_POINT('Ctrl Pts',(-38.2784657870358,33.5140853838181,5.45447087407863));
#19144=CARTESIAN_POINT('Ctrl Pts',(-37.8426352258847,32.9188002435034,5.48799796236394));
#19145=CARTESIAN_POINT('Ctrl Pts',(-37.1623350357574,31.9896029126267,5.54033133814803));
#19146=CARTESIAN_POINT('Ctrl Pts',(-35.9825496061728,31.4260975368425,5.59266471393211));
#19147=CARTESIAN_POINT('Ctrl Pts',(-34.8322413698574,31.4809342241349,5.6449980897162));
#19148=CARTESIAN_POINT('Ctrl Pts',(-33.681933133542,31.5357709114273,5.69733146550028));
#19149=CARTESIAN_POINT('Ctrl Pts',(-32.5611020904959,32.2089496617965,5.74966484128436));
#19150=CARTESIAN_POINT('Ctrl Pts',(-31.9722782631938,33.1986480172104,5.80199821706845));
#19151=CARTESIAN_POINT('Ctrl Pts',(-31.3834544358917,34.1883463726244,5.85433159285253));
#19152=CARTESIAN_POINT('Ctrl Pts',(-31.3266378243335,35.4945643330831,5.90666496863662));
#19153=CARTESIAN_POINT('Ctrl Pts',(-31.8273023322845,36.531651876217,5.95899834442071));
#19154=CARTESIAN_POINT('Ctrl Pts',(-32.3279668402356,37.5687394193509,6.01133172020479));
#19155=CARTESIAN_POINT('Ctrl Pts',(-33.3861124676959,38.3366965451598,6.06366509598887));
#19156=CARTESIAN_POINT('Ctrl Pts',(-34.5273147413959,38.4912078741205,6.11599847177296));
#19157=CARTESIAN_POINT('Ctrl Pts',(-35.668517015096,38.6457192030811,6.16833184755704));
#19158=CARTESIAN_POINT('Ctrl Pts',(-36.8927759350357,38.1867847351935,6.22066522334113));
#19159=CARTESIAN_POINT('Ctrl Pts',(-37.6511887502036,37.3201661507465,6.27299859912521));
#19160=CARTESIAN_POINT('Ctrl Pts',(-38.2039026464539,36.688594367157,6.31113796525282));
#19161=CARTESIAN_POINT('Ctrl Pts',(-38.5091981905113,35.8404949979527,6.34927733138042));
#19162=CARTESIAN_POINT('Ctrl Pts',(-38.5163029138352,34.997016742257,6.38741669750802));
#19163=CARTESIAN_POINT('Origin',(-35.,35.,4.));
#19164=CARTESIAN_POINT('',(-38.521739013009,35.0017650567249,7.38741669750802));
#19165=CARTESIAN_POINT('',(-38.5153120432796,35.002811202661,7.11258330249199));
#19166=CARTESIAN_POINT('',(-38.5175,35.,4.));
#19167=CARTESIAN_POINT('',(-32.3264680662287,37.2858331630075,8.));
#19168=CARTESIAN_POINT('Ctrl Pts',(-38.521739013009,35.0017650567249,7.38741669750802));
#19169=CARTESIAN_POINT('Ctrl Pts',(-38.515045138314,33.9623979425516,7.43461100431976));
#19170=CARTESIAN_POINT('Ctrl Pts',(-38.025374647688,32.917767542155,7.4818053111315));
#19171=CARTESIAN_POINT('Ctrl Pts',(-37.2186053621485,32.2635140899837,7.52899961794324));
#19172=CARTESIAN_POINT('Ctrl Pts',(-36.3239855860891,31.5380178578407,7.58133299372732));
#19173=CARTESIAN_POINT('Ctrl Pts',(-35.039448183402,31.2925450618756,7.63366636951141));
#19174=CARTESIAN_POINT('Ctrl Pts',(-33.9411232613757,31.6392615106971,7.68599974529549));
#19175=CARTESIAN_POINT('Ctrl Pts',(-32.8427983393495,31.9859779595187,7.73833312107958));
#19176=CARTESIAN_POINT('Ctrl Pts',(-31.9306858979841,32.9248836531268,7.79066649686366));
#19177=CARTESIAN_POINT('Ctrl Pts',(-31.6136962443577,34.0300695623378,7.84299987264775));
#19178=CARTESIAN_POINT('Ctrl Pts',(-31.2967065907312,35.1352554715487,7.89533324843183));
#19179=CARTESIAN_POINT('Ctrl Pts',(-31.5748397248436,36.4067215963625,7.94766662421592));
#19180=CARTESIAN_POINT('Ctrl Pts',(-32.3264680662287,37.2858331630075,8.));
#19181=CARTESIAN_POINT('',(-37.6785007864356,37.2890249916441,8.));
#19182=CARTESIAN_POINT('Origin',(-35.,35.,8.));
#19183=CARTESIAN_POINT('Ctrl Pts',(-37.6785239274887,37.2890398567007,8.));
#19184=CARTESIAN_POINT('Ctrl Pts',(-36.9607510630042,38.1233253004298,7.95000212253756));
#19185=CARTESIAN_POINT('Ctrl Pts',(-35.8186698457281,38.5989197552422,7.90000424507511));
#19186=CARTESIAN_POINT('Ctrl Pts',(-34.7217022012346,38.5118537728532,7.85000636761267));
#19187=CARTESIAN_POINT('Ctrl Pts',(-33.5734930596489,38.4207207687012,7.79767299182859));
#19188=CARTESIAN_POINT('Ctrl Pts',(-32.4747106147993,37.7131336670436,7.7453396160445));
#19189=CARTESIAN_POINT('Ctrl Pts',(-31.9173295125726,36.7055536114064,7.69300624026042));
#19190=CARTESIAN_POINT('Ctrl Pts',(-31.3599484103458,35.6979735557692,7.64067286447633));
#19191=CARTESIAN_POINT('Ctrl Pts',(-31.3439686507417,34.3904005461523,7.58833948869225));
#19192=CARTESIAN_POINT('Ctrl Pts',(-31.8768870047646,33.3694814192899,7.53600611290817));
#19193=CARTESIAN_POINT('Ctrl Pts',(-32.4098053587874,32.3485622924274,7.48367273712408));
#19194=CARTESIAN_POINT('Ctrl Pts',(-33.4916218264372,31.6142970483194,7.43133936134));
#19195=CARTESIAN_POINT('Ctrl Pts',(-34.6371339251584,31.4957034085517,7.37900598555591));
#19196=CARTESIAN_POINT('Ctrl Pts',(-35.7826460238797,31.3771097687841,7.32667260977183));
#19197=CARTESIAN_POINT('Ctrl Pts',(-36.9918537536724,31.8741877333568,7.27433923398774));
#19198=CARTESIAN_POINT('Ctrl Pts',(-37.7226848809369,32.7641661288242,7.22200585820366));
#19199=CARTESIAN_POINT('Ctrl Pts',(-38.232043765465,33.3844440368906,7.18553167296644));
#19200=CARTESIAN_POINT('Ctrl Pts',(-38.5090307393652,34.1955737201714,7.14905748772921));
#19201=CARTESIAN_POINT('Ctrl Pts',(-38.5153120432796,35.002811202661,7.11258330249199));
#19202=CARTESIAN_POINT('Origin',(-35.,-35.,4.));
#19203=CARTESIAN_POINT('',(-38.5120271382808,-35.0001374244476,0.387416697508025));
#19204=CARTESIAN_POINT('',(-38.5151976130935,-35.0046525930694,0.112583302491978));
#19205=CARTESIAN_POINT('',(-38.5175,-35.,4.));
#19206=CARTESIAN_POINT('',(-37.6735319337713,-32.7141668369925,0.));
#19207=CARTESIAN_POINT('Ctrl Pts',(-38.5151976130935,-35.0046525930694,
0.112583302491978));
#19208=CARTESIAN_POINT('Ctrl Pts',(-38.5080219923978,-34.1767290340604,
0.075055534994651));
#19209=CARTESIAN_POINT('Ctrl Pts',(-38.2125174896864,-33.3445694048179,
0.0375277674973242));
#19210=CARTESIAN_POINT('Ctrl Pts',(-37.6735319337713,-32.7141668369925,
-2.28983498828939E-15));
#19211=CARTESIAN_POINT('',(-32.3214990837181,-32.7109751024398,8.09549783939668E-17));
#19212=CARTESIAN_POINT('Origin',(-35.,-35.,0.));
#19213=CARTESIAN_POINT('Ctrl Pts',(-32.3214759334524,-32.7109602322923,
3.12480707463443E-17));
#19214=CARTESIAN_POINT('Ctrl Pts',(-33.0392487617403,-31.8766749582113,
0.0499978774624439));
#19215=CARTESIAN_POINT('Ctrl Pts',(-34.1813300785248,-31.4010800346315,
0.099995754924887));
#19216=CARTESIAN_POINT('Ctrl Pts',(-35.2782977997678,-31.4881459202074,
0.149993632387331));
#19217=CARTESIAN_POINT('Ctrl Pts',(-36.4265070216881,-31.5792788230239,
0.202327008171415));
#19218=CARTESIAN_POINT('Ctrl Pts',(-37.5252895219377,-32.2868662308611,
0.254660383955499));
#19219=CARTESIAN_POINT('Ctrl Pts',(-38.0826706431354,-33.2944463926721,
0.306993759739583));
#19220=CARTESIAN_POINT('Ctrl Pts',(-38.3681877823846,-33.8105769080839,
0.333801405662397));
#19221=CARTESIAN_POINT('Ctrl Pts',(-38.5116424994856,-34.4054248019609,
0.360609051585211));
#19222=CARTESIAN_POINT('Ctrl Pts',(-38.5120271382808,-35.0001374244476,
0.387416697508025));
#19223=CARTESIAN_POINT('Origin',(-35.,-35.,4.));
#19224=CARTESIAN_POINT('',(-38.5212304296149,-35.0021519659852,1.38741669750803));
#19225=CARTESIAN_POINT('',(-38.5220168341852,-34.9983176676613,1.11258330249198));
#19226=CARTESIAN_POINT('',(-38.5175,-35.,4.));
#19227=CARTESIAN_POINT('Ctrl Pts',(-38.5220168341852,-34.9983176676613,
1.11258330249198));
#19228=CARTESIAN_POINT('Ctrl Pts',(-38.52260684792,-34.8986110126186,1.10805583214991));
#19229=CARTESIAN_POINT('Ctrl Pts',(-38.5187311767415,-34.7989511930367,
1.10352836180784));
#19230=CARTESIAN_POINT('Ctrl Pts',(-38.5102392653976,-34.699686678491,1.09900089146577));
#19231=CARTESIAN_POINT('Ctrl Pts',(-38.4120806130139,-33.5522805666331,
1.04666751568169));
#19232=CARTESIAN_POINT('Ctrl Pts',(-37.6971357336766,-32.4576920494149,
0.994334139897603));
#19233=CARTESIAN_POINT('Ctrl Pts',(-36.6859405355102,-31.906559687218,0.942000764113519));
#19234=CARTESIAN_POINT('Ctrl Pts',(-35.6747453373438,-31.355427325021,0.889667388329434));
#19235=CARTESIAN_POINT('Ctrl Pts',(-34.3672998203483,-31.3477511178455,
0.83733401254535));
#19236=CARTESIAN_POINT('Ctrl Pts',(-33.3498297550083,-31.8872254772169,
0.785000636761265));
#19237=CARTESIAN_POINT('Ctrl Pts',(-32.3323596896683,-32.4266998365882,
0.732667260977181));
#19238=CARTESIAN_POINT('Ctrl Pts',(-31.6048650759839,-33.5133247625066,
0.680333885193095));
#19239=CARTESIAN_POINT('Ctrl Pts',(-31.4934686932928,-34.6593973938948,
0.628000509409011));
#19240=CARTESIAN_POINT('Ctrl Pts',(-31.3820723106017,-35.8054700252831,
0.575667133624927));
#19241=CARTESIAN_POINT('Ctrl Pts',(-31.8867741589039,-37.0109903621411,
0.523333757840844));
#19242=CARTESIAN_POINT('Ctrl Pts',(-32.7813942262272,-37.7364865047087,
0.47100038205676));
#19243=CARTESIAN_POINT('Ctrl Pts',(-33.6760142935505,-38.4619826472763,
0.418667006272675));
#19244=CARTESIAN_POINT('Ctrl Pts',(-34.9605525798949,-38.7074545955534,
0.366333630488589));
#19245=CARTESIAN_POINT('Ctrl Pts',(-36.0588770784695,-38.3607385484851,
0.314000254704505));
#19246=CARTESIAN_POINT('Ctrl Pts',(-37.157201577044,-38.0140225014167,0.26166687892042));
#19247=CARTESIAN_POINT('Ctrl Pts',(-38.0693122878488,-37.0751184590028,
0.209333503136336));
#19248=CARTESIAN_POINT('Ctrl Pts',(-38.3863019623769,-35.9699324345579,
0.157000127352251));
#19249=CARTESIAN_POINT('Ctrl Pts',(-38.4759813473142,-35.6572648277626,
0.142194519065493));
#19250=CARTESIAN_POINT('Ctrl Pts',(-38.518028568312,-35.3312883810079,0.127388910778735));
#19251=CARTESIAN_POINT('Ctrl Pts',(-38.5151976130935,-35.0046525930694,
0.112583302491978));
#19252=CARTESIAN_POINT('Ctrl Pts',(-38.5120271382808,-35.0001374244476,
0.387416697508025));
#19253=CARTESIAN_POINT('Ctrl Pts',(-38.5123933840156,-35.5664114565052,
0.412942427369296));
#19254=CARTESIAN_POINT('Ctrl Pts',(-38.3830453480461,-36.1325628449505,
0.438468157230567));
#19255=CARTESIAN_POINT('Ctrl Pts',(-38.1231131273625,-36.6305186098067,
0.463993887091838));
#19256=CARTESIAN_POINT('Ctrl Pts',(-37.5901947482463,-37.6514377493457,
0.516327262875923));
#19257=CARTESIAN_POINT('Ctrl Pts',(-36.5083782478681,-38.3857031126391,
0.568660638660007));
#19258=CARTESIAN_POINT('Ctrl Pts',(-35.362866098922,-38.5042967770896,0.620994014444091));
#19259=CARTESIAN_POINT('Ctrl Pts',(-34.2173539499758,-38.6228904415402,
0.673327390228176));
#19260=CARTESIAN_POINT('Ctrl Pts',(-33.0081461524618,-38.1258124071479,
0.72566076601226));
#19261=CARTESIAN_POINT('Ctrl Pts',(-32.2773149895643,-37.2358339601687,
0.777994141796345));
#19262=CARTESIAN_POINT('Ctrl Pts',(-31.5464838266669,-36.3458555131895,
0.83032751758043));
#19263=CARTESIAN_POINT('Ctrl Pts',(-31.294029298386,-35.0629766536234,0.882660893364515));
#19264=CARTESIAN_POINT('Ctrl Pts',(-31.6331812255463,-33.9624299433603,
0.934994269148599));
#19265=CARTESIAN_POINT('Ctrl Pts',(-31.9723331527066,-32.8618832330971,
0.987327644932684));
#19266=CARTESIAN_POINT('Ctrl Pts',(-32.9030915353081,-31.9436686721369,
1.03966102071677));
#19267=CARTESIAN_POINT('Ctrl Pts',(-34.0081262229406,-31.6194484991129,
1.09199439650085));
#19268=CARTESIAN_POINT('Ctrl Pts',(-35.1131609105731,-31.2952283260889,
1.14432777228494));
#19269=CARTESIAN_POINT('Ctrl Pts',(-36.3924719032364,-31.5650025410011,
1.19666114806902));
#19270=CARTESIAN_POINT('Ctrl Pts',(-37.2724839907223,-32.3078283275476,
1.24899452385311));
#19271=CARTESIAN_POINT('Ctrl Pts',(-38.0483635269158,-32.9627549301865,
1.29513524840475));
#19272=CARTESIAN_POINT('Ctrl Pts',(-38.5138518348506,-33.9854036989656,
1.34127597295639));
#19273=CARTESIAN_POINT('Ctrl Pts',(-38.5212304296149,-35.0021519659852,
1.38741669750803));
#19274=CARTESIAN_POINT('Origin',(-35.,-35.,4.));
#19275=CARTESIAN_POINT('',(-38.5169621951111,-34.9969726963287,2.38741669750803));
#19276=CARTESIAN_POINT('',(-38.5122617995812,-34.9992080290324,2.11258330249198));
#19277=CARTESIAN_POINT('',(-38.5175,-35.,4.));
#19278=CARTESIAN_POINT('Ctrl Pts',(-38.5122617995812,-34.9992080290324,
2.11258330249198));
#19279=CARTESIAN_POINT('Ctrl Pts',(-38.5133509957446,-34.4699799892041,
2.08872275352108));
#19280=CARTESIAN_POINT('Ctrl Pts',(-38.4009678500058,-33.9411911577145,
2.06486220455019));
#19281=CARTESIAN_POINT('Ctrl Pts',(-38.1726980103725,-33.4683479591114,
2.04100165557929));
#19282=CARTESIAN_POINT('Ctrl Pts',(-37.6720334484517,-32.4312603032644,
1.98866827979521));
#19283=CARTESIAN_POINT('Ctrl Pts',(-36.613887707127,-31.6633030916115,1.93633490401112));
#19284=CARTESIAN_POINT('Ctrl Pts',(-35.4726853098873,-31.5087917472057,
1.88400152822704));
#19285=CARTESIAN_POINT('Ctrl Pts',(-34.3314829126475,-31.3542804028,1.83166815244296));
#19286=CARTESIAN_POINT('Ctrl Pts',(-33.1072238594927,-31.8132149256414,
1.77933477665887));
#19287=CARTESIAN_POINT('Ctrl Pts',(-32.3488109629184,-32.6798336014156,
1.72700140087479));
#19288=CARTESIAN_POINT('Ctrl Pts',(-31.5903980663441,-33.5464522771898,
1.6746680250907));
#19289=CARTESIAN_POINT('Ctrl Pts',(-31.2978313263503,-34.8207551058968,
1.62233464930662));
#19290=CARTESIAN_POINT('Ctrl Pts',(-31.602283651433,-35.931394685751,1.57000127352253));
#19291=CARTESIAN_POINT('Ctrl Pts',(-31.9067359765157,-37.0420342656052,
1.51766789773845));
#19292=CARTESIAN_POINT('Ctrl Pts',(-32.808207366675,-37.9890105966065,1.46533452195436));
#19293=CARTESIAN_POINT('Ctrl Pts',(-33.9025203970559,-38.3477576413965,
1.41300114617028));
#19294=CARTESIAN_POINT('Ctrl Pts',(-34.9968334274368,-38.7065046861866,
1.36066777038619));
#19295=CARTESIAN_POINT('Ctrl Pts',(-36.2839880980393,-38.4770224447653,
1.30833439460211));
#19296=CARTESIAN_POINT('Ctrl Pts',(-37.1868792206255,-37.7621694708059,
1.25600101881803));
#19297=CARTESIAN_POINT('Ctrl Pts',(-38.0116593343501,-37.1091599302205,
1.20819511337601));
#19298=CARTESIAN_POINT('Ctrl Pts',(-38.515786834056,-36.0511278602802,1.16038920793399));
#19299=CARTESIAN_POINT('Ctrl Pts',(-38.5220168341852,-34.9983176676613,
1.11258330249198));
#19300=CARTESIAN_POINT('Ctrl Pts',(-38.5212304296149,-35.0021519659852,
1.38741669750803));
#19301=CARTESIAN_POINT('Ctrl Pts',(-38.5222207275437,-35.1386120556355,
1.39360934874047));
#19302=CARTESIAN_POINT('Ctrl Pts',(-38.5149591261082,-35.2749658599455,
1.39980199997291));
#19303=CARTESIAN_POINT('Ctrl Pts',(-38.4990885075235,-35.4103101250027,
1.40599465120536));
#19304=CARTESIAN_POINT('Ctrl Pts',(-38.3649677545306,-36.5540887777307,
1.45832802698944));
#19305=CARTESIAN_POINT('Ctrl Pts',(-37.6160130662365,-37.6257687250057,
1.51066140277353));
#19306=CARTESIAN_POINT('Ctrl Pts',(-36.5880243363171,-38.1448600164999,
1.56299477855761));
#19307=CARTESIAN_POINT('Ctrl Pts',(-35.5600356063977,-38.6639513079941,
1.6153281543417));
#19308=CARTESIAN_POINT('Ctrl Pts',(-34.2530128348529,-38.6304539437074,
1.66766153012578));
#19309=CARTESIAN_POINT('Ctrl Pts',(-33.2529647263785,-38.059385190685,1.71999490590987));
#19310=CARTESIAN_POINT('Ctrl Pts',(-32.2529166179041,-37.4883164376626,
1.77232828169395));
#19311=CARTESIAN_POINT('Ctrl Pts',(-31.5598431725,-36.3796762959045,1.82466165747803));
#19312=CARTESIAN_POINT('Ctrl Pts',(-31.4844878017471,-35.2305296041615,
1.87699503326212));
#19313=CARTESIAN_POINT('Ctrl Pts',(-31.4091324309942,-34.0813829124186,
1.9293284090462));
#19314=CARTESIAN_POINT('Ctrl Pts',(-31.9514951348924,-32.8917296706907,
1.98166178483029));
#19315=CARTESIAN_POINT('Ctrl Pts',(-32.8684046918336,-32.1949562623368,
2.03399516061437));
#19316=CARTESIAN_POINT('Ctrl Pts',(-33.7853142487749,-31.4981828539828,
2.08632853639846));
#19317=CARTESIAN_POINT('Ctrl Pts',(-35.0767706587592,-31.2942892790027,
2.13866191218254));
#19318=CARTESIAN_POINT('Ctrl Pts',(-36.1637433953085,-31.6746923755375,
2.19099528796663));
#19319=CARTESIAN_POINT('Ctrl Pts',(-37.2507161318578,-32.0550954720723,
2.24332866375071));
#19320=CARTESIAN_POINT('Ctrl Pts',(-38.1332051949721,-33.019795240122,2.29566203953479));
#19321=CARTESIAN_POINT('Ctrl Pts',(-38.4155423057474,-34.1362638239756,
2.34799541531888));
#19322=CARTESIAN_POINT('Ctrl Pts',(-38.4864345470726,-34.416598775556,2.36113584271526));
#19323=CARTESIAN_POINT('Ctrl Pts',(-38.519489264757,-34.7065022308021,2.37427627011164));
#19324=CARTESIAN_POINT('Ctrl Pts',(-38.5169621951111,-34.9969726963287,
2.38741669750803));
#19325=CARTESIAN_POINT('Origin',(-35.,-35.,4.));
#19326=CARTESIAN_POINT('',(-38.5133646692972,-35.0020090495363,3.38741669750803));
#19327=CARTESIAN_POINT('',(-38.5195236027652,-35.0027703381826,3.11258330249198));
#19328=CARTESIAN_POINT('',(-38.5175,-35.,4.));
#19329=CARTESIAN_POINT('Ctrl Pts',(-38.5195236027652,-35.0027703381826,
3.11258330249198));
#19330=CARTESIAN_POINT('Ctrl Pts',(-38.5112998170852,-34.0497594617567,
3.06938967489226));
#19331=CARTESIAN_POINT('Ctrl Pts',(-38.1096194803006,-33.0906361399806,
3.02619604729253));
#19332=CARTESIAN_POINT('Ctrl Pts',(-37.4184570108864,-32.4381577473637,
2.98300241969281));
#19333=CARTESIAN_POINT('Ctrl Pts',(-36.5810449376309,-31.6476152805848,
2.93066904390873));
#19334=CARTESIAN_POINT('Ctrl Pts',(-35.3186808383768,-31.3072193659425,
2.87833566812464));
#19335=CARTESIAN_POINT('Ctrl Pts',(-34.1973517093896,-31.5695881165025,
2.82600229234056));
#19336=CARTESIAN_POINT('Ctrl Pts',(-33.0760225804023,-31.8319568670625,
2.77366891655648));
#19337=CARTESIAN_POINT('Ctrl Pts',(-32.0957284216819,-32.6970902828246,
2.72133554077239));
#19338=CARTESIAN_POINT('Ctrl Pts',(-31.6959888274348,-33.7771017035233,
2.66900216498831));
#19339=CARTESIAN_POINT('Ctrl Pts',(-31.2962492331877,-34.8571131242219,
2.61666878920422));
#19340=CARTESIAN_POINT('Ctrl Pts',(-31.477064203414,-36.1520025498569,2.56433541342014));
#19341=CARTESIAN_POINT('Ctrl Pts',(-32.1573644670244,-37.0811999812203,
2.51200203763605));
#19342=CARTESIAN_POINT('Ctrl Pts',(-32.8376647306348,-38.0103974125836,
2.45966866185197));
#19343=CARTESIAN_POINT('Ctrl Pts',(-34.0174502876292,-38.5739028496752,
2.40733528606788));
#19344=CARTESIAN_POINT('Ctrl Pts',(-35.1677586482437,-38.5190661562666,
2.3550019102838));
#19345=CARTESIAN_POINT('Ctrl Pts',(-36.3180670088582,-38.4642294628581,
2.30266853449971));
#19346=CARTESIAN_POINT('Ctrl Pts',(-37.4388981730927,-37.7910506389493,
2.25033515871563));
#19347=CARTESIAN_POINT('Ctrl Pts',(-38.0277220639514,-36.8013521769744,
2.19800178293155));
#19348=CARTESIAN_POINT('Ctrl Pts',(-38.3480813072967,-36.2628905837198,
2.16952895611836));
#19349=CARTESIAN_POINT('Ctrl Pts',(-38.5109620602598,-35.6307365970085,
2.14105612930517));
#19350=CARTESIAN_POINT('Ctrl Pts',(-38.5122617995812,-34.9992080290324,
2.11258330249198));
#19351=CARTESIAN_POINT('Ctrl Pts',(-38.5169621951111,-34.9969726963287,
2.38741669750803));
#19352=CARTESIAN_POINT('Ctrl Pts',(-38.5094248976387,-35.8633367513267,
2.42660964589573));
#19353=CARTESIAN_POINT('Ctrl Pts',(-38.1853504786061,-36.7347449543441,
2.46580259428343));
#19354=CARTESIAN_POINT('Ctrl Pts',(-37.6045916266667,-37.3723557446642,
2.50499554267113));
#19355=CARTESIAN_POINT('Ctrl Pts',(-36.8291186783745,-38.2237416818415,
2.55732891845522));
#19356=CARTESIAN_POINT('Ctrl Pts',(-35.5959876233539,-38.6582761565386,
2.6096622942393));
#19357=CARTESIAN_POINT('Ctrl Pts',(-34.4580786668646,-38.4811335311572,
2.66199567002338));
#19358=CARTESIAN_POINT('Ctrl Pts',(-33.3201697103753,-38.3039909057758,
2.71432904580747));
#19359=CARTESIAN_POINT('Ctrl Pts',(-32.2774828524173,-37.5151711803159,
2.76666242159156));
#19360=CARTESIAN_POINT('Ctrl Pts',(-31.7975117563928,-36.4683454731577,
2.81899579737564));
#19361=CARTESIAN_POINT('Ctrl Pts',(-31.3175406603683,-35.4215197659996,
2.87132917315973));
#19362=CARTESIAN_POINT('Ctrl Pts',(-31.4002853262773,-34.1166880771431,
2.92366254894381));
#19363=CARTESIAN_POINT('Ctrl Pts',(-32.008646781737,-33.138877947982,2.97599592472789));
#19364=CARTESIAN_POINT('Ctrl Pts',(-32.6170082371967,-32.1610678188208,
3.02832930051198));
#19365=CARTESIAN_POINT('Ctrl Pts',(-33.7509864822071,-31.5102792493549,
3.08066267629606));
#19366=CARTESIAN_POINT('Ctrl Pts',(-34.9021569334111,-31.4782964190287,
3.13299605208015));
#19367=CARTESIAN_POINT('Ctrl Pts',(-36.0533273846151,-31.4463135887025,
3.18532942786423));
#19368=CARTESIAN_POINT('Ctrl Pts',(-37.2216900420126,-32.033136497516,3.23766280364832));
#19369=CARTESIAN_POINT('Ctrl Pts',(-37.883403902666,-32.9756602781289,3.2899961794324));
#19370=CARTESIAN_POINT('Ctrl Pts',(-38.2940055257973,-33.5605079247801,
3.32246968545761));
#19371=CARTESIAN_POINT('Ctrl Pts',(-38.5095293369816,-34.2823130619538,
3.35494319148282));
#19372=CARTESIAN_POINT('Ctrl Pts',(-38.5133646692972,-35.0020090495363,
3.38741669750803));
#19373=CARTESIAN_POINT('Origin',(-35.,-35.,4.));
#19374=CARTESIAN_POINT('',(-38.5230462440028,-35.0002063500719,4.38741669750802));
#19375=CARTESIAN_POINT('',(-38.5188572457002,-34.9970948475072,4.11258330249198));
#19376=CARTESIAN_POINT('',(-38.5175,-35.,4.));
#19377=CARTESIAN_POINT('Ctrl Pts',(-38.5188572457002,-34.9970948475072,
4.11258330249198));
#19378=CARTESIAN_POINT('Ctrl Pts',(-38.5208451479049,-34.772082045238,4.10238997204752));
#19379=CARTESIAN_POINT('Ctrl Pts',(-38.5010645257441,-34.5474171474031,
4.09219664160305));
#19380=CARTESIAN_POINT('Ctrl Pts',(-38.4582307571508,-34.3272370005912,
4.08200331115859));
#19381=CARTESIAN_POINT('Ctrl Pts',(-38.2383187548614,-33.1968144732253,
4.0296699353745));
#19382=CARTESIAN_POINT('Ctrl Pts',(-37.410753954154,-32.1846045081767,3.97733655959042));
#19383=CARTESIAN_POINT('Ctrl Pts',(-36.3465790030625,-31.7444362988739,
3.92500318380633));
#19384=CARTESIAN_POINT('Ctrl Pts',(-35.2824040519711,-31.3042680895711,
3.87266980802225));
#19385=CARTESIAN_POINT('Ctrl Pts',(-33.9816189504956,-31.4361416360142,
3.82033643223816));
#19386=CARTESIAN_POINT('Ctrl Pts',(-33.0274369384391,-32.0809308006472,
3.76800305645408));
#19387=CARTESIAN_POINT('Ctrl Pts',(-32.0732549263827,-32.7257199652802,
3.71566968067));
#19388=CARTESIAN_POINT('Ctrl Pts',(-31.4656760037452,-33.8834247481031,
3.66333630488591));
#19389=CARTESIAN_POINT('Ctrl Pts',(-31.4771110949952,-35.0349826573345,
3.61100292910183));
#19390=CARTESIAN_POINT('Ctrl Pts',(-31.4885461862452,-36.1865405665659,
3.55866955331774));
#19391=CARTESIAN_POINT('Ctrl Pts',(-32.1189952913826,-37.3319516022057,
3.50633617753366));
#19392=CARTESIAN_POINT('Ctrl Pts',(-33.0857935298184,-37.957665230428,3.45400280174958));
#19393=CARTESIAN_POINT('Ctrl Pts',(-34.0525917682542,-38.5833788586504,
3.40166942596549));
#19394=CARTESIAN_POINT('Ctrl Pts',(-35.3557391399884,-38.6893950794552,
3.3493360501814));
#19395=CARTESIAN_POINT('Ctrl Pts',(-36.4109632703443,-38.2281810151433,
3.29700267439732));
#19396=CARTESIAN_POINT('Ctrl Pts',(-37.4661874007003,-37.7669669508313,
3.24466929861323));
#19397=CARTESIAN_POINT('Ctrl Pts',(-38.273488289678,-36.7385226014027,3.19233592282915));
#19398=CARTESIAN_POINT('Ctrl Pts',(-38.4709087105384,-35.6039559172305,
3.14000254704507));
#19399=CARTESIAN_POINT('Ctrl Pts',(-38.5053871462609,-35.4058098271621,
3.1308627988607));
#19400=CARTESIAN_POINT('Ctrl Pts',(-38.5212637513569,-35.2044269229967,
3.12172305067634));
#19401=CARTESIAN_POINT('Ctrl Pts',(-38.5195236027652,-35.0027703381826,
3.11258330249198));
#19402=CARTESIAN_POINT('Ctrl Pts',(-38.5133646692972,-35.0020090495363,
3.38741669750803));
#19403=CARTESIAN_POINT('Ctrl Pts',(-38.5157102491126,-35.4421545813516,
3.4072765672669));
#19404=CARTESIAN_POINT('Ctrl Pts',(-38.4388801758726,-35.8815112497523,
3.42713643702578));
#19405=CARTESIAN_POINT('Ctrl Pts',(-38.2790749297269,-36.2882689858157,
3.44699630678465));
#19406=CARTESIAN_POINT('Ctrl Pts',(-37.8579670322255,-37.3601292604774,
3.49932968256874));
#19407=CARTESIAN_POINT('Ctrl Pts',(-36.8606861733137,-38.2056251573884,
3.55166305835282));
#19408=CARTESIAN_POINT('Ctrl Pts',(-35.7343680095528,-38.4456745351613,
3.60399643413691));
#19409=CARTESIAN_POINT('Ctrl Pts',(-34.6080498457918,-38.6857239129342,
3.65632980992099));
#19410=CARTESIAN_POINT('Ctrl Pts',(-33.3526943771818,-38.3203267715691,
3.70866318570508));
#19411=CARTESIAN_POINT('Ctrl Pts',(-32.5311462498722,-37.5133106723387,
3.76099656148916));
#19412=CARTESIAN_POINT('Ctrl Pts',(-31.7095981225626,-36.7062945731084,
3.81332993727325));
#19413=CARTESIAN_POINT('Ctrl Pts',(-31.3218573365535,-35.4576595160129,
3.86566331305733));
#19414=CARTESIAN_POINT('Ctrl Pts',(-31.5417693331035,-34.3272370181493,
3.91799668884141));
#19415=CARTESIAN_POINT('Ctrl Pts',(-31.7616813296536,-33.1968145202857,
3.9703300646255));
#19416=CARTESIAN_POINT('Ctrl Pts',(-32.5892461087628,-32.184604581654,4.02266344040958));
#19417=CARTESIAN_POINT('Ctrl Pts',(-33.653421032081,-31.7444363838389,4.07499681619367));
#19418=CARTESIAN_POINT('Ctrl Pts',(-34.7175959553992,-31.3042681860239,
4.12733019197775));
#19419=CARTESIAN_POINT('Ctrl Pts',(-36.0183810229263,-31.4361417290255,
4.17966356776184));
#19420=CARTESIAN_POINT('Ctrl Pts',(-36.9725630100801,-32.0809308768304,
4.23199694354592));
#19421=CARTESIAN_POINT('Ctrl Pts',(-37.9171401399176,-32.7192295355597,
4.28380352819995));
#19422=CARTESIAN_POINT('Ctrl Pts',(-38.5220569274439,-33.8601696875978,
4.33561011285399));
#19423=CARTESIAN_POINT('Ctrl Pts',(-38.5230462440028,-35.0002063500719,
4.38741669750802));
#19424=CARTESIAN_POINT('Origin',(-35.,-35.,4.));
#19425=CARTESIAN_POINT('',(-38.5138068989996,-34.9977297535637,5.38741669750802));
#19426=CARTESIAN_POINT('',(-38.5124574312326,-35.001138833141,5.11258330249198));
#19427=CARTESIAN_POINT('',(-38.5175,-35.,4.));
#19428=CARTESIAN_POINT('Ctrl Pts',(-38.5124574312326,-35.001138833141,5.11258330249198));
#19429=CARTESIAN_POINT('Ctrl Pts',(-38.5105122060607,-34.3463332977053,
5.08305689341869));
#19430=CARTESIAN_POINT('Ctrl Pts',(-38.3345898905329,-33.6905568650893,
5.0535304843454));
#19431=CARTESIAN_POINT('Ctrl Pts',(-37.9913532963331,-33.1388778994087,
5.02400407527211));
#19432=CARTESIAN_POINT('Ctrl Pts',(-37.3829918249966,-32.1610677447274,
4.97167069948802));
#19433=CARTESIAN_POINT('Ctrl Pts',(-36.2490135503901,-31.5102791582787,
4.91933732370394));
#19434=CARTESIAN_POINT('Ctrl Pts',(-35.0978430691422,-31.4782963271182,
4.86700394791986));
#19435=CARTESIAN_POINT('Ctrl Pts',(-33.9466725878942,-31.4463134959578,
4.81467057213577));
#19436=CARTESIAN_POINT('Ctrl Pts',(-32.7783099000047,-32.0331364200855,
4.76233719635169));
#19437=CARTESIAN_POINT('Ctrl Pts',(-32.1165960220819,-32.9756602252966,
4.7100038205676));
#19438=CARTESIAN_POINT('Ctrl Pts',(-31.454882144159,-33.9181840305077,4.65767044478352));
#19439=CARTESIAN_POINT('Ctrl Pts',(-31.2998170762027,-35.216408716802,4.60533706899943));
#19440=CARTESIAN_POINT('Ctrl Pts',(-31.7209249846943,-36.2882690194377,
4.55300369321535));
#19441=CARTESIAN_POINT('Ctrl Pts',(-32.1420328931859,-37.3601293220733,
4.50067031743126));
#19442=CARTESIAN_POINT('Ctrl Pts',(-33.1393137781253,-38.2056252410501,
4.44833694164718));
#19443=CARTESIAN_POINT('Ctrl Pts',(-34.2656319712814,-38.4456746250879,
4.39600356586309));
#19444=CARTESIAN_POINT('Ctrl Pts',(-35.3919501644375,-38.6857240091257,
4.34367019007901));
#19445=CARTESIAN_POINT('Ctrl Pts',(-36.6473056658103,-38.3203268582244,
4.29133681429492));
#19446=CARTESIAN_POINT('Ctrl Pts',(-37.468853814561,-37.5133107379322,4.23900343851084));
#19447=CARTESIAN_POINT('Ctrl Pts',(-38.1303833971331,-36.8634826809916,
4.19686339317122));
#19448=CARTESIAN_POINT('Ctrl Pts',(-38.5106390985996,-35.9273158131948,
4.1547233478316));
#19449=CARTESIAN_POINT('Ctrl Pts',(-38.5188572457002,-34.9970948475072,
4.11258330249198));
#19450=CARTESIAN_POINT('Ctrl Pts',(-38.5230462440028,-35.0002063500719,
4.38741669750802));
#19451=CARTESIAN_POINT('Ctrl Pts',(-38.5230563037894,-35.0117987220789,
4.38794348863807));
#19452=CARTESIAN_POINT('Ctrl Pts',(-38.5230039194247,-35.023391000668,4.38847027976812));
#19453=CARTESIAN_POINT('Ctrl Pts',(-38.5228888130629,-35.0349826564212,
4.38899707089817));
#19454=CARTESIAN_POINT('Ctrl Pts',(-38.5114537221114,-36.186540535599,4.44133044668226));
#19455=CARTESIAN_POINT('Ctrl Pts',(-37.8810046334278,-37.3319515413465,
4.49366382246634));
#19456=CARTESIAN_POINT('Ctrl Pts',(-36.9142064202239,-37.9576651532382,
4.54599719825043));
#19457=CARTESIAN_POINT('Ctrl Pts',(-35.94740820702,-38.5833787651299,4.59833057403451));
#19458=CARTESIAN_POINT('Ctrl Pts',(-34.6442608692957,-38.6893949831658,
4.6506639498186));
#19459=CARTESIAN_POINT('Ctrl Pts',(-33.5890367664795,-38.2281809308918,
4.70299732560268));
#19460=CARTESIAN_POINT('Ctrl Pts',(-32.5338126636633,-37.7669668786178,
4.75533070138677));
#19461=CARTESIAN_POINT('Ctrl Pts',(-31.7265117957552,-36.7385225560339,
4.80766407717085));
#19462=CARTESIAN_POINT('Ctrl Pts',(-31.529091380047,-35.6039559014703,4.85999745295494));
#19463=CARTESIAN_POINT('Ctrl Pts',(-31.3316709643388,-34.4693892469067,
4.91233082873902));
#19464=CARTESIAN_POINT('Ctrl Pts',(-31.7441310008306,-33.2287002603633,
4.9646642045231));
#19465=CARTESIAN_POINT('Ctrl Pts',(-32.5815430522312,-32.4381578142198,
5.01699758030719));
#19466=CARTESIAN_POINT('Ctrl Pts',(-33.4189551036319,-31.6476153680763,
5.06933095609127));
#19467=CARTESIAN_POINT('Ctrl Pts',(-34.6813191699414,-31.3072194623328,
5.12166433187536));
#19468=CARTESIAN_POINT('Ctrl Pts',(-35.8026482696631,-31.5695882060385,
5.17399770765944));
#19469=CARTESIAN_POINT('Ctrl Pts',(-36.9239773693848,-31.8319569497442,
5.22633108344353));
#19470=CARTESIAN_POINT('Ctrl Pts',(-37.9042715025186,-32.6970903428993,
5.27866445922761));
#19471=CARTESIAN_POINT('Ctrl Pts',(-38.3040110863345,-33.7771017354242,
5.33099783501169));
#19472=CARTESIAN_POINT('Ctrl Pts',(-38.4476597125745,-34.1652097916211,
5.34980412251047));
#19473=CARTESIAN_POINT('Ctrl Pts',(-38.5163376200166,-34.5810664169843,
5.36861041000925));
#19474=CARTESIAN_POINT('Ctrl Pts',(-38.5138068989996,-34.9977297535637,
5.38741669750802));
#19475=CARTESIAN_POINT('Origin',(-35.,-35.,4.));
#19476=CARTESIAN_POINT('',(-38.5163032009778,-35.0029832534533,6.38741669750803));
#19477=CARTESIAN_POINT('',(-38.522424122767,-35.0013091826171,6.11258330249198));
#19478=CARTESIAN_POINT('',(-38.5175,-35.,4.));
#19479=CARTESIAN_POINT('Ctrl Pts',(-38.522424122767,-35.0013091826171,6.11258330249198));
#19480=CARTESIAN_POINT('Ctrl Pts',(-38.5172132511134,-33.9256163607463,
6.06372381478986));
#19481=CARTESIAN_POINT('Ctrl Pts',(-37.9876405112709,-32.8454778142804,
6.01486432708775));
#19482=CARTESIAN_POINT('Ctrl Pts',(-37.1315953638235,-32.1949561890823,
5.96600483938563));
#19483=CARTESIAN_POINT('Ctrl Pts',(-36.2146857829733,-31.4981827625019,
5.91367146360154));
#19484=CARTESIAN_POINT('Ctrl Pts',(-34.9232293392347,-31.2942891822923,
5.86133808781746));
#19485=CARTESIAN_POINT('Ctrl Pts',(-33.8362565743057,-31.6746922887769,
5.80900471203338));
#19486=CARTESIAN_POINT('Ctrl Pts',(-32.7492838093767,-32.0550953952615,
5.75667133624929));
#19487=CARTESIAN_POINT('Ctrl Pts',(-31.8667947232573,-33.0197951884404,
5.7043379604652));
#19488=CARTESIAN_POINT('Ctrl Pts',(-31.5844576051196,-34.1362638014206,
5.65200458468112));
#19489=CARTESIAN_POINT('Ctrl Pts',(-31.302120486982,-35.2527324144008,5.59967120889704));
#19490=CARTESIAN_POINT('Ctrl Pts',(-31.6199353368261,-36.5209698471824,
5.54733783311296));
#19491=CARTESIAN_POINT('Ctrl Pts',(-32.3954083053537,-37.3723558065856,
5.49500445732887));
#19492=CARTESIAN_POINT('Ctrl Pts',(-33.1708812738812,-38.2237417659887,
5.44267108154479));
#19493=CARTESIAN_POINT('Ctrl Pts',(-34.4040123610921,-38.6582762520135,
5.3903377057607));
#19494=CARTESIAN_POINT('Ctrl Pts',(-35.5419213472807,-38.4811336220058,
5.33800432997661));
#19495=CARTESIAN_POINT('Ctrl Pts',(-36.6798303334694,-38.3039909919981,
5.28567095419253));
#19496=CARTESIAN_POINT('Ctrl Pts',(-37.722517218636,-37.515171245958,5.23333757840845));
#19497=CARTESIAN_POINT('Ctrl Pts',(-38.202488327186,-36.468345511481,5.18100420262436));
#19498=CARTESIAN_POINT('Ctrl Pts',(-38.4116604841668,-36.0121372252676,
5.15819723591357));
#19499=CARTESIAN_POINT('Ctrl Pts',(-38.5139599737744,-35.5069276682025,
5.13539026920277));
#19500=CARTESIAN_POINT('Ctrl Pts',(-38.5124574312326,-35.001138833141,5.11258330249198));
#19501=CARTESIAN_POINT('Ctrl Pts',(-38.5138068989996,-34.9977297535637,
5.38741669750802));
#19502=CARTESIAN_POINT('Ctrl Pts',(-38.5092952319858,-35.7405402881605,
5.42094378579333));
#19503=CARTESIAN_POINT('Ctrl Pts',(-38.2784660556449,-36.4859147377931,
5.45447087407864));
#19504=CARTESIAN_POINT('Ctrl Pts',(-37.8426354587898,-37.0811999269324,
5.48799796236395));
#19505=CARTESIAN_POINT('Ctrl Pts',(-37.1623352129312,-38.0103973340206,
5.54033133814803));
#19506=CARTESIAN_POINT('Ctrl Pts',(-35.982549686716,-38.5739027563021,5.59266471393212));
#19507=CARTESIAN_POINT('Ctrl Pts',(-34.8322413561292,-38.5190660643709,
5.6449980897162));
#19508=CARTESIAN_POINT('Ctrl Pts',(-33.6819330255423,-38.4642293724398,
5.69733146550029));
#19509=CARTESIAN_POINT('Ctrl Pts',(-32.5611018905839,-37.791050566296,5.74966484128437));
#19510=CARTESIAN_POINT('Ctrl Pts',(-31.9722780150789,-36.8013521300638,
5.80199821706845));
#19511=CARTESIAN_POINT('Ctrl Pts',(-31.3834541395739,-35.8116536938316,
5.85433159285254));
#19512=CARTESIAN_POINT('Ctrl Pts',(-31.3266375235224,-34.5054356275111,
5.90666496863662));
#19513=CARTESIAN_POINT('Ctrl Pts',(-31.8273020724053,-33.4683479988925,
5.95899834442071));
#19514=CARTESIAN_POINT('Ctrl Pts',(-32.3279666212882,-32.431260370274,6.01133172020479));
#19515=CARTESIAN_POINT('Ctrl Pts',(-33.3861123351056,-31.6633031793574,
6.06366509598888));
#19516=CARTESIAN_POINT('Ctrl Pts',(-34.5273147025013,-31.5087918386834,
6.11599847177296));
#19517=CARTESIAN_POINT('Ctrl Pts',(-35.668517069897,-31.3542804980094,6.16833184755705));
#19518=CARTESIAN_POINT('Ctrl Pts',(-36.892776090871,-31.8132150075779,6.22066522334113));
#19519=CARTESIAN_POINT('Ctrl Pts',(-37.6511889677791,-32.6798336612887,
6.27299859912521));
#19520=CARTESIAN_POINT('Ctrl Pts',(-38.2039029090244,-33.3114054953559,
6.31113796525282));
#19521=CARTESIAN_POINT('Ctrl Pts',(-38.509198477207,-34.1595049296877,6.34927733138042));
#19522=CARTESIAN_POINT('Ctrl Pts',(-38.5163032009778,-35.0029832534533,
6.38741669750803));
#19523=CARTESIAN_POINT('Origin',(-35.,-35.,4.));
#19524=CARTESIAN_POINT('',(-38.5217392653161,-34.9982348400382,7.38741669750802));
#19525=CARTESIAN_POINT('',(-38.5153122961063,-34.9971887940747,7.11258330249198));
#19526=CARTESIAN_POINT('',(-38.5175,-35.,4.));
#19527=CARTESIAN_POINT('',(-32.3264680662287,-32.7141668369925,8.));
#19528=CARTESIAN_POINT('Ctrl Pts',(-38.5217392653161,-34.9982348400382,
7.38741669750802));
#19529=CARTESIAN_POINT('Ctrl Pts',(-38.5150454835571,-36.0376021634142,
7.43461100431976));
#19530=CARTESIAN_POINT('Ctrl Pts',(-38.0253751592018,-37.0822329702746,
7.48180531113151));
#19531=CARTESIAN_POINT('Ctrl Pts',(-37.2186056743939,-37.7364863611315,
7.52899961794325));
#19532=CARTESIAN_POINT('Ctrl Pts',(-36.3239856773675,-38.4619825252834,
7.58133299372733));
#19533=CARTESIAN_POINT('Ctrl Pts',(-35.0394476042314,-38.7074546780583,
7.63366636951141));
#19534=CARTESIAN_POINT('Ctrl Pts',(-33.9411230034093,-38.3607385339716,
7.68599974529549));
#19535=CARTESIAN_POINT('Ctrl Pts',(-32.8427984025871,-38.0140223898848,
7.73833312107958));
#19536=CARTESIAN_POINT('Ctrl Pts',(-31.9306872740789,-37.0751179489365,
7.79066649686366));
#19537=CARTESIAN_POINT('Ctrl Pts',(-31.613697604643,-35.9699319523746,7.84299987264775));
#19538=CARTESIAN_POINT('Ctrl Pts',(-31.2967079352071,-34.8647459558128,
7.89533324843184));
#19539=CARTESIAN_POINT('Ctrl Pts',(-31.5748397248436,-33.5932784036375,
7.94766662421592));
#19540=CARTESIAN_POINT('Ctrl Pts',(-32.3264680662287,-32.7141668369925,
8.));
#19541=CARTESIAN_POINT('',(-37.6785009901498,-32.7109751557132,8.));
#19542=CARTESIAN_POINT('Origin',(-35.,-35.,8.));
#19543=CARTESIAN_POINT('Ctrl Pts',(-37.6785241456451,-32.7109602826759,
8.));
#19544=CARTESIAN_POINT('Ctrl Pts',(-36.9607513379489,-31.8766751051408,
7.95000212253756));
#19545=CARTESIAN_POINT('Ctrl Pts',(-35.8186699645707,-31.4010799150529,
7.90000424507511));
#19546=CARTESIAN_POINT('Ctrl Pts',(-34.7217021996619,-31.4881457455928,
7.85000636761267));
#19547=CARTESIAN_POINT('Ctrl Pts',(-33.573492932036,-31.5792785908026,7.79767299182859));
#19548=CARTESIAN_POINT('Ctrl Pts',(-32.4747104002448,-32.2868661727234,
7.7453396160445));
#19549=CARTESIAN_POINT('Ctrl Pts',(-31.9173292682424,-33.2944463949298,
7.69300624026042));
#19550=CARTESIAN_POINT('Ctrl Pts',(-31.3599481362399,-34.3020266171361,
7.64067286447633));
#19551=CARTESIAN_POINT('Ctrl Pts',(-31.3439684040262,-35.609599479628,7.58833948869224));
#19552=CARTESIAN_POINT('Ctrl Pts',(-31.8768867974267,-36.6305186264058,
7.53600611290816));
#19553=CARTESIAN_POINT('Ctrl Pts',(-32.4098051908272,-37.6514377731836,
7.48367273712407));
#19554=CARTESIAN_POINT('Ctrl Pts',(-33.491621709842,-38.3857032042473,7.43133936134));
#19555=CARTESIAN_POINT('Ctrl Pts',(-34.6371338873761,-38.5042968827328,
7.37900598555591));
#19556=CARTESIAN_POINT('Ctrl Pts',(-35.7826460649101,-38.6228905612183,
7.32667260977183));
#19557=CARTESIAN_POINT('Ctrl Pts',(-36.9918539009634,-38.1258124871256,
7.27433923398775));
#19558=CARTESIAN_POINT('Ctrl Pts',(-37.7226850841419,-37.2358340108349,
7.22200585820366));
#19559=CARTESIAN_POINT('Ctrl Pts',(-38.2320440076398,-36.615556046438,7.18553167296643));
#19560=CARTESIAN_POINT('Ctrl Pts',(-38.5090309960538,-35.8044263207662,
7.14905748772921));
#19561=CARTESIAN_POINT('Ctrl Pts',(-38.5153122961063,-34.9971887940747,
7.11258330249198));
#19562=CARTESIAN_POINT('Origin',(35.,-35.,4.));
#19563=CARTESIAN_POINT('',(31.4879726191333,-35.0001375015905,0.387416697508024));
#19564=CARTESIAN_POINT('',(31.4847993146864,-35.0046492582639,0.112583302491975));
#19565=CARTESIAN_POINT('',(31.4825,-35.,4.));
#19566=CARTESIAN_POINT('',(32.3264680662287,-32.7141668369925,0.));
#19567=CARTESIAN_POINT('Ctrl Pts',(31.4847993146864,-35.0046492582639,0.112583302491975));
#19568=CARTESIAN_POINT('Ctrl Pts',(31.4919760559448,-34.1767269622227,0.0750555349946493));
#19569=CARTESIAN_POINT('Ctrl Pts',(31.7874825103136,-33.3445694048179,0.037527767497323));
#19570=CARTESIAN_POINT('Ctrl Pts',(32.3264680662287,-32.7141668369925,-2.98372437868011E-15));
#19571=CARTESIAN_POINT('',(37.6785011129036,-32.7109752438421,-5.55678203018928E-16));
#19572=CARTESIAN_POINT('Origin',(35.,-35.,0.));
#19573=CARTESIAN_POINT('Ctrl Pts',(37.6785242770714,-32.7109603660127,-2.86292032689789E-16));
#19574=CARTESIAN_POINT('Ctrl Pts',(36.9607515035944,-31.8766753489742,0.0499978774624439));
#19575=CARTESIAN_POINT('Ctrl Pts',(35.8186700361932,-31.4010797162719,0.099995754924888));
#19576=CARTESIAN_POINT('Ctrl Pts',(34.7217021987141,-31.4881454554173,0.149993632387332));
#19577=CARTESIAN_POINT('Ctrl Pts',(33.5734928551282,-31.5792782049632,0.202327008171416));
#19578=CARTESIAN_POINT('Ctrl Pts',(32.4747102708807,-32.2868660760186,0.2546603839555));
#19579=CARTESIAN_POINT('Ctrl Pts',(31.9173291209027,-33.2944463985812,0.306993759739584));
#19580=CARTESIAN_POINT('Ctrl Pts',(31.6318119669108,-33.8105769963377,0.333801405662397));
#19581=CARTESIAN_POINT('Ctrl Pts',(31.488357249556,-34.4054248931928,0.360609051585211));
#19582=CARTESIAN_POINT('Ctrl Pts',(31.4879726191333,-35.0001375015905,0.387416697508024));
#19583=CARTESIAN_POINT('Origin',(35.,-35.,4.));
#19584=CARTESIAN_POINT('',(31.4787693262007,-35.0021519651487,1.38741669750802));
#19585=CARTESIAN_POINT('',(31.4779839561681,-34.998317589092,1.11258330249197));
#19586=CARTESIAN_POINT('',(31.4825,-35.,4.));
#19587=CARTESIAN_POINT('Ctrl Pts',(31.4779839561681,-34.998317589092,1.11258330249197));
#19588=CARTESIAN_POINT('Ctrl Pts',(31.4773939435915,-34.8986109589584,1.10805583214991));
#19589=CARTESIAN_POINT('Ctrl Pts',(31.4812696152992,-34.7989511654426,1.10352836180784));
#19590=CARTESIAN_POINT('Ctrl Pts',(31.4897615265674,-34.6996866782215,1.09900089146577));
#19591=CARTESIAN_POINT('Ctrl Pts',(31.5879201780762,-33.5522808822113,1.04666751568169));
#19592=CARTESIAN_POINT('Ctrl Pts',(32.3028649757287,-32.457692848996,0.994334139897601));
#19593=CARTESIAN_POINT('Ctrl Pts',(33.314059894657,-31.906560527472,0.942000764113516));
#19594=CARTESIAN_POINT('Ctrl Pts',(34.3252548135852,-31.3554282059481,0.889667388329432));
#19595=CARTESIAN_POINT('Ctrl Pts',(35.6326998537893,-31.3477515961155,0.837334012545348));
#19596=CARTESIAN_POINT('Ctrl Pts',(36.650169778933,-31.8872259747803,0.785000636761264));
#19597=CARTESIAN_POINT('Ctrl Pts',(37.6676397040767,-32.4267003534451,0.732667260977179));
#19598=CARTESIAN_POINT('Ctrl Pts',(38.39513451416,-33.5133257206073,0.680333885193094));
#19599=CARTESIAN_POINT('Ctrl Pts',(38.5065306720619,-34.6593978563341,0.628000509409009));
#19600=CARTESIAN_POINT('Ctrl Pts',(38.6179268299637,-35.8054699920609,0.575667133624925));
#19601=CARTESIAN_POINT('Ctrl Pts',(38.1132243356843,-37.0109888963523,0.523333757840841));
#19602=CARTESIAN_POINT('Ctrl Pts',(37.2186048923566,-37.7364852312874,0.471000382056757));
#19603=CARTESIAN_POINT('Ctrl Pts',(36.3239854490289,-38.4619815662224,0.418667006272672));
#19604=CARTESIAN_POINT('Ctrl Pts',(35.0394490566529,-38.7074553318012,0.366333630488587));
#19605=CARTESIAN_POINT('Ctrl Pts',(33.9411236515154,-38.3607384247595,0.314000254704503));
#19606=CARTESIAN_POINT('Ctrl Pts',(32.842798246378,-38.0140215177178,0.261666878920419));
#19607=CARTESIAN_POINT('Ctrl Pts',(31.930683828479,-37.0751139380558,0.209333503136335));
#19608=CARTESIAN_POINT('Ctrl Pts',(31.6136941980954,-35.9699281595357,0.157000127352251));
#19609=CARTESIAN_POINT('Ctrl Pts',(31.524014825647,-35.6572606223148,0.142194519065492));
#19610=CARTESIAN_POINT('Ctrl Pts',(31.4819679173789,-35.3312845479312,0.127388910778734));
#19611=CARTESIAN_POINT('Ctrl Pts',(31.4847993146864,-35.0046492582639,0.112583302491975));
#19612=CARTESIAN_POINT('Ctrl Pts',(31.4879726191333,-35.0001375015905,0.387416697508024));
#19613=CARTESIAN_POINT('Ctrl Pts',(31.4876063813705,-35.5664115202329,0.412942427369295));
#19614=CARTESIAN_POINT('Ctrl Pts',(31.6169544331328,-36.1325628797889,0.438468157230566));
#19615=CARTESIAN_POINT('Ctrl Pts',(31.8768866723687,-36.6305186540646,0.463993887091838));
#19616=CARTESIAN_POINT('Ctrl Pts',(32.4098050895213,-37.6514378129155,0.516327262875923));
#19617=CARTESIAN_POINT('Ctrl Pts',(33.491621639535,-38.3857033565476,0.568660638660007));
#19618=CARTESIAN_POINT('Ctrl Pts',(34.6371338646016,-38.5042970583454,0.620994014444092));
#19619=CARTESIAN_POINT('Ctrl Pts',(35.7826460896681,-38.6228907601432,0.673327390228177));
#19620=CARTESIAN_POINT('Ctrl Pts',(36.9918539897876,-38.1258126201067,0.725660766012261));
#19621=CARTESIAN_POINT('Ctrl Pts',(37.7226852066847,-37.235834095095,0.777994141796346));
#19622=CARTESIAN_POINT('Ctrl Pts',(38.4535164235819,-36.3458555700833,0.83032751758043));
#19623=CARTESIAN_POINT('Ctrl Pts',(38.7059709572567,-35.0629766600964,0.882660893364514));
#19624=CARTESIAN_POINT('Ctrl Pts',(38.3668190041959,-33.9624298822548,0.934994269148598));
#19625=CARTESIAN_POINT('Ctrl Pts',(38.027667051135,-32.8618831044132,0.987327644932683));
#19626=CARTESIAN_POINT('Ctrl Pts',(37.0969086113384,-31.9436684587171,1.03966102071677));
#19627=CARTESIAN_POINT('Ctrl Pts',(35.9918738484399,-31.6194482583158,1.09199439650085));
#19628=CARTESIAN_POINT('Ctrl Pts',(34.8868390855414,-31.2952280579146,1.14432777228494));
#19629=CARTESIAN_POINT('Ctrl Pts',(33.607527999541,-31.5650023028083,1.19666114806902));
#19630=CARTESIAN_POINT('Ctrl Pts',(32.7275158499642,-32.3078281435934,1.24899452385311));
#19631=CARTESIAN_POINT('Ctrl Pts',(31.9516362590269,-32.9627547940529,1.29513524840474));
#19632=CARTESIAN_POINT('Ctrl Pts',(31.4861479206373,-33.9854036295086,1.34127597295638));
#19633=CARTESIAN_POINT('Ctrl Pts',(31.4787693262007,-35.0021519651487,1.38741669750802));
#19634=CARTESIAN_POINT('Origin',(35.,-35.,4.));
#19635=CARTESIAN_POINT('',(31.4830375605149,-34.9969726960772,2.38741669750802));
#19636=CARTESIAN_POINT('',(31.4877390119671,-34.9992080277921,2.11258330249198));
#19637=CARTESIAN_POINT('',(31.4825,-35.,4.));
#19638=CARTESIAN_POINT('Ctrl Pts',(31.4877390119671,-34.9992080277921,2.11258330249198));
#19639=CARTESIAN_POINT('Ctrl Pts',(31.4866498159747,-34.4699801096587,2.08872275352108));
#19640=CARTESIAN_POINT('Ctrl Pts',(31.5990329357071,-33.9411914000592,2.06486220455019));
#19641=CARTESIAN_POINT('Ctrl Pts',(31.8273027226982,-33.4683483113999,2.04100165557929));
#19642=CARTESIAN_POINT('Ctrl Pts',(32.3279671691587,-32.431260896693,1.98866827979521));
#19643=CARTESIAN_POINT('Ctrl Pts',(33.3861126668897,-31.6633038687123,1.93633490401112));
#19644=CARTESIAN_POINT('Ctrl Pts',(34.5273147998293,-31.5087925573416,1.88400152822704));
#19645=CARTESIAN_POINT('Ctrl Pts',(35.6685169327689,-31.3542812459709,1.83166815244295));
#19646=CARTESIAN_POINT('Ctrl Pts',(36.892775700917,-31.8132156512101,1.77933477665887));
#19647=CARTESIAN_POINT('Ctrl Pts',(37.651188423337,-32.679834131615,1.72700140087478));
#19648=CARTESIAN_POINT('Ctrl Pts',(38.409601145757,-33.5464526120198,1.6746680250907));
#19649=CARTESIAN_POINT('Ctrl Pts',(38.7021678224488,-34.8207551675903,1.62233464930661));
#19650=CARTESIAN_POINT('Ctrl Pts',(38.3977155653522,-35.9313944817532,1.57000127352253));
#19651=CARTESIAN_POINT('Ctrl Pts',(38.0932633082556,-37.0420337959161,1.51766789773845));
#19652=CARTESIAN_POINT('Ctrl Pts',(37.1917921173706,-37.9890098686715,1.46533452195436));
#19653=CARTESIAN_POINT('Ctrl Pts',(36.0974793449018,-38.347756846785,1.41300114617028));
#19654=CARTESIAN_POINT('Ctrl Pts',(35.0031665724331,-38.7065038248986,1.36066777038619));
#19655=CARTESIAN_POINT('Ctrl Pts',(33.7160122183805,-38.4770217083703,1.30833439460211));
#19656=CARTESIAN_POINT('Ctrl Pts',(32.8131212940369,-37.7621688707036,1.25600101881802));
#19657=CARTESIAN_POINT('Ctrl Pts',(31.9883413614044,-37.10915945462,1.20819511337601));
#19658=CARTESIAN_POINT('Ctrl Pts',(31.4842139440677,-36.051127518694,1.16038920793399));
#19659=CARTESIAN_POINT('Ctrl Pts',(31.4779839561681,-34.998317589092,1.11258330249197));
#19660=CARTESIAN_POINT('Ctrl Pts',(31.4787693262007,-35.0021519651487,1.38741669750802));
#19661=CARTESIAN_POINT('Ctrl Pts',(31.4777790283158,-35.1386120640087,1.39360934874047));
#19662=CARTESIAN_POINT('Ctrl Pts',(31.4850406303498,-35.2749658775635,1.39980199997291));
#19663=CARTESIAN_POINT('Ctrl Pts',(31.5009112501032,-35.4103101518596,1.40599465120536));
#19664=CARTESIAN_POINT('Ctrl Pts',(31.6350320129721,-36.554088882664,1.45832802698944));
#19665=CARTESIAN_POINT('Ctrl Pts',(32.3839867518631,-37.6257689075961,1.51066140277353));
#19666=CARTESIAN_POINT('Ctrl Pts',(33.4119755528977,-38.1448602359127,1.56299477855761));
#19667=CARTESIAN_POINT('Ctrl Pts',(34.4399643539324,-38.6639515642293,1.6153281543417));
#19668=CARTESIAN_POINT('Ctrl Pts',(35.7469872171107,-38.6304541959304,1.66766153012578));
#19669=CARTESIAN_POINT('Ctrl Pts',(36.7470353952608,-38.0593854028254,1.71999490590987));
#19670=CARTESIAN_POINT('Ctrl Pts',(37.7470835734109,-37.4883166097203,1.77232828169395));
#19671=CARTESIAN_POINT('Ctrl Pts',(38.4401570665328,-36.3796763918093,1.82466165747804));
#19672=CARTESIAN_POINT('Ctrl Pts',(38.5155124424211,-35.2305296204218,1.87699503326212));
#19673=CARTESIAN_POINT('Ctrl Pts',(38.5908678183095,-34.0813828490343,1.9293284090462));
#19674=CARTESIAN_POINT('Ctrl Pts',(38.0485050769643,-32.8917295241703,1.98166178483029));
#19675=CARTESIAN_POINT('Ctrl Pts',(37.1315954563618,-32.1949560672859,2.03399516061437));
#19676=CARTESIAN_POINT('Ctrl Pts',(36.2146858357593,-31.4981826104015,2.08632853639846));
#19677=CARTESIAN_POINT('Ctrl Pts',(34.9232293358993,-31.2942890214966,2.13866191218254));
#19678=CARTESIAN_POINT('Ctrl Pts',(33.8362565237849,-31.6746921445243,2.19099528796663));
#19679=CARTESIAN_POINT('Ctrl Pts',(32.7492837116705,-32.055095267552,2.24332866375071));
#19680=CARTESIAN_POINT('Ctrl Pts',(31.8667945873017,-33.0197951025121,2.2956620395348));
#19681=CARTESIAN_POINT('Ctrl Pts',(31.5844574569229,-34.1362637639197,2.34799541531888));
#19682=CARTESIAN_POINT('Ctrl Pts',(31.5135652106755,-34.4165987349732,2.36113584271526));
#19683=CARTESIAN_POINT('Ctrl Pts',(31.4805104906949,-34.7065022103634,2.37427627011164));
#19684=CARTESIAN_POINT('Ctrl Pts',(31.4830375605149,-34.9969726960772,2.38741669750802));
#19685=CARTESIAN_POINT('Origin',(35.,-35.,4.));
#19686=CARTESIAN_POINT('',(31.486635086556,-35.0020090496756,3.38741669750802));
#19687=CARTESIAN_POINT('',(31.4804772106861,-35.0027703375482,3.11258330249198));
#19688=CARTESIAN_POINT('',(31.4825,-35.,4.));
#19689=CARTESIAN_POINT('Ctrl Pts',(31.4804772106861,-35.0027703375482,3.11258330249198));
#19690=CARTESIAN_POINT('Ctrl Pts',(31.4887009944635,-34.0497596813621,3.06938967489225));
#19691=CARTESIAN_POINT('Ctrl Pts',(31.8903812384068,-33.090636581221,3.02619604729253));
#19692=CARTESIAN_POINT('Ctrl Pts',(32.5815435480781,-32.4381583394347,2.98300241969281));
#19693=CARTESIAN_POINT('Ctrl Pts',(33.4189554277892,-31.647616055402,2.93066904390873));
#19694=CARTESIAN_POINT('Ctrl Pts',(34.6813192352892,-31.3072202195671,2.87833566812464));
#19695=CARTESIAN_POINT('Ctrl Pts',(35.8026481051029,-31.5695889094262,2.82600229234056));
#19696=CARTESIAN_POINT('Ctrl Pts',(36.9239769749167,-31.8319575992854,2.77366891655647));
#19697=CARTESIAN_POINT('Ctrl Pts',(37.904270907044,-32.6970908148387,2.72133554077239));
#19698=CARTESIAN_POINT('Ctrl Pts',(38.3040104089138,-33.7771019860347,2.66900216498831));
#19699=CARTESIAN_POINT('Ctrl Pts',(38.7037499107836,-34.8571131572306,2.61666878920422));
#19700=CARTESIAN_POINT('Ctrl Pts',(38.5229349823959,-36.1520022840693,2.56433541342014));
#19701=CARTESIAN_POINT('Ctrl Pts',(37.8426348759932,-37.0811995004531,2.51200203763605));
#19702=CARTESIAN_POINT('Ctrl Pts',(37.1623347695905,-38.0103967168369,2.45966866185197));
#19703=CARTESIAN_POINT('Ctrl Pts',(35.9825494851727,-38.5739020227658,2.40733528606788));
#19704=CARTESIAN_POINT('Ctrl Pts',(34.832241390481,-38.5190653424433,2.3550019102838));
#19705=CARTESIAN_POINT('Ctrl Pts',(33.6819332957892,-38.4642286621207,2.30266853449971));
#19706=CARTESIAN_POINT('Ctrl Pts',(32.5611023908235,-37.7910499955468,2.25033515871563));
#19707=CARTESIAN_POINT('Ctrl Pts',(31.9722786359356,-36.8013517615434,2.19800178293155));
#19708=CARTESIAN_POINT('Ctrl Pts',(31.6519194665675,-36.2628902923203,2.16952895611836));
#19709=CARTESIAN_POINT('Ctrl Pts',(31.4890387510844,-35.6307364505496,2.14105612930517));
#19710=CARTESIAN_POINT('Ctrl Pts',(31.4877390119671,-34.9992080277921,2.11258330249198));
#19711=CARTESIAN_POINT('Ctrl Pts',(31.4830375605149,-34.9969726960772,2.38741669750802));
#19712=CARTESIAN_POINT('Ctrl Pts',(31.490574858507,-35.8633368112863,2.42660964589573));
#19713=CARTESIAN_POINT('Ctrl Pts',(31.8146493000371,-36.734745074899,2.46580259428343));
#19714=CARTESIAN_POINT('Ctrl Pts',(32.3954081923274,-37.3723559095391,2.50499554267113));
#19715=CARTESIAN_POINT('Ctrl Pts',(33.1708811944992,-38.223741905896,2.55732891845522));
#19716=CARTESIAN_POINT('Ctrl Pts',(34.4040123352312,-38.6582764107548,2.60966229423931));
#19717=CARTESIAN_POINT('Ctrl Pts',(35.5419213707996,-38.4811337730552,2.66199567002339));
#19718=CARTESIAN_POINT('Ctrl Pts',(36.679830406368,-38.3039911353557,2.71432904580747));
#19719=CARTESIAN_POINT('Ctrl Pts',(37.7225173367726,-37.5151713550979,2.76666242159156));
#19720=CARTESIAN_POINT('Ctrl Pts',(38.2024884661482,-36.4683455751991,2.81899579737564));
#19721=CARTESIAN_POINT('Ctrl Pts',(38.6824595955238,-35.4215197953004,2.87132917315972));
#19722=CARTESIAN_POINT('Ctrl Pts',(38.5997149238704,-34.1166880157607,2.92366254894381));
#19723=CARTESIAN_POINT('Ctrl Pts',(37.9913534261364,-33.1388778186484,2.97599592472789));
#19724=CARTESIAN_POINT('Ctrl Pts',(37.3829919284024,-32.161067621536,3.02832930051198));
#19725=CARTESIAN_POINT('Ctrl Pts',(36.2490136045879,-31.510279006851,3.08066267629606));
#19726=CARTESIAN_POINT('Ctrl Pts',(35.0978430733873,-31.4782961743034,3.13299605208015));
#19727=CARTESIAN_POINT('Ctrl Pts',(33.9466725421867,-31.4463133417559,3.18532942786423));
#19728=CARTESIAN_POINT('Ctrl Pts',(32.7783098036,-32.0331362913458,3.23766280364832));
#19729=CARTESIAN_POINT('Ctrl Pts',(32.116595896964,-32.975660137455,3.2899961794324));
#19730=CARTESIAN_POINT('Ctrl Pts',(31.7059942452997,-33.5605078247475,3.32246968545761));
#19731=CARTESIAN_POINT('Ctrl Pts',(31.4904704191383,-34.2823130120804,3.35494319148282));
#19732=CARTESIAN_POINT('Ctrl Pts',(31.486635086556,-35.0020090496756,3.38741669750802));
#19733=CARTESIAN_POINT('Origin',(35.,-35.,4.));
#19734=CARTESIAN_POINT('',(31.4769535111774,-35.000206350087,4.38741669750802));
#19735=CARTESIAN_POINT('',(31.481143567597,-34.9970948481792,4.11258330249198));
#19736=CARTESIAN_POINT('',(31.4825,-35.,4.));
#19737=CARTESIAN_POINT('Ctrl Pts',(31.481143567597,-34.9970948481792,4.11258330249198));
#19738=CARTESIAN_POINT('Ctrl Pts',(31.4791556658517,-34.7720820979161,4.10238997204751));
#19739=CARTESIAN_POINT('Ctrl Pts',(31.4989362834408,-34.5474172520071,4.09219664160305));
#19740=CARTESIAN_POINT('Ctrl Pts',(31.5417700421341,-34.3272371560843,4.08200331115859));
#19741=CARTESIAN_POINT('Ctrl Pts',(31.7616819935963,-33.1968148899876,4.0296699353745));
#19742=CARTESIAN_POINT('Ctrl Pts',(32.5892466030323,-32.1846051588847,3.97733655959042));
#19743=CARTESIAN_POINT('Ctrl Pts',(33.6534213081659,-31.7444370513165,3.92500318380633));
#19744=CARTESIAN_POINT('Ctrl Pts',(34.7175960132996,-31.3042689437483,3.87266980802225));
#19745=CARTESIAN_POINT('Ctrl Pts',(36.0183808141308,-31.4361424597148,3.82033643223816));
#19746=CARTESIAN_POINT('Ctrl Pts',(36.9725626056516,-32.0809314753194,3.76800305645408));
#19747=CARTESIAN_POINT('Ctrl Pts',(37.9267443971724,-32.7257204909241,3.71566968066999));
#19748=CARTESIAN_POINT('Ctrl Pts',(38.5343231793827,-33.883425006167,3.66333630488591));
#19749=CARTESIAN_POINT('Ctrl Pts',(38.5228880907758,-35.0349826492465,3.61100292910183));
#19750=CARTESIAN_POINT('Ctrl Pts',(38.5114530021688,-36.186540292326,3.55866955331774));
#19751=CARTESIAN_POINT('Ctrl Pts',(37.8810040427447,-37.3319510632421,3.50633617753366));
#19752=CARTESIAN_POINT('Ctrl Pts',(36.9142060277602,-37.9576645468416,3.45400280174957));
#19753=CARTESIAN_POINT('Ctrl Pts',(35.9474080127757,-38.5833780304411,3.40166942596549));
#19754=CARTESIAN_POINT('Ctrl Pts',(34.6442609422309,-38.6893942267241,3.3493360501814));
#19755=CARTESIAN_POINT('Ctrl Pts',(33.5890370557646,-38.2281802690192,3.29700267439732));
#19756=CARTESIAN_POINT('Ctrl Pts',(32.5338131692983,-37.7669663113142,3.24466929861323));
#19757=CARTESIAN_POINT('Ctrl Pts',(31.7265124669105,-36.7385221996213,3.19233592282915));
#19758=CARTESIAN_POINT('Ctrl Pts',(31.5290920916777,-35.6039557776596,3.14000254704507));
#19759=CARTESIAN_POINT('Ctrl Pts',(31.4946136639238,-35.4058097333848,3.1308627988607));
#19760=CARTESIAN_POINT('Ctrl Pts',(31.478737062497,-35.2044268757596,3.12172305067634));
#19761=CARTESIAN_POINT('Ctrl Pts',(31.4804772106861,-35.0027703375482,3.11258330249198));
#19762=CARTESIAN_POINT('Ctrl Pts',(31.486635086556,-35.0020090496756,3.38741669750802));
#19763=CARTESIAN_POINT('Ctrl Pts',(31.4842895065774,-35.4421546120773,3.4072765672669));
#19764=CARTESIAN_POINT('Ctrl Pts',(31.5611195851562,-35.8815113110096,3.42713643702578));
#19765=CARTESIAN_POINT('Ctrl Pts',(31.7209248424069,-36.2882690753391,3.44699630678465));
#19766=CARTESIAN_POINT('Ctrl Pts',(32.1420327691713,-37.3601294244856,3.49932968256874));
#19767=CARTESIAN_POINT('Ctrl Pts',(33.1393136973855,-38.2056253801502,3.55166305835282));
#19768=CARTESIAN_POINT('Ctrl Pts',(34.2656319394155,-38.4456747746043,3.60399643413691));
#19769=CARTESIAN_POINT('Ctrl Pts',(35.3919501814454,-38.6857241690583,3.65632980992099));
#19770=CARTESIAN_POINT('Ctrl Pts',(36.647305737291,-38.3203270023018,3.70866318570508));
#19771=CARTESIAN_POINT('Ctrl Pts',(37.4688539216907,-37.5133108469912,3.76099656148916));
#19772=CARTESIAN_POINT('Ctrl Pts',(38.2904021060904,-36.7062946916805,3.81332993727324));
#19773=CARTESIAN_POINT('Ctrl Pts',(38.6781429190441,-35.4576595478158,3.86566331305733));
#19774=CARTESIAN_POINT('Ctrl Pts',(38.4582309072122,-34.3272369713982,3.91799668884141));
#19775=CARTESIAN_POINT('Ctrl Pts',(38.2383188953802,-33.1968143949805,3.9703300646255));
#19776=CARTESIAN_POINT('Ctrl Pts',(37.4107540587627,-32.1846043860099,4.02266344040958));
#19777=CARTESIAN_POINT('Ctrl Pts',(36.346579061494,-31.744436157607,4.07499681619367));
#19778=CARTESIAN_POINT('Ctrl Pts',(35.2824040642253,-31.3042679292041,4.12733019197775));
#19779=CARTESIAN_POINT('Ctrl Pts',(33.9816189063054,-31.4361414813689,4.17966356776183));
#19780=CARTESIAN_POINT('Ctrl Pts',(33.0274368528446,-32.0809306739812,4.23199694354592));
#19781=CARTESIAN_POINT('Ctrl Pts',(32.0828596573675,-32.7192293770668,4.28380352819995));
#19782=CARTESIAN_POINT('Ctrl Pts',(31.477942827805,-33.8601696083914,4.33561011285399));
#19783=CARTESIAN_POINT('Ctrl Pts',(31.4769535111774,-35.000206350087,4.38741669750802));
#19784=CARTESIAN_POINT('Origin',(35.,-35.,4.));
#19785=CARTESIAN_POINT('',(31.4861928568261,-34.9977297533801,5.38741669750802));
#19786=CARTESIAN_POINT('',(31.4875433805768,-35.0011388328632,5.11258330249198));
#19787=CARTESIAN_POINT('',(31.4825,-35.,4.));
#19788=CARTESIAN_POINT('Ctrl Pts',(31.4875433805768,-35.0011388328632,5.11258330249198));
#19789=CARTESIAN_POINT('Ctrl Pts',(31.4894886053032,-34.3463334487764,5.08305689341869));
#19790=CARTESIAN_POINT('Ctrl Pts',(31.6654108801779,-33.6905571677388,5.0535304843454));
#19791=CARTESIAN_POINT('Ctrl Pts',(32.0086473950495,-33.1388783295694,5.02400407527211));
#19792=CARTESIAN_POINT('Ctrl Pts',(32.6170087257827,-32.1610684008923,4.97167069948802));
#19793=CARTESIAN_POINT('Ctrl Pts',(33.7509867382882,-31.5102799648413,4.91933732370394));
#19794=CARTESIAN_POINT('Ctrl Pts',(34.9021569534692,-31.478297141069,4.86700394791986));
#19795=CARTESIAN_POINT('Ctrl Pts',(36.0533271686501,-31.4463143172967,4.81467057213577));
#19796=CARTESIAN_POINT('Ctrl Pts',(37.2216895865065,-32.0331371058031,4.76233719635168));
#19797=CARTESIAN_POINT('Ctrl Pts',(37.8834033114917,-32.975660693175,4.7100038205676));
#19798=CARTESIAN_POINT('Ctrl Pts',(38.5451170364769,-33.9181842805469,4.65767044478351));
#19799=CARTESIAN_POINT('Ctrl Pts',(38.7001820685911,-35.2164086667843,4.60533706899943));
#19800=CARTESIAN_POINT('Ctrl Pts',(38.2790742574276,-36.2882687216848,4.55300369321535));
#19801=CARTESIAN_POINT('Ctrl Pts',(37.8579664462641,-37.3601287765853,4.50067031743126));
#19802=CARTESIAN_POINT('Ctrl Pts',(36.8606857918229,-38.205624500149,4.44833694164718));
#19803=CARTESIAN_POINT('Ctrl Pts',(35.7343678589879,-38.4456738287057,4.39600356586309));
#19804=CARTESIAN_POINT('Ctrl Pts',(34.6080499261528,-38.6857231572625,4.34367019007901));
#19805=CARTESIAN_POINT('Ctrl Pts',(33.3526947149239,-38.3203260908123,4.29133681429492));
#19806=CARTESIAN_POINT('Ctrl Pts',(32.5311467560536,-37.5133101570419,4.23900343851084));
#19807=CARTESIAN_POINT('Ctrl Pts',(31.8696173263776,-36.863482250293,4.19686339317122));
#19808=CARTESIAN_POINT('Ctrl Pts',(31.489361712798,-35.9273155988689,4.1547233478316));
#19809=CARTESIAN_POINT('Ctrl Pts',(31.481143567597,-34.9970948481792,4.11258330249198));
#19810=CARTESIAN_POINT('Ctrl Pts',(31.4769535111774,-35.000206350087,4.38741669750802));
#19811=CARTESIAN_POINT('Ctrl Pts',(31.47694345139,-35.0117987228996,4.38794348863807));
#19812=CARTESIAN_POINT('Ctrl Pts',(31.4769958357584,-35.0233910022943,4.38847027976812));
#19813=CARTESIAN_POINT('Ctrl Pts',(31.4771109421281,-35.034982658853,4.38899707089817));
#19814=CARTESIAN_POINT('Ctrl Pts',(31.4885460338743,-36.1865406180529,4.44133044668226));
#19815=CARTESIAN_POINT('Ctrl Pts',(32.1189951663686,-37.3319517033932,4.49366382246634));
#19816=CARTESIAN_POINT('Ctrl Pts',(33.0857934467562,-37.9576653587677,4.54599719825043));
#19817=CARTESIAN_POINT('Ctrl Pts',(34.0525917271438,-38.5833790141421,4.59833057403451));
#19818=CARTESIAN_POINT('Ctrl Pts',(35.3557391554246,-38.6893952395508,4.6506639498186));
#19819=CARTESIAN_POINT('Ctrl Pts',(36.4109633315695,-38.228181155224,4.70299732560268));
#19820=CARTESIAN_POINT('Ctrl Pts',(37.4661875077144,-37.7669670708972,4.75533070138676));
#19821=CARTESIAN_POINT('Ctrl Pts',(38.2734884317233,-36.738522676835,4.80766407717085));
#19822=CARTESIAN_POINT('Ctrl Pts',(38.47090886115,-35.6039559434342,4.85999745295493));
#19823=CARTESIAN_POINT('Ctrl Pts',(38.6683292905767,-34.4693892100334,4.91233082873902));
#19824=CARTESIAN_POINT('Ctrl Pts',(38.2558692254213,-33.2287001372941,4.9646642045231));
#19825=CARTESIAN_POINT('Ctrl Pts',(37.4184571158289,-32.4381576362056,5.01699758030719));
#19826=CARTESIAN_POINT('Ctrl Pts',(36.5810450062365,-31.6476151351171,5.06933095609127));
#19827=CARTESIAN_POINT('Ctrl Pts',(35.3186808522071,-31.3072192056794,5.12166433187536));
#19828=CARTESIAN_POINT('Ctrl Pts',(34.1973516745615,-31.5695879676355,5.17399770765944));
#19829=CARTESIAN_POINT('Ctrl Pts',(33.0760224969158,-31.8319567295916,5.22633108344352));
#19830=CARTESIAN_POINT('Ctrl Pts',(32.0957282956539,-32.6970901829416,5.27866445922761));
#19831=CARTESIAN_POINT('Ctrl Pts',(31.6959886840635,-33.7771016504831,5.33099783501169));
#19832=CARTESIAN_POINT('Ctrl Pts',(31.5523400478426,-34.1652097336376,5.34980412251047));
#19833=CARTESIAN_POINT('Ctrl Pts',(31.4836621356307,-34.5810663878724,5.36861041000924));
#19834=CARTESIAN_POINT('Ctrl Pts',(31.4861928568261,-34.9977297533801,5.38741669750802));
#19835=CARTESIAN_POINT('Origin',(35.,-35.,4.));
#19836=CARTESIAN_POINT('',(31.4836965554877,-35.0029832498286,6.38741669750802));
#19837=CARTESIAN_POINT('',(31.4775766908735,-35.0013091813966,6.11258330249198));
#19838=CARTESIAN_POINT('',(31.4825,-35.,4.));
#19839=CARTESIAN_POINT('Ctrl Pts',(31.4775766908735,-35.0013091813966,6.11258330249198));
#19840=CARTESIAN_POINT('Ctrl Pts',(31.4827875611424,-33.9256166077537,6.06372381478986));
#19841=CARTESIAN_POINT('Ctrl Pts',(32.0123601793055,-32.8454783123193,6.01486432708774));
#19842=CARTESIAN_POINT('Ctrl Pts',(32.8684051290729,-32.1949568378204,5.96600483938563));
#19843=CARTESIAN_POINT('Ctrl Pts',(33.7853144981881,-31.4981835726539,5.91367146360154));
#19844=CARTESIAN_POINT('Ctrl Pts',(35.0767706429996,-31.2942900387516,5.86133808781746));
#19845=CARTESIAN_POINT('Ctrl Pts',(36.1637431566001,-31.6746930571201,5.80900471203337));
#19846=CARTESIAN_POINT('Ctrl Pts',(37.2507156702007,-32.0550960754886,5.75667133624929));
#19847=CARTESIAN_POINT('Ctrl Pts',(38.1332045525903,-33.0197956461279,5.70433796046521));
#19848=CARTESIAN_POINT('Ctrl Pts',(38.4155416055276,-34.1362640011663,5.65200458468112));
#19849=CARTESIAN_POINT('Ctrl Pts',(38.6978786584649,-35.2527323562045,5.59967120889703));
#19850=CARTESIAN_POINT('Ctrl Pts',(38.3800638819499,-36.5209694956418,5.54733783311295));
#19851=CARTESIAN_POINT('Ctrl Pts',(37.6045910926243,-37.3723552582146,5.49500445732887));
#19852=CARTESIAN_POINT('Ctrl Pts',(36.8291183032988,-38.2237410207875,5.44267108154478));
#19853=CARTESIAN_POINT('Ctrl Pts',(35.5959875011627,-38.658275406496,5.3903377057607));
#19854=CARTESIAN_POINT('Ctrl Pts',(34.4580787779894,-38.4811328174583,5.33800432997662));
#19855=CARTESIAN_POINT('Ctrl Pts',(33.3201700548161,-38.3039902284206,5.28567095419253));
#19856=CARTESIAN_POINT('Ctrl Pts',(32.2774834106055,-37.5151706646368,5.23333757840844));
#19857=CARTESIAN_POINT('Ctrl Pts',(31.7975124129806,-36.4683451720932,5.18100420262436));
#19858=CARTESIAN_POINT('Ctrl Pts',(31.5883403043411,-36.0121369913148,5.15819723591357));
#19859=CARTESIAN_POINT('Ctrl Pts',(31.486040838379,-35.5069275510188,5.13539026920277));
#19860=CARTESIAN_POINT('Ctrl Pts',(31.4875433805768,-35.0011388328632,5.11258330249198));
#19861=CARTESIAN_POINT('Ctrl Pts',(31.4861928568261,-34.9977297533801,5.38741669750802));
#19862=CARTESIAN_POINT('Ctrl Pts',(31.4907045241579,-35.7405403395491,5.42094378579333));
#19863=CARTESIAN_POINT('Ctrl Pts',(31.7215337165433,-36.4859148409341,5.45447087407864));
#19864=CARTESIAN_POINT('Ctrl Pts',(32.1573643436795,-37.081200071482,5.48799796236395));
#19865=CARTESIAN_POINT('Ctrl Pts',(32.8376646368048,-38.0103975432063,5.54033133814803));
#19866=CARTESIAN_POINT('Ctrl Pts',(34.0174502449743,-38.5739030049216,5.59266471393212));
#19867=CARTESIAN_POINT('Ctrl Pts',(35.1677586555142,-38.5190663090568,5.6449980897162));
#19868=CARTESIAN_POINT('Ctrl Pts',(36.318067066054,-38.464229613192,5.69733146550028));
#19869=CARTESIAN_POINT('Ctrl Pts',(37.4388982789643,-37.7910507597469,5.74966484128437));
#19870=CARTESIAN_POINT('Ctrl Pts',(38.0277221953511,-36.8013522549706,5.80199821706845));
#19871=CARTESIAN_POINT('Ctrl Pts',(38.6165461117379,-35.8116537501943,5.85433159285254));
#19872=CARTESIAN_POINT('Ctrl Pts',(38.6733627316013,-34.5054355940866,5.90666496863662));
#19873=CARTESIAN_POINT('Ctrl Pts',(38.172698148003,-33.4683478929687,5.9589983444207));
#19874=CARTESIAN_POINT('Ctrl Pts',(37.6720335644046,-32.4312601918508,6.01133172020479));
#19875=CARTESIAN_POINT('Ctrl Pts',(36.6138877773445,-31.6633029457227,6.06366509598888));
#19876=CARTESIAN_POINT('Ctrl Pts',(35.4726853304849,-31.5087915951115,6.11599847177296));
#19877=CARTESIAN_POINT('Ctrl Pts',(34.3314828836252,-31.3542802445004,6.16833184755705));
#19878=CARTESIAN_POINT('Ctrl Pts',(33.107223776966,-31.8132147894062,6.22066522334113));
#19879=CARTESIAN_POINT('Ctrl Pts',(32.3488108476933,-32.6798335018657,6.27299859912521));
#19880=CARTESIAN_POINT('Ctrl Pts',(31.7960968682859,-33.3114053787477,6.31113796525282));
#19881=CARTESIAN_POINT('Ctrl Pts',(31.4908012796383,-34.1595048683285,6.34927733138042));
#19882=CARTESIAN_POINT('Ctrl Pts',(31.4836965554877,-35.0029832498286,6.38741669750802));
#19883=CARTESIAN_POINT('Origin',(35.,-35.,4.));
#19884=CARTESIAN_POINT('',(31.478260520576,-34.9982347527286,7.38741669750802));
#19885=CARTESIAN_POINT('',(31.4846885160394,-34.9971888045819,7.11258330249198));
#19886=CARTESIAN_POINT('',(31.4825,-35.,4.));
#19887=CARTESIAN_POINT('',(37.6735319337713,-32.7141668369925,8.));
#19888=CARTESIAN_POINT('Ctrl Pts',(31.478260520576,-34.9982347527286,7.38741669750802));
#19889=CARTESIAN_POINT('Ctrl Pts',(31.4849542237249,-36.0376022532878,7.43461100431976));
#19890=CARTESIAN_POINT('Ctrl Pts',(31.9746244075585,-37.0822334042073,7.4818053111315));
#19891=CARTESIAN_POINT('Ctrl Pts',(32.7813940610787,-37.7364867433061,7.52899961794324));
#19892=CARTESIAN_POINT('Ctrl Pts',(33.6760142451889,-38.4619828500639,7.58133299372733));
#19893=CARTESIAN_POINT('Ctrl Pts',(34.9605528856554,-38.7074544587316,7.63366636951141));
#19894=CARTESIAN_POINT('Ctrl Pts',(36.0588772142959,-38.3607385729207,7.6859997452955));
#19895=CARTESIAN_POINT('Ctrl Pts',(37.1572015429365,-38.0140226871098,7.73833312107958));
#19896=CARTESIAN_POINT('Ctrl Pts',(38.069311559751,-37.0751193068202,7.79066649686367));
#19897=CARTESIAN_POINT('Ctrl Pts',(38.386301242806,-35.9699332359521,7.84299987264775));
#19898=CARTESIAN_POINT('Ctrl Pts',(38.703290925861,-34.864747165084,7.89533324843183));
#19899=CARTESIAN_POINT('Ctrl Pts',(38.4251602751564,-33.5932784036374,7.94766662421592));
#19900=CARTESIAN_POINT('Ctrl Pts',(37.6735319337713,-32.7141668369925,8.));
#19901=CARTESIAN_POINT('',(32.3214996650065,-32.7109746768979,8.));
#19902=CARTESIAN_POINT('Origin',(35.,-35.,8.));
#19903=CARTESIAN_POINT('Ctrl Pts',(32.3214765561793,-32.7109598296518,8.));
#19904=CARTESIAN_POINT('Ctrl Pts',(33.0392495465109,-31.8766737967152,7.95000212253756));
#19905=CARTESIAN_POINT('Ctrl Pts',(34.181330417556,-31.4010809746138,7.90000424507511));
#19906=CARTESIAN_POINT('Ctrl Pts',(35.2782977952799,-31.4881472942925,7.85000636761267));
#19907=CARTESIAN_POINT('Ctrl Pts',(36.4265066576347,-31.5792806514897,7.79767299182859));
#19908=CARTESIAN_POINT('Ctrl Pts',(37.5252889103119,-32.2868666869212,7.74533961604451));
#19909=CARTESIAN_POINT('Ctrl Pts',(38.0826699468004,-33.2944463733222,7.69300624026042));
#19910=CARTESIAN_POINT('Ctrl Pts',(38.6400509832889,-34.302026059723,7.64067286447634));
#19911=CARTESIAN_POINT('Ctrl Pts',(38.6560308035887,-35.6095993970933,7.58833948869224));
#19912=CARTESIAN_POINT('Ctrl Pts',(38.1231125366528,-36.6305184803578,7.53600611290816));
#19913=CARTESIAN_POINT('Ctrl Pts',(37.5901942697169,-37.6514375636223,7.48367273712407));
#19914=CARTESIAN_POINT('Ctrl Pts',(36.5083779155453,-38.3857023927811,7.43133936133999));
#19915=CARTESIAN_POINT('Ctrl Pts',(35.3628659911708,-38.5042959466132,7.37900598555591));
#19916=CARTESIAN_POINT('Ctrl Pts',(34.2173540667963,-38.6228895004453,7.32667260977183));
#19917=CARTESIAN_POINT('Ctrl Pts',(33.0081465722189,-38.1258117789507,7.27433923398774));
#19918=CARTESIAN_POINT('Ctrl Pts',(32.2773155686706,-37.2358335624551,7.22200585820366));
#19919=CARTESIAN_POINT('Ctrl Pts',(31.7679567703675,-36.6155557791246,7.18553167296643));
#19920=CARTESIAN_POINT('Ctrl Pts',(31.4909698285316,-35.80442618944,7.1490574877292));
#19921=CARTESIAN_POINT('Ctrl Pts',(31.4846885160394,-34.9971888045819,7.11258330249198));
#19922=CARTESIAN_POINT('Origin',(-35.,35.,10.2084234471775));
#19923=CARTESIAN_POINT('',(-39.0787305107814,35.0019482814736,0.791576552822544));
#19924=CARTESIAN_POINT('',(-39.0671617292797,34.9998409589035,0.708423447177453));
#19925=CARTESIAN_POINT('',(-39.0735,35.0000000000001,10.2084234471775));
#19926=CARTESIAN_POINT('',(-33.9479286229388,31.0647048309474,0.));
#19927=CARTESIAN_POINT('Ctrl Pts',(-39.0671617292797,34.9998409589035,0.708423447177453));
#19928=CARTESIAN_POINT('Ctrl Pts',(-39.0667162804106,35.6885579272407,0.68161580125464));
#19929=CARTESIAN_POINT('Ctrl Pts',(-38.5762700272017,37.7222374436051,0.602474779547742));
#19930=CARTESIAN_POINT('Ctrl Pts',(-35.379526836985,39.7808556694562,0.471000382056761));
#19931=CARTESIAN_POINT('Ctrl Pts',(-31.2187001848465,37.9557862959725,0.314000254704507));
#19932=CARTESIAN_POINT('Ctrl Pts',(-30.4549372314006,33.4726351387477,0.157000127352253));
#19933=CARTESIAN_POINT('Ctrl Pts',(-32.6539236935135,31.4106472544613,0.0523333757840845));
#19934=CARTESIAN_POINT('Ctrl Pts',(-33.9479286229388,31.0647048309474,0.));
#19935=CARTESIAN_POINT('',(-36.0547197101746,31.058399207452,2.73005324693302E-15));
#19936=CARTESIAN_POINT('Origin',(-35.,35.,0.));
#19937=CARTESIAN_POINT('Ctrl Pts',(-39.0787305107814,35.0019482814736,0.791576552822544));
#19938=CARTESIAN_POINT('Ctrl Pts',(-39.0794137856881,35.117415240318,0.787049082480477));
#19939=CARTESIAN_POINT('Ctrl Pts',(-39.0230450544057,36.5668924114048,0.730188236354325));
#19940=CARTESIAN_POINT('Ctrl Pts',(-37.2955092110801,39.2117686241983,0.620994014444089));
#19941=CARTESIAN_POINT('Ctrl Pts',(-32.7531819533668,39.2384377406302,0.463993887091835));
#19942=CARTESIAN_POINT('Ctrl Pts',(-30.2257196451616,35.46328448449,0.306993759739582));
#19943=CARTESIAN_POINT('Ctrl Pts',(-31.9530720002325,31.3373697401077,0.152329130708971));
#19944=CARTESIAN_POINT('Ctrl Pts',(-34.822442511108,30.7329994872565,0.0499978774624443));
#19945=CARTESIAN_POINT('Ctrl Pts',(-36.0547320440515,31.0583698407595,2.40774197454718E-15));
#19946=CARTESIAN_POINT('Origin',(-35.,35.,10.2084234471775));
#19947=CARTESIAN_POINT('',(-39.0674335213841,35.0009171557363,1.79157655282254));
#19948=CARTESIAN_POINT('',(-39.0778197532985,34.9975078784707,1.70842344717745));
#19949=CARTESIAN_POINT('',(-39.0735,35.0000000000001,10.2084234471775));
#19950=CARTESIAN_POINT('Ctrl Pts',(-39.0778197532985,34.9975078784707,1.70842344717745));
#19951=CARTESIAN_POINT('Ctrl Pts',(-39.0692748471557,36.1749702057365,1.66228272262582));
#19952=CARTESIAN_POINT('Ctrl Pts',(-37.9187924724061,38.702508200362,1.56380862229009));
#19953=CARTESIAN_POINT('Ctrl Pts',(-33.6495204180096,39.602789266723,1.41300114617028));
#19954=CARTESIAN_POINT('Ctrl Pts',(-30.4158794824773,36.4127281948833,1.25600101881803));
#19955=CARTESIAN_POINT('Ctrl Pts',(-31.2929570903083,31.9557501199225,1.09900089146578));
#19956=CARTESIAN_POINT('Ctrl Pts',(-35.4939869156159,30.2288018345407,0.942000764113521));
#19957=CARTESIAN_POINT('Ctrl Pts',(-38.6106822216958,32.3442076080298,0.811808282684081));
#19958=CARTESIAN_POINT('Ctrl Pts',(-39.0675858772087,34.3440577791618,0.733949177038725));
#19959=CARTESIAN_POINT('Ctrl Pts',(-39.0671617292797,34.9998409589035,0.708423447177453));
#19960=CARTESIAN_POINT('Ctrl Pts',(-39.0674335213841,35.0009171557363,1.79157655282255));
#19961=CARTESIAN_POINT('Ctrl Pts',(-39.0686948832473,35.6137985390812,1.76771600385165));
#19962=CARTESIAN_POINT('Ctrl Pts',(-38.6530957043657,37.569289309386,1.69152207909667));
#19963=CARTESIAN_POINT('Ctrl Pts',(-35.6435862778458,39.7534633517259,1.56299477855761));
#19964=CARTESIAN_POINT('Ctrl Pts',(-31.3902652615342,38.1590329639038,1.40599465120536));
#19965=CARTESIAN_POINT('Ctrl Pts',(-30.3738298371754,33.7318498284919,1.2489945238531));
#19966=CARTESIAN_POINT('Ctrl Pts',(-33.5057219097166,30.4418645346457,1.09199439650085));
#19967=CARTESIAN_POINT('Ctrl Pts',(-37.8485989831919,31.216140614721,0.939521739490665));
#19968=CARTESIAN_POINT('Ctrl Pts',(-39.0715157588091,33.7827238362241,0.839382458264561));
#19969=CARTESIAN_POINT('Ctrl Pts',(-39.0787305107814,35.0019482814736,0.791576552822544));
#19970=CARTESIAN_POINT('Origin',(-35.,35.,10.2084234471775));
#19971=CARTESIAN_POINT('',(-39.0758431739381,34.9967917635303,2.79157655282255));
#19972=CARTESIAN_POINT('',(-39.0728768523265,35.0035058195583,2.70842344717746));
#19973=CARTESIAN_POINT('',(-39.0735,35.0000000000001,10.2084234471775));
#19974=CARTESIAN_POINT('Ctrl Pts',(-39.0728768523265,35.0035058195583,2.70842344717746));
#19975=CARTESIAN_POINT('Ctrl Pts',(-39.075803367569,35.3398899970603,2.69528301978107));
#19976=CARTESIAN_POINT('Ctrl Pts',(-38.8850706886071,37.0126939576436,2.62980921660061));
#19977=CARTESIAN_POINT('Ctrl Pts',(-36.5844982252159,39.5275826001387,2.51200203763606));
#19978=CARTESIAN_POINT('Ctrl Pts',(-32.0977201830868,38.819215512031,2.3550019102838));
#19979=CARTESIAN_POINT('Ctrl Pts',(-30.2134435993119,34.6861220528707,2.19800178293155));
#19980=CARTESIAN_POINT('Ctrl Pts',(-32.6213194634248,30.8344843115421,2.04100165557929));
#19981=CARTESIAN_POINT('Ctrl Pts',(-37.1621781583154,30.7181077707172,1.88400152822704));
#19982=CARTESIAN_POINT('Ctrl Pts',(-38.9994901450348,33.3471191547144,1.77314212542643));
#19983=CARTESIAN_POINT('Ctrl Pts',(-39.0789665845212,34.8394779904932,1.7146160984099));
#19984=CARTESIAN_POINT('Ctrl Pts',(-39.0778197532985,34.9975078784707,1.70842344717745));
#19985=CARTESIAN_POINT('Ctrl Pts',(-39.0758431739381,34.9967917635303,2.79157655282255));
#19986=CARTESIAN_POINT('Ctrl Pts',(-39.0663194813852,36.100441948558,2.74838292522283));
#19987=CARTESIAN_POINT('Ctrl Pts',(-38.0375439399374,38.5569291706849,2.65285592183902));
#19988=CARTESIAN_POINT('Ctrl Pts',(-33.9071518161688,39.6706875589806,2.50499554267113));
#19989=CARTESIAN_POINT('Ctrl Pts',(-30.5014136769744,36.6650408935442,2.34799541531887));
#19990=CARTESIAN_POINT('Ctrl Pts',(-31.1296010783918,32.1663358219723,2.19099528796663));
#19991=CARTESIAN_POINT('Ctrl Pts',(-35.2284122688067,30.2086051339802,2.03399516061437));
#19992=CARTESIAN_POINT('Ctrl Pts',(-38.5306034134223,32.1919236036427,1.90085558223301));
#19993=CARTESIAN_POINT('Ctrl Pts',(-39.0659283364897,34.2695649347001,1.82004937963574));
#19994=CARTESIAN_POINT('Ctrl Pts',(-39.0674335213841,35.0009171557363,1.79157655282255));
#19995=CARTESIAN_POINT('Origin',(-35.,35.,10.2084234471775));
#19996=CARTESIAN_POINT('',(-39.0750714879939,35.0033643604342,3.79157655282255));
#19997=CARTESIAN_POINT('',(-39.0687106773974,34.997673386605,3.70842344717746));
#19998=CARTESIAN_POINT('',(-39.0735,35.0000000000001,10.2084234471775));
#19999=CARTESIAN_POINT('Ctrl Pts',(-39.0687106773974,34.997673386605,3.70842344717746));
#20000=CARTESIAN_POINT('Ctrl Pts',(-39.0642691067062,35.8311293539699,3.67594994115225));
#20001=CARTESIAN_POINT('Ctrl Pts',(-38.4124444982778,38.0141380355395,3.59114305934295));
#20002=CARTESIAN_POINT('Ctrl Pts',(-34.866781479659,39.7949860223284,3.45400280174958));
#20003=CARTESIAN_POINT('Ctrl Pts',(-30.9271141000824,37.5340162820022,3.29700267439732));
#20004=CARTESIAN_POINT('Ctrl Pts',(-30.6396425700269,33.0007698436185,3.14000254704507));
#20005=CARTESIAN_POINT('Ctrl Pts',(-34.2621453998186,30.2602522415144,2.98300241969281));
#20006=CARTESIAN_POINT('Ctrl Pts',(-38.1877198129624,31.6435581024348,2.83914271973695));
#20007=CARTESIAN_POINT('Ctrl Pts',(-39.064148159005,34.0001984453322,2.74761639556516));
#20008=CARTESIAN_POINT('Ctrl Pts',(-39.0728768523265,35.0035058195583,2.70842344717746));
#20009=CARTESIAN_POINT('Ctrl Pts',(-39.0750714879939,35.0033643604342,3.79157655282255));
#20010=CARTESIAN_POINT('Ctrl Pts',(-39.0773736113907,35.2639441995514,3.78138322237809));
#20011=CARTESIAN_POINT('Ctrl Pts',(-38.9368585171591,36.8598904257655,3.71885651614954));
#20012=CARTESIAN_POINT('Ctrl Pts',(-36.8334386787628,39.4326225179073,3.6039964341369));
#20013=CARTESIAN_POINT('Ctrl Pts',(-32.314250849668,38.9744674195804,3.44699630678465));
#20014=CARTESIAN_POINT('Ctrl Pts',(-30.2034000494222,34.9523692588031,3.2899961794324));
#20015=CARTESIAN_POINT('Ctrl Pts',(-32.3937064417451,30.9729820366429,3.13299605208014));
#20016=CARTESIAN_POINT('Ctrl Pts',(-36.9211012705904,30.6046604636344,2.97599592472789));
#20017=CARTESIAN_POINT('Ctrl Pts',(-38.9541946698804,33.1946779489209,2.86218942497536));
#20018=CARTESIAN_POINT('Ctrl Pts',(-39.0778583821194,34.7632599826793,2.80071630100691));
#20019=CARTESIAN_POINT('Ctrl Pts',(-39.0758431739381,34.9967917635303,2.79157655282255));
#20020=CARTESIAN_POINT('Origin',(-35.,35.,10.2084234471775));
#20021=CARTESIAN_POINT('',(-39.0676600758127,34.9986811552388,4.79157655282255));
#20022=CARTESIAN_POINT('',(-39.0799225868021,34.9997610328513,4.70842344717746));
#20023=CARTESIAN_POINT('',(-39.0735,35.0000000000001,10.2084234471775));
#20024=CARTESIAN_POINT('Ctrl Pts',(-39.0799225868021,34.9997610328513,4.70842344717746));
#20025=CARTESIAN_POINT('Ctrl Pts',(-39.0787768922257,36.3199995443189,4.65661686252342));
#20026=CARTESIAN_POINT('Ctrl Pts',(-37.6705855754179,38.9760045490164,4.5524769020853));
#20027=CARTESIAN_POINT('Ctrl Pts',(-33.1665613873943,39.4326223579625,4.3960035658631));
#20028=CARTESIAN_POINT('Ctrl Pts',(-30.2914357144823,35.9160024456566,4.23900343851084));
#20029=CARTESIAN_POINT('Ctrl Pts',(-31.6385248082081,31.5779943532675,4.08200331115859));
#20030=CARTESIAN_POINT('Ctrl Pts',(-35.9998809552364,30.3085315529294,3.92500318380634));
#20031=CARTESIAN_POINT('Ctrl Pts',(-38.7479935181635,32.6383846484188,3.80047656247929));
#20032=CARTESIAN_POINT('Ctrl Pts',(-39.0714270153063,34.4879554969268,3.72828331693633));
#20033=CARTESIAN_POINT('Ctrl Pts',(-39.0687106773974,34.997673386605,3.70842344717746));
#20034=CARTESIAN_POINT('Ctrl Pts',(-39.0676600758127,34.9986811552388,4.79157655282255));
#20035=CARTESIAN_POINT('Ctrl Pts',(-39.065407375266,35.756989657491,4.76205014374926));
#20036=CARTESIAN_POINT('Ctrl Pts',(-38.500581632009,37.8624610972284,4.68019035889188));
#20037=CARTESIAN_POINT('Ctrl Pts',(-35.1332185251462,39.7949861953461,4.54599719825043));
#20038=CARTESIAN_POINT('Ctrl Pts',(-31.0740926686951,37.7562458887763,4.38899707089817));
#20039=CARTESIAN_POINT('Ctrl Pts',(-30.5353655822401,33.2459534545604,4.23199694354592));
#20040=CARTESIAN_POINT('Ctrl Pts',(-34.0001190086845,30.3085313836444,4.07499681619366));
#20041=CARTESIAN_POINT('Ctrl Pts',(-38.0783115555367,31.4955735687615,3.92819001928588));
#20042=CARTESIAN_POINT('Ctrl Pts',(-39.0655543252915,33.9261064127185,3.83371659816217));
#20043=CARTESIAN_POINT('Ctrl Pts',(-39.0750714879939,35.0033643604342,3.79157655282255));
#20044=CARTESIAN_POINT('Origin',(-35.,35.,10.2084234471775));
#20045=CARTESIAN_POINT('',(-39.0792021698116,34.998483879503,5.79157655282255));
#20046=CARTESIAN_POINT('',(-39.0692228089002,35.0026290967949,5.70842344717746));
#20047=CARTESIAN_POINT('',(-39.0735,35.0000000000001,10.2084234471775));
#20048=CARTESIAN_POINT('Ctrl Pts',(-39.0692228089002,35.0026290967949,5.70842344717746));
#20049=CARTESIAN_POINT('Ctrl Pts',(-39.0721535526687,35.4851530378365,5.68961715967868));
#20050=CARTESIAN_POINT('Ctrl Pts',(-38.7712970745332,37.3068911247937,5.61847749639582));
#20051=CARTESIAN_POINT('Ctrl Pts',(-36.092848144401,39.6706873903976,5.49500445732886));
#20052=CARTESIAN_POINT('Ctrl Pts',(-31.7071427262397,38.4880838865661,5.33800432997662));
#20053=CARTESIAN_POINT('Ctrl Pts',(-30.2741740089879,34.1776820335287,5.18100420262436));
#20054=CARTESIAN_POINT('Ctrl Pts',(-33.0788987987297,30.6046606222411,5.02400407527212));
#20055=CARTESIAN_POINT('Ctrl Pts',(-37.6062934642105,30.9729821819491,4.86700394791985));
#20056=CARTESIAN_POINT('Ctrl Pts',(-39.073846927859,33.6392591565121,4.76181040522164));
#20057=CARTESIAN_POINT('Ctrl Pts',(-39.0799342367062,34.9863362926946,4.70895023830751));
#20058=CARTESIAN_POINT('Ctrl Pts',(-39.0799225868021,34.9997610328513,4.70842344717746));
#20059=CARTESIAN_POINT('Ctrl Pts',(-39.0792021698116,34.998483879503,5.79157655282255));
#20060=CARTESIAN_POINT('Ctrl Pts',(-39.0731676328035,36.2442079435004,5.74271706512043));
#20061=CARTESIAN_POINT('Ctrl Pts',(-37.8030025161425,38.8348894467969,5.64152420163423));
#20062=CARTESIAN_POINT('Ctrl Pts',(-33.4155017175264,39.5275827633586,5.48799796236395));
#20063=CARTESIAN_POINT('Ctrl Pts',(-30.3495579785441,36.176022571197,5.33099783501169));
#20064=CARTESIAN_POINT('Ctrl Pts',(-31.4537103860929,31.7699118586619,5.17399770765944));
#20065=CARTESIAN_POINT('Ctrl Pts',(-35.7378546268185,30.2602520705083,5.01699758030719));
#20066=CARTESIAN_POINT('Ctrl Pts',(-38.6790874120226,32.4853711659013,4.88952386202822));
#20067=CARTESIAN_POINT('Ctrl Pts',(-39.0694001203352,34.4129439352318,4.81438351953334));
#20068=CARTESIAN_POINT('Ctrl Pts',(-39.0676600758127,34.9986811552388,4.79157655282255));
#20069=CARTESIAN_POINT('Origin',(-35.,35.,10.2084234471775));
#20070=CARTESIAN_POINT('',(-39.070966199943,35.0032555604945,6.79157655282255));
#20071=CARTESIAN_POINT('',(-39.0721136942453,34.9965451882256,6.70842344717746));
#20072=CARTESIAN_POINT('',(-39.0735,35.0000000000001,10.2084234471775));
#20073=CARTESIAN_POINT('Ctrl Pts',(-39.0721136942453,34.9965451882256,6.70842344717746));
#20074=CARTESIAN_POINT('Ctrl Pts',(-39.0638859499781,35.9733493601025,6.67028408104985));
#20075=CARTESIAN_POINT('Ctrl Pts',(-38.2252019424137,38.3031815231405,6.57981133913817));
#20076=CARTESIAN_POINT('Ctrl Pts',(-34.3564137457339,39.7534631780217,6.4370052214424));
#20077=CARTESIAN_POINT('Ctrl Pts',(-30.6802037555765,37.0854262040492,6.28000509409013));
#20078=CARTESIAN_POINT('Ctrl Pts',(-30.8775960516807,32.5473632088007,6.12300496673789));
#20079=CARTESIAN_POINT('Ctrl Pts',(-34.7715877393978,30.2086053071985,5.96600483938563));
#20080=CARTESIAN_POINT('Ctrl Pts',(-38.3794219899756,31.9318288223888,5.82781099953215));
#20081=CARTESIAN_POINT('Ctrl Pts',(-39.0639979975134,34.142404941861,5.74195053546276));
#20082=CARTESIAN_POINT('Ctrl Pts',(-39.0692228089002,35.0026290967949,5.70842344717746));
#20083=CARTESIAN_POINT('Ctrl Pts',(-39.070966199943,35.0032555604945,6.79157655282255));
#20084=CARTESIAN_POINT('Ctrl Pts',(-39.0741290517156,35.409727295843,6.77571736227569));
#20085=CARTESIAN_POINT('Ctrl Pts',(-38.8328829256554,37.1538415310843,6.70752479594475));
#20086=CARTESIAN_POINT('Ctrl Pts',(-36.3504796357983,39.6027894460767,6.58699885382972));
#20087=CARTESIAN_POINT('Ctrl Pts',(-31.905897053523,38.6655398223873,6.42999872647746));
#20088=CARTESIAN_POINT('Ctrl Pts',(-30.2358031812474,34.4413383659989,6.27299859912522));
#20089=CARTESIAN_POINT('Ctrl Pts',(-32.8378217627235,30.7181076142107,6.11599847177296));
#20090=CARTESIAN_POINT('Ctrl Pts',(-37.3786806229274,30.8344841622903,5.95899834442071));
#20091=CARTESIAN_POINT('Ctrl Pts',(-39.0372095034026,33.4874666211437,5.85085770477057));
#20092=CARTESIAN_POINT('Ctrl Pts',(-39.0796312227382,34.9099134465561,5.79505044090451));
#20093=CARTESIAN_POINT('Ctrl Pts',(-39.0792021698116,34.998483879503,5.79157655282255));
#20094=CARTESIAN_POINT('Origin',(-35.,35.,10.2084234471775));
#20095=CARTESIAN_POINT('',(-39.0691248821302,34.9959228837483,7.79157655282255));
#20096=CARTESIAN_POINT('',(-39.0784090602678,35.0020440536087,7.70842344717746));
#20097=CARTESIAN_POINT('',(-39.0735,35.0000000000001,10.2084234471775));
#20098=CARTESIAN_POINT('',(-36.0520713770612,31.0647048309474,8.));
#20099=CARTESIAN_POINT('Ctrl Pts',(-36.0520713770612,31.0647048309474,8.));
#20100=CARTESIAN_POINT('Ctrl Pts',(-37.3460763064866,31.4106472544613,7.94766662421592));
#20101=CARTESIAN_POINT('Ctrl Pts',(-38.8056938328118,32.7793309690615,7.87819214182344));
#20102=CARTESIAN_POINT('Ctrl Pts',(-39.0721267560147,34.5563414191054,7.80871765943095));
#20103=CARTESIAN_POINT('Ctrl Pts',(-39.0691248821302,34.9959228837483,7.79157655282255));
#20104=CARTESIAN_POINT('',(-33.9452804362612,31.0583992034428,8.));
#20105=CARTESIAN_POINT('Origin',(-35.,35.,8.));
#20106=CARTESIAN_POINT('Ctrl Pts',(-33.9452681066883,31.058369845356,8.));
#20107=CARTESIAN_POINT('Ctrl Pts',(-35.1775577544271,30.7329993831125,7.95000212253756));
#20108=CARTESIAN_POINT('Ctrl Pts',(-37.9028280459028,31.3070187859893,7.85280993826337));
#20109=CARTESIAN_POINT('Ctrl Pts',(-39.0706571061612,33.7983874965128,7.7556177539892));
#20110=CARTESIAN_POINT('Ctrl Pts',(-39.0784090602678,35.0020440536087,7.70842344717747));
#20111=CARTESIAN_POINT('Origin',(35.,35.,10.2084234471775));
#20112=CARTESIAN_POINT('',(30.9212698233586,35.0019483146883,0.791576552822542));
#20113=CARTESIAN_POINT('',(30.9328374281389,34.9998406908479,0.708423447177449));
#20114=CARTESIAN_POINT('',(30.9265,35.0000000000001,10.2084234471775));
#20115=CARTESIAN_POINT('',(36.0520713770613,31.0647048309474,0.));
#20116=CARTESIAN_POINT('Ctrl Pts',(30.9328374281389,34.9998406908479,0.708423447177449));
#20117=CARTESIAN_POINT('Ctrl Pts',(30.9332828479214,35.688557610158,0.681615801254637));
#20118=CARTESIAN_POINT('Ctrl Pts',(31.423729103703,37.7222371568615,0.602474779547742));
#20119=CARTESIAN_POINT('Ctrl Pts',(34.620473026815,39.7808594262888,0.47100038205676));
#20120=CARTESIAN_POINT('Ctrl Pts',(38.7813013396977,37.9557820285754,0.314000254704507));
#20121=CARTESIAN_POINT('Ctrl Pts',(39.5450610063768,33.4726465453437,0.157000127352254));
#20122=CARTESIAN_POINT('Ctrl Pts',(37.3460763064866,31.4106472544613,0.0523333757840845));
#20123=CARTESIAN_POINT('Ctrl Pts',(36.0520713770613,31.0647048309474,0.));
#20124=CARTESIAN_POINT('',(33.9452806327216,31.0583991975554,1.9516645121422E-15));
#20125=CARTESIAN_POINT('Origin',(35.,35.,0.));
#20126=CARTESIAN_POINT('Ctrl Pts',(30.9212698233586,35.0019483146883,0.791576552822542));
#20127=CARTESIAN_POINT('Ctrl Pts',(30.9205865489415,35.1174152630019,0.787049082480475));
#20128=CARTESIAN_POINT('Ctrl Pts',(30.9769552830328,36.5668922956884,0.730188236354323));
#20129=CARTESIAN_POINT('Ctrl Pts',(32.7044910542971,39.2117680815463,0.620994014444087));
#20130=CARTESIAN_POINT('Ctrl Pts',(37.246817707304,39.2384377086451,0.463993887091833));
#20131=CARTESIAN_POINT('Ctrl Pts',(39.7742802645754,35.4632838929154,0.30699375973958));
#20132=CARTESIAN_POINT('Ctrl Pts',(38.0469271024438,31.3373709383794,0.152329130708969));
#20133=CARTESIAN_POINT('Ctrl Pts',(35.1775581103468,30.7329992432291,0.0499978774624438));
#20134=CARTESIAN_POINT('Ctrl Pts',(33.9452683089267,31.0583698510224,2.42915496745377E-15));
#20135=CARTESIAN_POINT('Origin',(35.,35.,10.2084234471775));
#20136=CARTESIAN_POINT('',(30.9325668217157,35.0009171562606,1.79157655282254));
#20137=CARTESIAN_POINT('',(30.9221793985577,34.9975078813789,1.70842344717745));
#20138=CARTESIAN_POINT('',(30.9265,35.0000000000001,10.2084234471775));
#20139=CARTESIAN_POINT('Ctrl Pts',(30.9221793985577,34.9975078813789,1.70842344717745));
#20140=CARTESIAN_POINT('Ctrl Pts',(30.9307243035611,36.174970446985,1.66228272262581));
#20141=CARTESIAN_POINT('Ctrl Pts',(32.0812069040633,38.7025089358584,1.56380862229009));
#20142=CARTESIAN_POINT('Ctrl Pts',(36.3504798927025,39.6027903023767,1.41300114617028));
#20143=CARTESIAN_POINT('Ctrl Pts',(39.5841214241815,36.41272834745,1.25600101881803));
#20144=CARTESIAN_POINT('Ctrl Pts',(38.7070437601939,31.9557497473198,1.09900089146578));
#20145=CARTESIAN_POINT('Ctrl Pts',(34.5060128656572,30.2288003607244,0.942000764113522));
#20146=CARTESIAN_POINT('Ctrl Pts',(31.3893171307454,32.344207693053,0.811808282684079));
#20147=CARTESIAN_POINT('Ctrl Pts',(30.9324133079056,34.3440575577889,0.733949177038721));
#20148=CARTESIAN_POINT('Ctrl Pts',(30.9328374281389,34.9998406908479,0.708423447177449));
#20149=CARTESIAN_POINT('Ctrl Pts',(30.9325668217157,35.0009171562606,1.79157655282254));
#20150=CARTESIAN_POINT('Ctrl Pts',(30.9313054599248,35.6137984881563,1.76771600385165));
#20151=CARTESIAN_POINT('Ctrl Pts',(31.3469046036967,37.5692890939049,1.69152207909667));
#20152=CARTESIAN_POINT('Ctrl Pts',(34.3564137772933,39.7534629455386,1.56299477855761));
#20153=CARTESIAN_POINT('Ctrl Pts',(38.6097344321268,38.159032706872,1.40599465120535));
#20154=CARTESIAN_POINT('Ctrl Pts',(39.6261697761982,33.7318499178854,1.2489945238531));
#20155=CARTESIAN_POINT('Ctrl Pts',(36.4942779564007,30.441864951573,1.09199439650085));
#20156=CARTESIAN_POINT('Ctrl Pts',(32.1514012728307,31.2161408778184,0.939521739490661));
#20157=CARTESIAN_POINT('Ctrl Pts',(30.9284845701608,33.7827239806345,0.839382458264559));
#20158=CARTESIAN_POINT('Ctrl Pts',(30.9212698233586,35.0019483146883,0.791576552822542));
#20159=CARTESIAN_POINT('Origin',(35.,35.,10.2084234471775));
#20160=CARTESIAN_POINT('',(30.9241571699662,34.9967917637985,2.79157655282254));
#20161=CARTESIAN_POINT('',(30.9271222988705,35.0035058204319,2.70842344717745));
#20162=CARTESIAN_POINT('',(30.9265,35.0000000000001,10.2084234471775));
#20163=CARTESIAN_POINT('Ctrl Pts',(30.9271222988705,35.0035058204319,2.70842344717745));
#20164=CARTESIAN_POINT('Ctrl Pts',(30.9241957830228,35.3398900680519,2.69528301978107));
#20165=CARTESIAN_POINT('Ctrl Pts',(31.1149285017256,37.0126943772598,2.62980921660061));
#20166=CARTESIAN_POINT('Ctrl Pts',(33.415501444059,39.52758354292,2.51200203763605));
#20167=CARTESIAN_POINT('Ctrl Pts',(37.902280422705,38.8192163097165,2.3550019102838));
#20168=CARTESIAN_POINT('Ctrl Pts',(39.7865573966804,34.6861219842625,2.19800178293155));
#20169=CARTESIAN_POINT('Ctrl Pts',(37.3786810353442,30.8344834494167,2.0410016555793));
#20170=CARTESIAN_POINT('Ctrl Pts',(32.8378213856151,30.7181068667712,1.88400152822704));
#20171=CARTESIAN_POINT('Ctrl Pts',(31.0005090266209,33.347118822167,1.77314212542643));
#20172=CARTESIAN_POINT('Ctrl Pts',(30.9210325674879,34.839477961413,1.7146160984099));
#20173=CARTESIAN_POINT('Ctrl Pts',(30.9221793985577,34.9975078813789,1.70842344717745));
#20174=CARTESIAN_POINT('Ctrl Pts',(30.9241571699662,34.9967917637985,2.79157655282254));
#20175=CARTESIAN_POINT('Ctrl Pts',(30.9336808617147,36.100441855715,2.74838292522282));
#20176=CARTESIAN_POINT('Ctrl Pts',(31.9624563163556,38.5569288706128,2.65285592183902));
#20177=CARTESIAN_POINT('Ctrl Pts',(36.0928480916297,39.6706871647746,2.50499554267113));
#20178=CARTESIAN_POINT('Ctrl Pts',(39.4985859434327,36.6650407532663,2.34799541531887));
#20179=CARTESIAN_POINT('Ctrl Pts',(38.8703985950797,32.1663360606625,2.19099528796662));
#20180=CARTESIAN_POINT('Ctrl Pts',(34.7715877503781,30.208605539026,2.03399516061437));
#20181=CARTESIAN_POINT('Ctrl Pts',(31.4693968846214,32.1919238394657,1.90085558223301));
#20182=CARTESIAN_POINT('Ctrl Pts',(30.9340720065237,34.2695649966187,1.82004937963573));
#20183=CARTESIAN_POINT('Ctrl Pts',(30.9325668217157,35.0009171562606,1.79157655282254));
#20184=CARTESIAN_POINT('Origin',(35.,35.,10.2084234471775));
#20185=CARTESIAN_POINT('',(30.9249288558452,35.0033643601501,3.79157655282254));
#20186=CARTESIAN_POINT('',(30.9312884745882,34.9976733861211,3.70842344717745));
#20187=CARTESIAN_POINT('',(30.9265,35.0000000000001,10.2084234471775));
#20188=CARTESIAN_POINT('Ctrl Pts',(30.9312884745882,34.9976733861211,3.70842344717745));
#20189=CARTESIAN_POINT('Ctrl Pts',(30.935730046206,35.8311295271992,3.67594994115225));
#20190=CARTESIAN_POINT('Ctrl Pts',(31.587554790492,38.0141386637623,3.59114305934295));
#20191=CARTESIAN_POINT('Ctrl Pts',(35.1332185480963,39.7949870216991,3.45400280174957));
#20192=CARTESIAN_POINT('Ctrl Pts',(39.0728867488228,37.5340168101838,3.29700267439732));
#20193=CARTESIAN_POINT('Ctrl Pts',(39.360358338736,33.0007694268683,3.14000254704507));
#20194=CARTESIAN_POINT('Ctrl Pts',(35.7378547540399,30.2602512537625,2.98300241969282));
#20195=CARTESIAN_POINT('Ctrl Pts',(31.8122795225231,31.6435574026667,2.83914271973694));
#20196=CARTESIAN_POINT('Ctrl Pts',(30.9358509939969,34.0001982370698,2.74761639556516));
#20197=CARTESIAN_POINT('Ctrl Pts',(30.9271222988705,35.0035058204319,2.70842344717745));
#20198=CARTESIAN_POINT('Ctrl Pts',(30.9249288558452,35.0033643601501,3.79157655282255));
#20199=CARTESIAN_POINT('Ctrl Pts',(30.9226267326427,35.2639441772806,3.78138322237808));
#20200=CARTESIAN_POINT('Ctrl Pts',(31.0631418150181,36.8598902688347,3.71885651614953));
#20201=CARTESIAN_POINT('Ctrl Pts',(33.1665614759356,39.4326221439007,3.60399643413691));
#20202=CARTESIAN_POINT('Ctrl Pts',(37.6857489237188,38.9744670842276,3.44699630678464));
#20203=CARTESIAN_POINT('Ctrl Pts',(39.7965995458586,34.9523692628263,3.2899961794324));
#20204=CARTESIAN_POINT('Ctrl Pts',(37.6062933383462,30.9729823764193,3.13299605208014));
#20205=CARTESIAN_POINT('Ctrl Pts',(33.078898891504,30.6046608345122,2.97599592472789));
#20206=CARTESIAN_POINT('Ctrl Pts',(31.0458056637607,33.1946781012295,2.86218942497536));
#20207=CARTESIAN_POINT('Ctrl Pts',(30.9221419619551,34.7632600026498,2.80071630100691));
#20208=CARTESIAN_POINT('Ctrl Pts',(30.9241571699662,34.9967917637985,2.79157655282254));
#20209=CARTESIAN_POINT('Origin',(35.,35.,10.2084234471775));
#20210=CARTESIAN_POINT('',(30.9323402673974,34.9986811553562,4.79157655282255));
#20211=CARTESIAN_POINT('',(30.920076562846,34.9997610327988,4.70842344717745));
#20212=CARTESIAN_POINT('',(30.9265,35.0000000000001,10.2084234471775));
#20213=CARTESIAN_POINT('Ctrl Pts',(30.920076562846,34.9997610327988,4.70842344717745));
#20214=CARTESIAN_POINT('Ctrl Pts',(30.9212222576611,36.3199998194329,4.65661686252342));
#20215=CARTESIAN_POINT('Ctrl Pts',(32.3294138679696,38.9760053777146,4.5524769020853));
#20216=CARTESIAN_POINT('Ctrl Pts',(36.833438994737,39.4326232818222,4.39600356586309));
#20217=CARTESIAN_POINT('Ctrl Pts',(39.7085652668935,35.9160026365752,4.23900343851085));
#20218=CARTESIAN_POINT('Ctrl Pts',(38.3614758924016,31.5779936400392,4.08200331115859));
#20219=CARTESIAN_POINT('Ctrl Pts',(34.0001188363665,30.3085305751198,3.92500318380634));
#20220=CARTESIAN_POINT('Ctrl Pts',(31.2520057006646,32.6383841561994,3.80047656247929));
#20221=CARTESIAN_POINT('Ctrl Pts',(30.9285721361126,34.4879553902047,3.72828331693633));
#20222=CARTESIAN_POINT('Ctrl Pts',(30.9312884745882,34.9976733861211,3.70842344717745));
#20223=CARTESIAN_POINT('Ctrl Pts',(30.9323402673974,34.9986811553562,4.79157655282255));
#20224=CARTESIAN_POINT('Ctrl Pts',(30.9345929677557,35.7569895936223,4.76205014374926));
#20225=CARTESIAN_POINT('Ctrl Pts',(31.4994186633631,37.8624608556942,4.68019035889188));
#20226=CARTESIAN_POINT('Ctrl Pts',(34.86678148609,39.7949857907703,4.54599719825042));
#20227=CARTESIAN_POINT('Ctrl Pts',(38.9259070000539,37.7562456562111,4.38899707089817));
#20228=CARTESIAN_POINT('Ctrl Pts',(39.4646340410498,33.2459536025622,4.23199694354592));
#20229=CARTESIAN_POINT('Ctrl Pts',(35.9998809069499,30.3085317794917,4.07499681619366));
#20230=CARTESIAN_POINT('Ctrl Pts',(31.9216887041993,31.4955738644524,3.92819001928588));
#20231=CARTESIAN_POINT('Ctrl Pts',(30.9344460177445,33.9261065033295,3.83371659816217));
#20232=CARTESIAN_POINT('Ctrl Pts',(30.9249288558452,35.0033643601501,3.79157655282255));
#20233=CARTESIAN_POINT('Origin',(35.,35.,10.2084234471775));
#20234=CARTESIAN_POINT('',(30.9207981741727,34.9984838800189,5.79157655282254));
#20235=CARTESIAN_POINT('',(30.93077634299,35.0026290974327,5.70842344717745));
#20236=CARTESIAN_POINT('',(30.9265,35.0000000000001,10.2084234471775));
#20237=CARTESIAN_POINT('Ctrl Pts',(30.93077634299,35.0026290974327,5.70842344717745));
#20238=CARTESIAN_POINT('Ctrl Pts',(30.9278455986019,35.4851531389532,5.68961715967867));
#20239=CARTESIAN_POINT('Ctrl Pts',(31.2287021394076,37.3068916052531,5.61847749639582));
#20240=CARTESIAN_POINT('Ctrl Pts',(33.9071516278456,39.6706883641509,5.49500445732887));
#20241=CARTESIAN_POINT('Ctrl Pts',(38.2928579600589,38.4880846134226,5.33800432997661));
#20242=CARTESIAN_POINT('Ctrl Pts',(39.72582697599,34.1776818622125,5.18100420262437));
#20243=CARTESIAN_POINT('Ctrl Pts',(36.9211016016709,30.6046597061106,5.0240040752721));
#20244=CARTESIAN_POINT('Ctrl Pts',(32.3937059925777,30.9729813426439,4.86700394791986));
#20245=CARTESIAN_POINT('Ctrl Pts',(30.9261522230555,33.6392588729013,4.76181040522164));
#20246=CARTESIAN_POINT('Ctrl Pts',(30.9200649129395,34.986336289844,4.7089502383075));
#20247=CARTESIAN_POINT('Ctrl Pts',(30.920076562846,34.9997610327988,4.70842344717745));
#20248=CARTESIAN_POINT('Ctrl Pts',(30.9207981741727,34.9984838800189,5.79157655282254));
#20249=CARTESIAN_POINT('Ctrl Pts',(30.9268327105953,36.2442078390725,5.74271706512043));
#20250=CARTESIAN_POINT('Ctrl Pts',(32.1969977207135,38.8348891225654,5.64152420163423));
#20251=CARTESIAN_POINT('Ctrl Pts',(36.5844981485848,39.5275823816942,5.48799796236394));
#20252=CARTESIAN_POINT('Ctrl Pts',(39.6504416291735,36.1760224717832,5.33099783501169));
#20253=CARTESIAN_POINT('Ctrl Pts',(38.5462893146292,31.7699121313011,5.17399770765944));
#20254=CARTESIAN_POINT('Ctrl Pts',(34.2621454354683,30.2602524703801,5.01699758030718));
#20255=CARTESIAN_POINT('Ctrl Pts',(31.3209128983978,32.4853713780877,4.88952386202822));
#20256=CARTESIAN_POINT('Ctrl Pts',(30.9306002230203,34.4129439847737,4.81438351953334));
#20257=CARTESIAN_POINT('Ctrl Pts',(30.9323402673974,34.9986811553562,4.79157655282255));
#20258=CARTESIAN_POINT('Origin',(35.,35.,10.2084234471775));
#20259=CARTESIAN_POINT('',(30.9290341434093,35.0032555560525,6.79157655282255));
#20260=CARTESIAN_POINT('',(30.9278854598697,34.9965452008231,6.70842344717745));
#20261=CARTESIAN_POINT('',(30.9265,35.0000000000001,10.2084234471775));
#20262=CARTESIAN_POINT('Ctrl Pts',(30.9278854598697,34.9965452008231,6.70842344717745));
#20263=CARTESIAN_POINT('Ctrl Pts',(30.9361132054557,35.973349573232,6.67028408104985));
#20264=CARTESIAN_POINT('Ctrl Pts',(31.7747973816342,38.3031821914714,6.57981133913817));
#20265=CARTESIAN_POINT('Ctrl Pts',(35.6435863904507,39.7534641813021,6.43700522144238));
#20266=CARTESIAN_POINT('Ctrl Pts',(39.3197971438036,37.085426632005,6.28000509409014));
#20267=CARTESIAN_POINT('Ctrl Pts',(39.122404807981,32.5473627011697,6.12300496673788));
#20268=CARTESIAN_POINT('Ctrl Pts',(35.2284123079944,30.2086043066787,5.96600483938564));
#20269=CARTESIAN_POINT('Ctrl Pts',(31.6205773057362,31.9318281835565,5.82781099953215));
#20270=CARTESIAN_POINT('Ctrl Pts',(30.9360011554815,34.1424047633691,5.74195053546276));
#20271=CARTESIAN_POINT('Ctrl Pts',(30.93077634299,35.0026290974327,5.70842344717745));
#20272=CARTESIAN_POINT('Ctrl Pts',(30.9290341434093,35.0032555560525,6.79157655282255));
#20273=CARTESIAN_POINT('Ctrl Pts',(30.9258712893501,35.4097272653281,6.77571736227569));
#20274=CARTESIAN_POINT('Ctrl Pts',(31.167117385295,37.1538413864501,6.70752479594475));
#20275=CARTESIAN_POINT('Ctrl Pts',(33.6495204900336,39.6027890266495,6.58699885382972));
#20276=CARTESIAN_POINT('Ctrl Pts',(38.0941026784935,38.6655395297167,6.42999872647747));
#20277=CARTESIAN_POINT('Ctrl Pts',(39.7641964207046,34.4413384042963,6.27299859912521));
#20278=CARTESIAN_POINT('Ctrl Pts',(37.1621780526355,30.7181079801836,6.11599847177296));
#20279=CARTESIAN_POINT('Ctrl Pts',(32.6213195789955,30.8344845112897,5.95899834442071));
#20280=CARTESIAN_POINT('Ctrl Pts',(30.9627908371619,33.4874667488915,5.85085770477057));
#20281=CARTESIAN_POINT('Ctrl Pts',(30.9203691212877,34.9099134545334,5.79505044090451));
#20282=CARTESIAN_POINT('Ctrl Pts',(30.9207981741727,34.9984838800189,5.79157655282254));
#20283=CARTESIAN_POINT('Origin',(35.,35.,10.2084234471775));
#20284=CARTESIAN_POINT('',(30.9308749498806,34.995920959377,7.79157655282255));
#20285=CARTESIAN_POINT('',(30.9215901961247,35.0020443570103,7.70842344717745));
#20286=CARTESIAN_POINT('',(30.9265,35.0000000000001,10.2084234471775));
#20287=CARTESIAN_POINT('',(33.9479286229388,31.0647048309474,8.));
#20288=CARTESIAN_POINT('Ctrl Pts',(33.9479286229388,31.0647048309474,8.));
#20289=CARTESIAN_POINT('Ctrl Pts',(32.6539236935135,31.4106472544613,7.94766662421592));
#20290=CARTESIAN_POINT('Ctrl Pts',(31.1943056926496,32.7793278989778,7.87819214182343));
#20291=CARTESIAN_POINT('Ctrl Pts',(30.927873001558,34.5563391849396,7.80871765943095));
#20292=CARTESIAN_POINT('Ctrl Pts',(30.9308749498806,34.995920959377,7.79157655282255));
#20293=CARTESIAN_POINT('',(36.0547204053665,31.0583992220146,8.));
#20294=CARTESIAN_POINT('Origin',(35.,35.,8.));
#20295=CARTESIAN_POINT('Ctrl Pts',(36.0547327596422,31.0583698145405,8.));
#20296=CARTESIAN_POINT('Ctrl Pts',(34.8224437745751,30.7329999802434,7.95000212253756));
#20297=CARTESIAN_POINT('Ctrl Pts',(32.0971699315749,31.3070160119469,7.85280993826337));
#20298=CARTESIAN_POINT('Ctrl Pts',(30.9293418770678,33.7983871843493,7.75561775398919));
#20299=CARTESIAN_POINT('Ctrl Pts',(30.9215901961247,35.0020443570103,7.70842344717745));
#20300=CARTESIAN_POINT('Origin',(-35.,-35.,10.2084234471775));
#20301=CARTESIAN_POINT('',(-39.0787307957508,-34.998051746757,0.791576552822544));
#20302=CARTESIAN_POINT('',(-39.0671620604938,-35.0001591466914,0.708423447177451));
#20303=CARTESIAN_POINT('',(-39.0735,-34.9999999999999,10.2084234471775));
#20304=CARTESIAN_POINT('',(-33.9479286229388,-38.9352951690526,0.));
#20305=CARTESIAN_POINT('Ctrl Pts',(-39.0671620604938,-35.0001591466914,
0.708423447177451));
#20306=CARTESIAN_POINT('Ctrl Pts',(-39.0667166230717,-34.3114421978074,
0.681615801254639));
#20307=CARTESIAN_POINT('Ctrl Pts',(-38.5762703689089,-32.2777626699106,
0.602474779547742));
#20308=CARTESIAN_POINT('Ctrl Pts',(-35.3795268907121,-30.2191428513895,
0.471000382056761));
#20309=CARTESIAN_POINT('Ctrl Pts',(-31.2186995847689,-32.0442153857854,
0.314000254704507));
#20310=CARTESIAN_POINT('Ctrl Pts',(-30.4549379250093,-36.5273603729133,
0.157000127352253));
#20311=CARTESIAN_POINT('Ctrl Pts',(-32.6539236935135,-38.5893527455387,
0.0523333757840845));
#20312=CARTESIAN_POINT('Ctrl Pts',(-33.9479286229388,-38.9352951690526,
0.));
#20313=CARTESIAN_POINT('',(-36.0547200012553,-38.9416007855471,4.26113251110999E-15));
#20314=CARTESIAN_POINT('Origin',(-35.,-35.,0.));
#20315=CARTESIAN_POINT('Ctrl Pts',(-39.0787307957508,-34.9980517467571,
0.791576552822544));
#20316=CARTESIAN_POINT('Ctrl Pts',(-39.0794140710738,-34.8825847789344,
0.787049082480477));
#20317=CARTESIAN_POINT('Ctrl Pts',(-39.0230453421645,-33.4331074898667,
0.730188236354326));
#20318=CARTESIAN_POINT('Ctrl Pts',(-37.2955094371433,-30.7882309135474,
0.620994014444089));
#20319=CARTESIAN_POINT('Ctrl Pts',(-32.7531816644513,-30.7615622313046,
0.463993887091836));
#20320=CARTESIAN_POINT('Ctrl Pts',(-30.2257195673566,-34.5367150123096,
0.306993759739581));
#20321=CARTESIAN_POINT('Ctrl Pts',(-31.9530712365814,-38.6626312798268,
0.152329130708972));
#20322=CARTESIAN_POINT('Ctrl Pts',(-34.8224430395506,-39.2670003060384,
0.0499978774624443));
#20323=CARTESIAN_POINT('Ctrl Pts',(-36.0547323436802,-38.9416301693299,
2.36437388764776E-15));
#20324=CARTESIAN_POINT('Origin',(-35.,-35.,10.2084234471775));
#20325=CARTESIAN_POINT('',(-39.0674338139571,-34.9990828447087,1.79157655282254));
#20326=CARTESIAN_POINT('',(-39.0778200867196,-35.0024921203811,1.70842344717745));
#20327=CARTESIAN_POINT('',(-39.0735,-34.9999999999999,10.2084234471775));
#20328=CARTESIAN_POINT('Ctrl Pts',(-39.0778200867196,-35.0024921203811,
1.70842344717745));
#20329=CARTESIAN_POINT('Ctrl Pts',(-39.0692751810275,-33.8250296994275,
1.66228272262581));
#20330=CARTESIAN_POINT('Ctrl Pts',(-37.9187927175433,-31.297491510544,1.56380862229009));
#20331=CARTESIAN_POINT('Ctrl Pts',(-33.6495202958365,-30.3972103260493,
1.41300114617028));
#20332=CARTESIAN_POINT('Ctrl Pts',(-30.4158791260905,-33.5872717453,1.25600101881803));
#20333=CARTESIAN_POINT('Ctrl Pts',(-31.2929567559004,-38.0442500262742,
1.09900089146578));
#20334=CARTESIAN_POINT('Ctrl Pts',(-35.4939870016774,-39.7711987453336,
0.942000764113521));
#20335=CARTESIAN_POINT('Ctrl Pts',(-38.6106824762136,-37.6557923579424,
0.81180828268408));
#20336=CARTESIAN_POINT('Ctrl Pts',(-39.0675861975231,-35.6559423079101,
0.733949177038723));
#20337=CARTESIAN_POINT('Ctrl Pts',(-39.0671620604938,-35.0001591466914,
0.708423447177451));
#20338=CARTESIAN_POINT('Ctrl Pts',(-39.0674338139571,-34.9990828447087,
1.79157655282254));
#20339=CARTESIAN_POINT('Ctrl Pts',(-39.0686951758822,-34.3862014174905,
1.76771600385165));
#20340=CARTESIAN_POINT('Ctrl Pts',(-38.6530959670617,-32.4307105068614,
1.69152207909667));
#20341=CARTESIAN_POINT('Ctrl Pts',(-35.6435863248602,-30.2465363019221,
1.56299477855761));
#20342=CARTESIAN_POINT('Ctrl Pts',(-31.3902650003177,-31.8409668168855,
1.40599465120536));
#20343=CARTESIAN_POINT('Ctrl Pts',(-30.3738295074692,-36.2681502477922,
1.2489945238531));
#20344=CARTESIAN_POINT('Ctrl Pts',(-33.5057217955833,-39.5581358207848,
1.09199439650085));
#20345=CARTESIAN_POINT('Ctrl Pts',(-37.8485992014502,-38.7838596097918,
0.939521739490664));
#20346=CARTESIAN_POINT('Ctrl Pts',(-39.0715160393823,-36.2172762868091,
0.839382458264562));
#20347=CARTESIAN_POINT('Ctrl Pts',(-39.0787307957508,-34.9980517467571,
0.791576552822544));
#20348=CARTESIAN_POINT('Origin',(-35.,-35.,10.2084234471775));
#20349=CARTESIAN_POINT('',(-39.0758434671966,-35.0032082366984,2.79157655282255));
#20350=CARTESIAN_POINT('',(-39.0728771860086,-34.996494180098,2.70842344717745));
#20351=CARTESIAN_POINT('',(-39.0735,-34.9999999999999,10.2084234471775));
#20352=CARTESIAN_POINT('Ctrl Pts',(-39.0728771860086,-34.996494180098,2.70842344717745));
#20353=CARTESIAN_POINT('Ctrl Pts',(-39.075803701489,-34.6601099750312,2.69528301978107));
#20354=CARTESIAN_POINT('Ctrl Pts',(-38.8850710069041,-32.9873058773963,
2.62980921660061));
#20355=CARTESIAN_POINT('Ctrl Pts',(-36.5844983552314,-30.4724170292356,
2.51200203763606));
#20356=CARTESIAN_POINT('Ctrl Pts',(-32.0977199449364,-31.1807841743797,
2.3550019102838));
#20357=CARTESIAN_POINT('Ctrl Pts',(-30.2134432077683,-35.3138779741053,
2.19800178293155));
#20358=CARTESIAN_POINT('Ctrl Pts',(-32.621319267345,-39.1655160273689,2.04100165557929));
#20359=CARTESIAN_POINT('Ctrl Pts',(-37.1621783376115,-39.2818925846584,
1.88400152822705));
#20360=CARTESIAN_POINT('Ctrl Pts',(-38.9994904706692,-36.6528809760016,
1.77314212542643));
#20361=CARTESIAN_POINT('Ctrl Pts',(-39.0789669178819,-35.1605220209328,
1.7146160984099));
#20362=CARTESIAN_POINT('Ctrl Pts',(-39.0778200867196,-35.0024921203811,
1.70842344717745));
#20363=CARTESIAN_POINT('Ctrl Pts',(-39.0758434671966,-35.0032082366984,
2.79157655282255));
#20364=CARTESIAN_POINT('Ctrl Pts',(-39.0663197739578,-33.8995579722718,
2.74838292522283));
#20365=CARTESIAN_POINT('Ctrl Pts',(-38.037544158487,-31.4430705734335,2.65285592183902));
#20366=CARTESIAN_POINT('Ctrl Pts',(-33.9071517375455,-30.3293121048675,
2.50499554267113));
#20367=CARTESIAN_POINT('Ctrl Pts',(-30.5014133532831,-33.3349589868354,
2.34799541531887));
#20368=CARTESIAN_POINT('Ctrl Pts',(-31.12960079995,-37.8336643815683,2.19099528796663));
#20369=CARTESIAN_POINT('Ctrl Pts',(-35.2284122851668,-39.7913952114128,
2.03399516061437));
#20370=CARTESIAN_POINT('Ctrl Pts',(-38.5306036675732,-37.8080765974554,
1.90085558223301));
#20371=CARTESIAN_POINT('Ctrl Pts',(-39.0659286289889,-35.7304351180991,
1.82004937963574));
#20372=CARTESIAN_POINT('Ctrl Pts',(-39.0674338139571,-34.9990828447087,
1.79157655282254));
#20373=CARTESIAN_POINT('Origin',(-35.,-35.,10.2084234471775));
#20374=CARTESIAN_POINT('',(-39.0750717811968,-34.9966356393236,3.79157655282255));
#20375=CARTESIAN_POINT('',(-39.0687110107696,-35.0023266135852,3.70842344717746));
#20376=CARTESIAN_POINT('',(-39.0735,-34.9999999999999,10.2084234471775));
#20377=CARTESIAN_POINT('Ctrl Pts',(-39.0687110107696,-35.0023266135852,
3.70842344717746));
#20378=CARTESIAN_POINT('Ctrl Pts',(-39.0642694397141,-34.16887057793,3.67594994115225));
#20379=CARTESIAN_POINT('Ctrl Pts',(-38.4124447778773,-31.9858617174929,
3.59114305934296));
#20380=CARTESIAN_POINT('Ctrl Pts',(-34.8667814687478,-30.2050135847982,
3.45400280174957));
#20381=CARTESIAN_POINT('Ctrl Pts',(-30.9271137663599,-32.4659835103585,
3.29700267439732));
#20382=CARTESIAN_POINT('Ctrl Pts',(-30.6396422127733,-36.9992303202149,
3.14000254704507));
#20383=CARTESIAN_POINT('Ctrl Pts',(-34.2621453393335,-39.7397481467912,
2.98300241969281));
#20384=CARTESIAN_POINT('Ctrl Pts',(-38.1877200741971,-38.356442172659,2.83914271973695));
#20385=CARTESIAN_POINT('Ctrl Pts',(-39.0641484919776,-35.9998016365399,
2.74761639556516));
#20386=CARTESIAN_POINT('Ctrl Pts',(-39.0728771860086,-34.996494180098,2.70842344717745));
#20387=CARTESIAN_POINT('Ctrl Pts',(-39.0750717811968,-34.9966356393236,
3.79157655282255));
#20388=CARTESIAN_POINT('Ctrl Pts',(-39.0773739047593,-34.7360557814575,
3.78138322237809));
#20389=CARTESIAN_POINT('Ctrl Pts',(-38.9368588004177,-33.1401094404144,
3.71885651614954));
#20390=CARTESIAN_POINT('Ctrl Pts',(-36.8334388106793,-30.5673771631648,
3.6039964341369));
#20391=CARTESIAN_POINT('Ctrl Pts',(-32.3142506564274,-31.0255322944533,
3.44699630678465));
#20392=CARTESIAN_POINT('Ctrl Pts',(-30.2033997043049,-35.0476307446275,
3.28999617943239));
#20393=CARTESIAN_POINT('Ctrl Pts',(-32.3937062542216,-39.0270182530956,
3.13299605208014));
#20394=CARTESIAN_POINT('Ctrl Pts',(-36.9211014088136,-39.3953398526252,
2.97599592472789));
#20395=CARTESIAN_POINT('Ctrl Pts',(-38.9541949543872,-36.8053221809578,
2.86218942497536));
#20396=CARTESIAN_POINT('Ctrl Pts',(-39.077858675523,-35.2367400343503,2.80071630100691));
#20397=CARTESIAN_POINT('Ctrl Pts',(-39.0758434671966,-35.0032082366984,
2.79157655282255));
#20398=CARTESIAN_POINT('Origin',(-35.,-35.,10.2084234471775));
#20399=CARTESIAN_POINT('',(-39.0676603684793,-35.0013188448613,4.79157655282255));
#20400=CARTESIAN_POINT('',(-39.0799229210932,-35.0002389671693,4.70842344717745));
#20401=CARTESIAN_POINT('',(-39.0735,-34.9999999999999,10.2084234471775));
#20402=CARTESIAN_POINT('Ctrl Pts',(-39.0799229210932,-35.0002389671693,
4.70842344717745));
#20403=CARTESIAN_POINT('Ctrl Pts',(-39.0787772264229,-33.680000347528,4.65661686252342));
#20404=CARTESIAN_POINT('Ctrl Pts',(-37.6705857942339,-31.023995125205,4.5524769020853));
#20405=CARTESIAN_POINT('Ctrl Pts',(-33.1665612371704,-30.5673772788489,
4.39600356586309));
#20406=CARTESIAN_POINT('Ctrl Pts',(-30.291435328683,-34.0839974792893,4.23900343851084));
#20407=CARTESIAN_POINT('Ctrl Pts',(-31.6385245327839,-38.4220059271175,
4.08200331115859));
#20408=CARTESIAN_POINT('Ctrl Pts',(-35.9998810371616,-39.6914688314679,
3.92500318380634));
#20409=CARTESIAN_POINT('Ctrl Pts',(-38.7479938252585,-37.361615545083,3.80047656247929));
#20410=CARTESIAN_POINT('Ctrl Pts',(-39.0714273489013,-35.5120445450279,
3.72828331693633));
#20411=CARTESIAN_POINT('Ctrl Pts',(-39.0687110107696,-35.0023266135852,
3.70842344717746));
#20412=CARTESIAN_POINT('Ctrl Pts',(-39.0676603684793,-35.0013188448613,
4.79157655282255));
#20413=CARTESIAN_POINT('Ctrl Pts',(-39.065407667772,-34.2430102880461,4.76205014374926));
#20414=CARTESIAN_POINT('Ctrl Pts',(-38.5005818838826,-32.1375386968076,
4.68019035889189));
#20415=CARTESIAN_POINT('Ctrl Pts',(-35.1332185347277,-30.2050134596587,
4.54599719825043));
#20416=CARTESIAN_POINT('Ctrl Pts',(-31.0740923862265,-32.2437539129077,
4.38899707089817));
#20417=CARTESIAN_POINT('Ctrl Pts',(-30.535365261007,-36.7540466716456,4.23199694354592));
#20418=CARTESIAN_POINT('Ctrl Pts',(-34.0001189367432,-39.6914689539076,
4.07499681619366));
#20419=CARTESIAN_POINT('Ctrl Pts',(-38.0783117770221,-38.5044266833838,
3.92819001928587));
#20420=CARTESIAN_POINT('Ctrl Pts',(-39.0655546178097,-36.0738936645484,
3.83371659816217));
#20421=CARTESIAN_POINT('Ctrl Pts',(-39.0750717811968,-34.9966356393236,
3.79157655282255));
#20422=CARTESIAN_POINT('Origin',(-35.,-35.,10.2084234471775));
#20423=CARTESIAN_POINT('',(-39.0792024631389,-35.0015161209354,5.79157655282255));
#20424=CARTESIAN_POINT('',(-39.0692231423099,-34.9973709029543,5.70842344717745));
#20425=CARTESIAN_POINT('',(-39.0735,-34.9999999999999,10.2084234471775));
#20426=CARTESIAN_POINT('Ctrl Pts',(-39.0692231423099,-34.9973709029543,
5.70842344717745));
#20427=CARTESIAN_POINT('Ctrl Pts',(-39.072153886322,-34.5148469224124,5.68961715967868));
#20428=CARTESIAN_POINT('Ctrl Pts',(-38.7712973835496,-32.6931086863282,
5.61847749639582));
#20429=CARTESIAN_POINT('Ctrl Pts',(-36.0928482339355,-30.3293122267992,
5.49500445732888));
#20430=CARTESIAN_POINT('Ctrl Pts',(-31.7071424564414,-31.5119158276916,
5.33800432997661));
#20431=CARTESIAN_POINT('Ctrl Pts',(-30.2741736217725,-35.8223180338192,
5.18100420262437));
#20432=CARTESIAN_POINT('Ctrl Pts',(-33.0788986413239,-39.395339737909,5.02400407527211));
#20433=CARTESIAN_POINT('Ctrl Pts',(-37.6062936777584,-39.0270181479993,
4.86700394791986));
#20434=CARTESIAN_POINT('Ctrl Pts',(-39.0738472616523,-36.3607409549812,
4.76181040522164));
#20435=CARTESIAN_POINT('Ctrl Pts',(-39.0799345709982,-35.013663708426,4.7089502383075));
#20436=CARTESIAN_POINT('Ctrl Pts',(-39.0799229210932,-35.0002389671693,
4.70842344717745));
#20437=CARTESIAN_POINT('Ctrl Pts',(-39.0792024631389,-35.0015161209354,
5.79157655282255));
#20438=CARTESIAN_POINT('Ctrl Pts',(-39.0731679256319,-33.7557919674485,
5.74271706512043));
#20439=CARTESIAN_POINT('Ctrl Pts',(-37.8030027181165,-31.1651102767228,
5.64152420163424));
#20440=CARTESIAN_POINT('Ctrl Pts',(-33.4155016033557,-30.4724169111822,
5.48799796236394));
#20441=CARTESIAN_POINT('Ctrl Pts',(-30.3495576440316,-33.8239773440302,
5.3309978350117));
#20442=CARTESIAN_POINT('Ctrl Pts',(-31.4537101308888,-38.230088373826,5.17399770765944));
#20443=CARTESIAN_POINT('Ctrl Pts',(-35.7378546799324,-39.7397482704758,
5.01699758030718));
#20444=CARTESIAN_POINT('Ctrl Pts',(-38.6790876767283,-37.5146290150371,
4.88952386202822));
#20445=CARTESIAN_POINT('Ctrl Pts',(-39.0694004131258,-35.5870561070142,
4.81438351953334));
#20446=CARTESIAN_POINT('Ctrl Pts',(-39.0676603684793,-35.0013188448613,
4.79157655282255));
#20447=CARTESIAN_POINT('Origin',(-35.,-35.,10.2084234471775));
#20448=CARTESIAN_POINT('',(-39.0709664927331,-34.9967444357251,6.79157655282255));
#20449=CARTESIAN_POINT('',(-39.0721140267755,-35.0034548068065,6.70842344717746));
#20450=CARTESIAN_POINT('',(-39.0735,-34.9999999999999,10.2084234471775));
#20451=CARTESIAN_POINT('Ctrl Pts',(-39.0721140267755,-35.0034548068065,
6.70842344717746));
#20452=CARTESIAN_POINT('Ctrl Pts',(-39.0638862819908,-34.0266505561004,
6.67028408104986));
#20453=CARTESIAN_POINT('Ctrl Pts',(-38.2252022081515,-31.6968182141492,
6.57981133913816));
#20454=CARTESIAN_POINT('Ctrl Pts',(-34.3564136921927,-30.2465364275518,
6.4370052214424));
#20455=CARTESIAN_POINT('Ctrl Pts',(-30.6802034020135,-32.9145736277213,
6.28000509409013));
#20456=CARTESIAN_POINT('Ctrl Pts',(-30.8775957137286,-37.4526369907548,
6.12300496673789));
#20457=CARTESIAN_POINT('Ctrl Pts',(-34.7715877207675,-39.7913950861294,
5.96600483938563));
#20458=CARTESIAN_POINT('Ctrl Pts',(-38.3794222668459,-38.0681714287485,
5.82781099953215));
#20459=CARTESIAN_POINT('Ctrl Pts',(-39.0639983304887,-35.8575951283075,
5.74195053546276));
#20460=CARTESIAN_POINT('Ctrl Pts',(-39.0692231423099,-34.9973709029543,
5.70842344717745));
#20461=CARTESIAN_POINT('Ctrl Pts',(-39.0709664927331,-34.9967444357251,
6.79157655282255));
#20462=CARTESIAN_POINT('Ctrl Pts',(-39.074129342561,-34.5902726781194,6.77571736227569));
#20463=CARTESIAN_POINT('Ctrl Pts',(-38.8328831908397,-32.8461583454701,
6.70752479594475));
#20464=CARTESIAN_POINT('Ctrl Pts',(-36.3504797430715,-30.3972101963624,
6.58699885382972));
#20465=CARTESIAN_POINT('Ctrl Pts',(-31.905896825022,-31.3344599279876,6.42999872647746));
#20466=CARTESIAN_POINT('Ctrl Pts',(-30.2358028418083,-35.5586616666892,
6.27299859912522));
#20467=CARTESIAN_POINT('Ctrl Pts',(-32.83782160528,-39.2818926978495,6.11599847177295));
#20468=CARTESIAN_POINT('Ctrl Pts',(-37.3786807951101,-39.1655161353224,
5.95899834442071));
#20469=CARTESIAN_POINT('Ctrl Pts',(-39.0372097938135,-36.5125334877904,
5.85085770477057));
#20470=CARTESIAN_POINT('Ctrl Pts',(-39.0796315161011,-35.090086560245,5.79505044090452));
#20471=CARTESIAN_POINT('Ctrl Pts',(-39.0792024631389,-35.0015161209354,
5.79157655282255));
#20472=CARTESIAN_POINT('Origin',(-35.,-35.,10.2084234471775));
#20473=CARTESIAN_POINT('',(-39.0691247390887,-35.0040754761348,7.79157655282255));
#20474=CARTESIAN_POINT('',(-39.0784093524563,-34.997955826836,7.70842344717746));
#20475=CARTESIAN_POINT('',(-39.0735,-34.9999999999999,10.2084234471775));
#20476=CARTESIAN_POINT('',(-36.0520713770612,-38.9352951690526,8.));
#20477=CARTESIAN_POINT('Ctrl Pts',(-36.0520713770612,-38.9352951690526,
8.));
#20478=CARTESIAN_POINT('Ctrl Pts',(-37.3460763064865,-38.5893527455387,
7.94766662421592));
#20479=CARTESIAN_POINT('Ctrl Pts',(-38.8056934287649,-37.2206664159851,
7.87819214182344));
#20480=CARTESIAN_POINT('Ctrl Pts',(-39.0721265495934,-35.4436566771087,
7.80871765943095));
#20481=CARTESIAN_POINT('Ctrl Pts',(-39.0691247390887,-35.0040754761348,
7.79157655282255));
#20482=CARTESIAN_POINT('',(-33.9452801041878,-38.9416007879337,8.));
#20483=CARTESIAN_POINT('Origin',(-35.,-35.,8.));
#20484=CARTESIAN_POINT('Ctrl Pts',(-33.9452677648582,-38.941630165528,8.));
#20485=CARTESIAN_POINT('Ctrl Pts',(-35.1775571519718,-39.2670003808689,
7.95000212253756));
#20486=CARTESIAN_POINT('Ctrl Pts',(-37.9028288422611,-38.6929823061133,
7.85280993826337));
#20487=CARTESIAN_POINT('Ctrl Pts',(-39.0706575059758,-36.2016126262027,
7.75561775398919));
#20488=CARTESIAN_POINT('Ctrl Pts',(-39.0784093524563,-34.997955826836,7.70842344717745));
#20489=CARTESIAN_POINT('Origin',(35.,-35.,10.2084234471775));
#20490=CARTESIAN_POINT('',(30.9212701195312,-34.9980516557686,0.791576552822542));
#20491=CARTESIAN_POINT('',(30.9328376585755,-35.000159236028,0.708423447177449));
#20492=CARTESIAN_POINT('',(30.9265,-34.9999999999999,10.2084234471775));
#20493=CARTESIAN_POINT('',(36.0520713770612,-38.9352951690526,0.));
#20494=CARTESIAN_POINT('Ctrl Pts',(30.9328376585755,-35.000159236028,0.708423447177449));
#20495=CARTESIAN_POINT('Ctrl Pts',(30.9332830863018,-34.31144230346,0.681615801254637));
#20496=CARTESIAN_POINT('Ctrl Pts',(31.423729341332,-32.2777627653814,0.602474779547741));
#20497=CARTESIAN_POINT('Ctrl Pts',(34.6204730639081,-30.2191415991965,0.471000382056761));
#20498=CARTESIAN_POINT('Ctrl Pts',(38.7813009234074,-32.0442168078902,0.314000254704507));
#20499=CARTESIAN_POINT('Ctrl Pts',(39.5450614875854,-36.5273565705141,0.157000127352254));
#20500=CARTESIAN_POINT('Ctrl Pts',(37.3460763064866,-38.5893527455387,0.0523333757840845));
#20501=CARTESIAN_POINT('Ctrl Pts',(36.0520713770612,-38.9352951690526,0.));
#20502=CARTESIAN_POINT('',(33.9452809380949,-38.9416008127442,2.82508323912273E-15));
#20503=CARTESIAN_POINT('Origin',(35.,-35.,0.));
#20504=CARTESIAN_POINT('Ctrl Pts',(30.9212701195312,-34.9980516557686,0.791576552822542));
#20505=CARTESIAN_POINT('Ctrl Pts',(30.9205868455494,-34.8825847167923,0.787049082480475));
#20506=CARTESIAN_POINT('Ctrl Pts',(30.9769555821544,-33.4331078068366,0.730188236354323));
#20507=CARTESIAN_POINT('Ctrl Pts',(32.704491289799,-30.7882324000235,0.620994014444087));
#20508=CARTESIAN_POINT('Ctrl Pts',(37.2468174060219,-30.7615623188695,0.463993887091833));
#20509=CARTESIAN_POINT('Ctrl Pts',(39.7742801854456,-34.536716632844,0.306993759739581));
#20510=CARTESIAN_POINT('Ctrl Pts',(38.0469263053514,-38.6626279973746,0.152329130708969));
#20511=CARTESIAN_POINT('Ctrl Pts',(35.1775586628442,-39.2670009745688,0.0499978774624438));
#20512=CARTESIAN_POINT('Ctrl Pts',(33.94526862329,-38.9416301412996,2.47469145869816E-15));
#20513=CARTESIAN_POINT('Origin',(35.,-35.,10.2084234471775));
#20514=CARTESIAN_POINT('',(30.9325671258701,-34.9990828432724,1.79157655282254));
#20515=CARTESIAN_POINT('',(30.9221796304986,-35.0024921194124,1.70842344717745));
#20516=CARTESIAN_POINT('',(30.9265,-34.9999999999999,10.2084234471775));
#20517=CARTESIAN_POINT('Ctrl Pts',(30.9221796304986,-35.0024921194124,1.70842344717745));
#20518=CARTESIAN_POINT('Ctrl Pts',(30.9307245358113,-33.8250296189916,1.66228272262581));
#20519=CARTESIAN_POINT('Ctrl Pts',(32.0812070745664,-31.2974912653129,1.56380862229009));
#20520=CARTESIAN_POINT('Ctrl Pts',(36.3504798077544,-30.397209980765,1.41300114617028));
#20521=CARTESIAN_POINT('Ctrl Pts',(39.5841211762074,-33.5872716944053,1.25600101881803));
#20522=CARTESIAN_POINT('Ctrl Pts',(38.7070435276578,-38.0442501505519,1.09900089146578));
#20523=CARTESIAN_POINT('Ctrl Pts',(34.5060129254091,-39.7711992366401,0.942000764113522));
#20524=CARTESIAN_POINT('Ctrl Pts',(31.3893173078737,-37.6557923296961,0.811808282684079));
#20525=CARTESIAN_POINT('Ctrl Pts',(30.9324135307783,-35.6559423817109,0.733949177038721));
#20526=CARTESIAN_POINT('Ctrl Pts',(30.9328376585755,-35.000159236028,0.708423447177449));
#20527=CARTESIAN_POINT('Ctrl Pts',(30.9325671258701,-34.9990828432724,1.79157655282254));
#20528=CARTESIAN_POINT('Ctrl Pts',(30.931305764143,-34.3862015569849,1.76771600385165));
#20529=CARTESIAN_POINT('Ctrl Pts',(31.3469048767902,-32.4307110971121,1.69152207909667));
#20530=CARTESIAN_POINT('Ctrl Pts',(34.3564138261785,-30.2465374145616,1.56299477855761));
#20531=CARTESIAN_POINT('Ctrl Pts',(38.6097341605507,-31.8409675209513,1.40599465120535));
#20532=CARTESIAN_POINT('Ctrl Pts',(39.6261694334752,-36.2681500029269,1.2489945238531));
#20533=CARTESIAN_POINT('Ctrl Pts',(36.4942778376799,-39.5581346787212,1.09199439650085));
#20534=CARTESIAN_POINT('Ctrl Pts',(32.1514014998571,-38.7838588891191,0.939521739490662));
#20535=CARTESIAN_POINT('Ctrl Pts',(30.928484861737,-36.2172758912295,0.839382458264559));
#20536=CARTESIAN_POINT('Ctrl Pts',(30.9212701195312,-34.9980516557686,0.791576552822542));
#20537=CARTESIAN_POINT('Origin',(35.,-35.,10.2084234471775));
#20538=CARTESIAN_POINT('',(30.9241574748343,-35.0032082359637,2.79157655282255));
#20539=CARTESIAN_POINT('',(30.9271225309901,-34.9964941798068,2.70842344717745));
#20540=CARTESIAN_POINT('',(30.9265,-34.9999999999999,10.2084234471775));
#20541=CARTESIAN_POINT('Ctrl Pts',(30.9271225309901,-34.9964941798068,2.70842344717745));
#20542=CARTESIAN_POINT('Ctrl Pts',(30.9241960153079,-34.6601099513618,2.69528301978107));
#20543=CARTESIAN_POINT('Ctrl Pts',(31.1149287231428,-32.9873057374911,2.62980921660061));
#20544=CARTESIAN_POINT('Ctrl Pts',(33.4155015345008,-30.4724167149005,2.51200203763606));
#20545=CARTESIAN_POINT('Ctrl Pts',(37.9022802570419,-31.180783908422,2.3550019102838));
#20546=CARTESIAN_POINT('Ctrl Pts',(39.7865571243079,-35.3138779969793,2.19800178293155));
#20547=CARTESIAN_POINT('Ctrl Pts',(37.3786808989502,-39.1655163148135,2.04100165557929));
#20548=CARTESIAN_POINT('Ctrl Pts',(32.8378215103303,-39.2818928860424,1.88400152822704));
#20549=CARTESIAN_POINT('Ctrl Pts',(31.0005092531499,-36.6528810868796,1.77314212542643));
#20550=CARTESIAN_POINT('Ctrl Pts',(30.9210327993872,-35.1605220306295,1.7146160984099));
#20551=CARTESIAN_POINT('Ctrl Pts',(30.9221796304986,-35.0024921194124,1.70842344717745));
#20552=CARTESIAN_POINT('Ctrl Pts',(30.9241574748343,-35.0032082359637,2.79157655282255));
#20553=CARTESIAN_POINT('Ctrl Pts',(30.9336811658698,-33.8995582265895,2.74838292522282));
#20554=CARTESIAN_POINT('Ctrl Pts',(31.9624565435572,-31.4430713953983,2.65285592183902));
#20555=CARTESIAN_POINT('Ctrl Pts',(36.092848009894,-30.329313184686,2.50499554267113));
#20556=CARTESIAN_POINT('Ctrl Pts',(39.4985856069267,-33.3349593710879,2.34799541531888));
#20557=CARTESIAN_POINT('Ctrl Pts',(38.8703983056154,-37.8336637277424,2.19099528796662));
#20558=CARTESIAN_POINT('Ctrl Pts',(34.7715877673847,-39.7913941019012,2.03399516061437));
#20559=CARTESIAN_POINT('Ctrl Pts',(31.4693971488356,-37.8080759514836,1.90085558223301));
#20560=CARTESIAN_POINT('Ctrl Pts',(30.9340723106019,-35.73043494849,1.82004937963573));
#20561=CARTESIAN_POINT('Ctrl Pts',(30.9325671258701,-34.9990828432724,1.79157655282254));
#20562=CARTESIAN_POINT('Origin',(35.,-35.,10.2084234471775));
#20563=CARTESIAN_POINT('',(30.9249291606556,-34.9966356401017,3.79157655282255));
#20564=CARTESIAN_POINT('',(30.9312887064921,-35.0023266137465,3.70842344717745));
#20565=CARTESIAN_POINT('',(30.9265,-34.9999999999999,10.2084234471775));
#20566=CARTESIAN_POINT('Ctrl Pts',(30.9312887064921,-35.0023266137465,3.70842344717745));
#20567=CARTESIAN_POINT('Ctrl Pts',(30.9357302778565,-34.1688705201733,3.67594994115225));
#20568=CARTESIAN_POINT('Ctrl Pts',(31.5875549849899,-31.9858615080358,3.59114305934295));
#20569=CARTESIAN_POINT('Ctrl Pts',(35.1332185405061,-30.2050132515957,3.45400280174957));
#20570=CARTESIAN_POINT('Ctrl Pts',(39.0728865166754,-32.4659833342563,3.29700267439732));
#20571=CARTESIAN_POINT('Ctrl Pts',(39.3603580902194,-36.9992304591644,3.14000254704507));
#20572=CARTESIAN_POINT('Ctrl Pts',(35.7378547119649,-39.73974847612,2.98300241969282));
#20573=CARTESIAN_POINT('Ctrl Pts',(31.8122797042457,-38.3564424059702,2.83914271973694));
#20574=CARTESIAN_POINT('Ctrl Pts',(30.9358512256228,-35.9998017059771,2.74761639556516));
#20575=CARTESIAN_POINT('Ctrl Pts',(30.9271225309901,-34.9964941798068,2.70842344717745));
#20576=CARTESIAN_POINT('Ctrl Pts',(30.9249291606557,-34.9966356401017,3.79157655282255));
#20577=CARTESIAN_POINT('Ctrl Pts',(30.9226270376253,-34.7360558424623,3.78138322237808));
#20578=CARTESIAN_POINT('Ctrl Pts',(31.0631421094905,-33.1401098702831,3.71885651614953));
#20579=CARTESIAN_POINT('Ctrl Pts',(33.1665616130745,-30.567378187653,3.6039964341369));
#20580=CARTESIAN_POINT('Ctrl Pts',(37.6857487228281,-31.0255332130596,3.44699630678465));
#20581=CARTESIAN_POINT('Ctrl Pts',(39.7965991870786,-35.0476307336073,3.28999617943239));
#20582=CARTESIAN_POINT('Ctrl Pts',(37.606293143399,-39.0270173223719,3.13299605208014));
#20583=CARTESIAN_POINT('Ctrl Pts',(33.0788990351993,-39.3953388367078,2.97599592472789));
#20584=CARTESIAN_POINT('Ctrl Pts',(31.0458059595307,-36.8053217637502,2.86218942497536));
#20585=CARTESIAN_POINT('Ctrl Pts',(30.9221422669741,-35.2367399796465,2.80071630100691));
#20586=CARTESIAN_POINT('Ctrl Pts',(30.9241574748343,-35.0032082359637,2.79157655282255));
#20587=CARTESIAN_POINT('Origin',(35.,-35.,10.2084234471775));
#20588=CARTESIAN_POINT('',(30.9323405716502,-35.0013188445396,4.79157655282255));
#20589=CARTESIAN_POINT('',(30.9200767953891,-35.0002389671868,4.70842344717745));
#20590=CARTESIAN_POINT('',(30.9265,-34.9999999999999,10.2084234471775));
#20591=CARTESIAN_POINT('Ctrl Pts',(30.9200767953891,-35.0002389671868,4.70842344717745));
#20592=CARTESIAN_POINT('Ctrl Pts',(30.9212224901389,-33.6800002558017,4.65661686252342));
#20593=CARTESIAN_POINT('Ctrl Pts',(32.3294140201846,-31.0239948489069,4.5524769020853));
#20594=CARTESIAN_POINT('Ctrl Pts',(36.8334388902368,-30.5673769708228,4.39600356586309));
#20595=CARTESIAN_POINT('Ctrl Pts',(39.7085649985197,-34.0839974156347,4.23900343851085));
#20596=CARTESIAN_POINT('Ctrl Pts',(38.3614757008081,-38.4220061649164,4.08200331115859));
#20597=CARTESIAN_POINT('Ctrl Pts',(34.0001188933562,-39.6914691574817,3.92500318380634));
#20598=CARTESIAN_POINT('Ctrl Pts',(31.2520059142893,-37.3616157091949,3.80047656247929));
#20599=CARTESIAN_POINT('Ctrl Pts',(30.9285723681714,-35.5120445806103,3.72828331693633));
#20600=CARTESIAN_POINT('Ctrl Pts',(30.9312887064921,-35.0023266137465,3.70842344717745));
#20601=CARTESIAN_POINT('Ctrl Pts',(30.9323405716502,-35.0013188445396,4.79157655282255));
#20602=CARTESIAN_POINT('Ctrl Pts',(30.9345932718416,-34.2430104629966,4.76205014374926));
#20603=CARTESIAN_POINT('Ctrl Pts',(31.4994189252081,-32.1375393584237,4.68019035889188));
#20604=CARTESIAN_POINT('Ctrl Pts',(34.8667814960507,-30.2050145678827,4.54599719825042));
#20605=CARTESIAN_POINT('Ctrl Pts',(38.9259067064028,-32.2437545499559,4.38899707089817));
#20606=CARTESIAN_POINT('Ctrl Pts',(39.4646337070995,-36.7540462662356,4.23199694354592));
#20607=CARTESIAN_POINT('Ctrl Pts',(35.9998808321606,-39.6914678695931,4.07499681619366));
#20608=CARTESIAN_POINT('Ctrl Pts',(31.921688934453,-38.5044258734202,3.92819001928587));
#20609=CARTESIAN_POINT('Ctrl Pts',(30.934446321843,-36.0738934163447,3.83371659816217));
#20610=CARTESIAN_POINT('Ctrl Pts',(30.9249291606557,-34.9966356401017,3.79157655282255));
#20611=CARTESIAN_POINT('Origin',(35.,-35.,10.2084234471775));
#20612=CARTESIAN_POINT('',(30.9207984791111,-35.0015161195221,5.79157655282255));
#20613=CARTESIAN_POINT('',(30.93077657492,-34.9973709027416,5.70842344717745));
#20614=CARTESIAN_POINT('',(30.9265,-34.9999999999999,10.2084234471775));
#20615=CARTESIAN_POINT('Ctrl Pts',(30.93077657492,-34.9973709027416,5.70842344717745));
#20616=CARTESIAN_POINT('Ctrl Pts',(30.9278458307013,-34.5148468886989,5.68961715967867));
#20617=CARTESIAN_POINT('Ctrl Pts',(31.2287023543687,-32.6931085261371,5.61847749639581));
#20618=CARTESIAN_POINT('Ctrl Pts',(33.9071516901285,-30.3293119021379,5.49500445732887));
#20619=CARTESIAN_POINT('Ctrl Pts',(38.292857772379,-31.5119155853487,5.33800432997662));
#20620=CARTESIAN_POINT('Ctrl Pts',(39.7258267066312,-35.8223180909381,5.18100420262436));
#20621=CARTESIAN_POINT('Ctrl Pts',(36.9211014921746,-39.3953400433581,5.02400407527211));
#20622=CARTESIAN_POINT('Ctrl Pts',(32.3937061411281,-39.0270184278339,4.86700394791986));
#20623=CARTESIAN_POINT('Ctrl Pts',(30.9261524552523,-36.3607410495406,4.76181040522164));
#20624=CARTESIAN_POINT('Ctrl Pts',(30.9200651454832,-35.0136637093765,4.7089502383075));
#20625=CARTESIAN_POINT('Ctrl Pts',(30.9200767953891,-35.0002389671868,4.70842344717745));
#20626=CARTESIAN_POINT('Ctrl Pts',(30.9207984791111,-35.0015161195221,5.79157655282254));
#20627=CARTESIAN_POINT('Ctrl Pts',(30.9268330150145,-33.7557922534996,5.74271706512043));
#20628=CARTESIAN_POINT('Ctrl Pts',(32.1969979306855,-31.1651111648659,5.64152420163423));
#20629=CARTESIAN_POINT('Ctrl Pts',(36.584498029893,-30.4724179566463,5.48799796236395));
#20630=CARTESIAN_POINT('Ctrl Pts',(39.6504412814188,-33.8239776163473,5.33099783501169));
#20631=CARTESIAN_POINT('Ctrl Pts',(38.5462890493217,-38.2300876270061,5.17399770765944));
#20632=CARTESIAN_POINT('Ctrl Pts',(34.2621454906851,-39.7397471751372,5.01699758030718));
#20633=CARTESIAN_POINT('Ctrl Pts',(31.3209131735827,-37.5146284338107,4.88952386202822));
#20634=CARTESIAN_POINT('Ctrl Pts',(30.9306005274021,-35.5870559713077,4.81438351953334));
#20635=CARTESIAN_POINT('Ctrl Pts',(30.9323405716502,-35.0013188445396,4.79157655282255));
#20636=CARTESIAN_POINT('Origin',(35.,-35.,10.2084234471775));
#20637=CARTESIAN_POINT('',(30.9290344477858,-34.9967444478932,6.79157655282255));
#20638=CARTESIAN_POINT('',(30.9278856911952,-35.003454802609,6.70842344717745));
#20639=CARTESIAN_POINT('',(30.9265,-34.9999999999999,10.2084234471775));
#20640=CARTESIAN_POINT('Ctrl Pts',(30.9278856911952,-35.003454802609,6.70842344717745));
#20641=CARTESIAN_POINT('Ctrl Pts',(30.9361134364198,-34.0266504850423,6.67028408104985));
#20642=CARTESIAN_POINT('Ctrl Pts',(31.7747975664789,-31.6968179913154,6.57981133913816));
#20643=CARTESIAN_POINT('Ctrl Pts',(35.6435863532121,-30.2465360930486,6.43700522144239));
#20644=CARTESIAN_POINT('Ctrl Pts',(39.3197968978512,-32.9145734850341,6.28000509409014));
#20645=CARTESIAN_POINT('Ctrl Pts',(39.1224045728929,-37.4526371600059,6.12300496673789));
#20646=CARTESIAN_POINT('Ctrl Pts',(35.2284122950338,-39.7913954197145,5.96600483938562));
#20647=CARTESIAN_POINT('Ctrl Pts',(31.6205774983358,-38.0681716417432,5.82781099953216));
#20648=CARTESIAN_POINT('Ctrl Pts',(30.9360013871094,-35.857595187819,5.74195053546276));
#20649=CARTESIAN_POINT('Ctrl Pts',(30.93077657492,-34.9973709027416,5.70842344717745));
#20650=CARTESIAN_POINT('Ctrl Pts',(30.9290344477858,-34.9967444478932,6.79157655282255));
#20651=CARTESIAN_POINT('Ctrl Pts',(30.9258715916941,-34.5902727617055,6.77571736227569));
#20652=CARTESIAN_POINT('Ctrl Pts',(31.1671176609215,-32.8461587416485,6.70752479594475));
#20653=CARTESIAN_POINT('Ctrl Pts',(33.6495206016122,-30.3972113452741,6.58699885382972));
#20654=CARTESIAN_POINT('Ctrl Pts',(38.09410244091,-31.3344607296745,6.42999872647747));
#20655=CARTESIAN_POINT('Ctrl Pts',(39.7641960678496,-35.558661561786,6.27299859912521));
#20656=CARTESIAN_POINT('Ctrl Pts',(37.1621778889461,-39.2818916953666,6.11599847177296));
#20657=CARTESIAN_POINT('Ctrl Pts',(32.6213197580022,-39.1655151793351,5.95899834442071));
#20658=CARTESIAN_POINT('Ctrl Pts',(30.962791139069,-36.5125331378606,5.85085770477057));
#20659=CARTESIAN_POINT('Ctrl Pts',(30.920369426263,-35.0900865383931,5.79505044090451));
#20660=CARTESIAN_POINT('Ctrl Pts',(30.9207984791111,-35.0015161195221,5.79157655282254));
#20661=CARTESIAN_POINT('Origin',(35.,-35.,10.2084234471775));
#20662=CARTESIAN_POINT('',(30.9308748007386,-35.0040807474719,7.79157655282254));
#20663=CARTESIAN_POINT('',(30.9215903995924,-34.9979557257256,7.70842344717745));
#20664=CARTESIAN_POINT('',(30.9265,-34.9999999999999,10.2084234471775));
#20665=CARTESIAN_POINT('',(33.9479286229388,-38.9352951690526,8.));
#20666=CARTESIAN_POINT('Ctrl Pts',(33.9479286229388,-38.9352951690526,8.));
#20667=CARTESIAN_POINT('Ctrl Pts',(32.6539236935135,-38.5893527455387,7.94766662421592));
#20668=CARTESIAN_POINT('Ctrl Pts',(31.1943052713303,-37.2206748258175,7.87819214182343));
#20669=CARTESIAN_POINT('Ctrl Pts',(30.9278727863252,-35.4436627970733,7.80871765943094));
#20670=CARTESIAN_POINT('Ctrl Pts',(30.9308748007386,-35.0040807474719,7.79157655282254));
#20671=CARTESIAN_POINT('',(36.0547201762178,-38.9416007819636,8.));
#20672=CARTESIAN_POINT('Origin',(35.,-35.,8.));
#20673=CARTESIAN_POINT('Ctrl Pts',(36.0547325237759,-38.9416301760088,8.));
#20674=CARTESIAN_POINT('Ctrl Pts',(34.822443357586,-39.2670001819919,7.95000212253756));
#20675=CARTESIAN_POINT('Ctrl Pts',(32.0971704836176,-38.6929832307492,7.85280993826338));
#20676=CARTESIAN_POINT('Ctrl Pts',(30.9293421550372,-36.2016127302822,7.75561775398919));
#20677=CARTESIAN_POINT('Ctrl Pts',(30.9215903995924,-34.9979557257256,7.70842344717745));
#20678=CARTESIAN_POINT('Origin',(35.,-35.,10.2084234471775));
#20679=CARTESIAN_POINT('Ctrl Pts',(30.9215903995924,-34.9979557257256,7.70842344717745));
#20680=CARTESIAN_POINT('Ctrl Pts',(30.9207462976534,-34.8668874511107,7.70328437820511));
#20681=CARTESIAN_POINT('Ctrl Pts',(30.9854756915705,-33.4019022214529,7.64581193344868));
#20682=CARTESIAN_POINT('Ctrl Pts',(32.753181490405,-30.7615622140283,7.53600611290817));
#20683=CARTESIAN_POINT('Ctrl Pts',(37.2955095733766,-30.7882306349807,7.3790059855559));
#20684=CARTESIAN_POINT('Ctrl Pts',(39.7793714317054,-34.5910508431566,7.22200585820367));
#20685=CARTESIAN_POINT('Ctrl Pts',(37.9775552386376,-38.7608686529102,7.0650057308514));
#20686=CARTESIAN_POINT('Ctrl Pts',(33.5057217267653,-39.5581360350982,6.90800560349915));
#20687=CARTESIAN_POINT('Ctrl Pts',(31.1346464724166,-37.067372389099,6.7891448422745));
#20688=CARTESIAN_POINT('Ctrl Pts',(30.9248236399074,-35.3669839150134,6.72261745683393));
#20689=CARTESIAN_POINT('Ctrl Pts',(30.9278856911952,-35.003454802609,6.70842344717745));
#20690=CARTESIAN_POINT('Ctrl Pts',(30.9308748007386,-35.0040807474719,7.79157655282254));
#20691=CARTESIAN_POINT('Ctrl Pts',(30.9370382125719,-34.10157834971,7.75638428364686));
#20692=CARTESIAN_POINT('Ctrl Pts',(31.6729756008745,-31.8449525580975,7.66885863868709));
#20693=CARTESIAN_POINT('Ctrl Pts',(35.3795267558193,-30.2191465582126,7.52899961794324));
#20694=CARTESIAN_POINT('Ctrl Pts',(39.1969165266342,-32.6774422642514,7.37199949059099));
#20695=CARTESIAN_POINT('Ctrl Pts',(39.2524336251343,-37.2202141105436,7.21499936323873));
#20696=CARTESIAN_POINT('Ctrl Pts',(35.4939867861423,-39.7711972931265,7.05799923588648));
#20697=CARTESIAN_POINT('Ctrl Pts',(31.7173198121032,-38.2186953257486,6.91685829908109));
#20698=CARTESIAN_POINT('Ctrl Pts',(30.9363086272988,-35.9315792701304,6.82805073805977));
#20699=CARTESIAN_POINT('Ctrl Pts',(30.9290344477858,-34.9967444478932,6.79157655282255));
#20700=CARTESIAN_POINT('Ctrl Pts',(37.6735319337713,-32.7141668369925,8.));
#20701=CARTESIAN_POINT('Ctrl Pts',(38.4251602751564,-33.5932784036374,7.94766662421592));
#20702=CARTESIAN_POINT('Ctrl Pts',(38.9814215765655,-36.1362159265307,7.84299987264775));
#20703=CARTESIAN_POINT('Ctrl Pts',(36.2450915261219,-38.9529260673994,7.6859997452955));
#20704=CARTESIAN_POINT('Ctrl Pts',(32.3914756047223,-38.2165112413961,7.52899961794324));
#20705=CARTESIAN_POINT('Ctrl Pts',(30.8773704214612,-34.5999494268526,7.37199949059098));
#20706=CARTESIAN_POINT('Ctrl Pts',(33.0598541530624,-31.3400748957517,7.21499936323873));
#20707=CARTESIAN_POINT('Ctrl Pts',(36.9821909719779,-31.3631032916521,7.05799923588648));
#20708=CARTESIAN_POINT('Ctrl Pts',(39.127025656321,-34.6468691152089,6.90099910853422));
#20709=CARTESIAN_POINT('Ctrl Pts',(37.5711428874206,-38.2475403183041,6.74399898118197));
#20710=CARTESIAN_POINT('Ctrl Pts',(33.7096786974094,-38.9359871126692,6.58699885382972));
#20711=CARTESIAN_POINT('Ctrl Pts',(31.005264414648,-36.0950579743517,6.42999872647747));
#20712=CARTESIAN_POINT('Ctrl Pts',(31.8829646703068,-32.272149334312,6.27299859912521));
#20713=CARTESIAN_POINT('Ctrl Pts',(35.5557419902844,-30.8953456995945,6.11599847177296));
#20714=CARTESIAN_POINT('Ctrl Pts',(38.7301793514647,-33.1992174379789,5.9589983444207));
#20715=CARTESIAN_POINT('Ctrl Pts',(38.5597294918745,-37.1178719063019,5.80199821706845));
#20716=CARTESIAN_POINT('Ctrl Pts',(35.1972358531438,-39.137408466637,5.6449980897162));
#20717=CARTESIAN_POINT('Ctrl Pts',(31.6578790286353,-37.4468920814909,5.48799796236395));
#20718=CARTESIAN_POINT('Ctrl Pts',(31.115434094392,-33.5622236362915,5.33099783501169));
#20719=CARTESIAN_POINT('Ctrl Pts',(34.0563166981778,-30.9668232762417,5.17399770765944));
#20720=CARTESIAN_POINT('Ctrl Pts',(37.8434091602659,-31.9880110645548,5.01699758030718));
#20721=CARTESIAN_POINT('Ctrl Pts',(39.0807893557322,-35.7100782827727,4.85999745295493));
#20722=CARTESIAN_POINT('Ctrl Pts',(36.6588865837055,-38.7954114649594,4.70299732560268));
#20723=CARTESIAN_POINT('Ctrl Pts',(32.7494442988629,-38.4773627887335,4.54599719825042));
#20724=CARTESIAN_POINT('Ctrl Pts',(30.8580969013801,-35.0411295327127,4.38899707089817));
#20725=CARTESIAN_POINT('Ctrl Pts',(32.6808337483856,-31.5680150335338,4.23199694354591));
#20726=CARTESIAN_POINT('Ctrl Pts',(36.5831892221451,-31.1723943770392,4.07499681619367));
#20727=CARTESIAN_POINT('Ctrl Pts',(39.0658837319978,-34.2090244039511,3.91799668884141));
#20728=CARTESIAN_POINT('Ctrl Pts',(37.9026612931367,-37.9549298355453,3.76099656148916));
#20729=CARTESIAN_POINT('Ctrl Pts',(34.1365946255998,-39.0511213358148,3.6039964341369));
#20730=CARTESIAN_POINT('Ctrl Pts',(31.144751840957,-36.5146334688211,3.44699630678465));
#20731=CARTESIAN_POINT('Ctrl Pts',(31.6099470650134,-32.6199592409358,3.2899961794324));
#20732=CARTESIAN_POINT('Ctrl Pts',(35.1150352807734,-30.8594903921659,3.13299605208014));
#20733=CARTESIAN_POINT('Ctrl Pts',(38.5169702522169,-32.811856236221,2.97599592472789));
#20734=CARTESIAN_POINT('Ctrl Pts',(38.7652042671773,-36.72635157484,2.81899579737563));
#20735=CARTESIAN_POINT('Ctrl Pts',(35.6371434759633,-39.0928109156136,2.66199567002339));
#20736=CARTESIAN_POINT('Ctrl Pts',(31.9377500537671,-37.7892074010372,2.50499554267113));
#20737=CARTESIAN_POINT('Ctrl Pts',(30.9843054629328,-33.9844949374723,2.34799541531888));
#20738=CARTESIAN_POINT('Ctrl Pts',(33.6317728360394,-31.0903954325918,2.19099528796662));
#20739=CARTESIAN_POINT('Ctrl Pts',(37.5061423356192,-31.7020761993063,2.03399516061437));
#20740=CARTESIAN_POINT('Ctrl Pts',(39.1332305596546,-35.2710361738983,1.87699503326212));
#20741=CARTESIAN_POINT('Ctrl Pts',(37.054010080289,-38.5969568276314,1.71999490590986));
#20742=CARTESIAN_POINT('Ctrl Pts',(33.1329414907541,-38.6974489325283,1.56299477855761));
#20743=CARTESIAN_POINT('Ctrl Pts',(30.8860772740811,-35.4824088577318,1.40599465120536));
#20744=CARTESIAN_POINT('Ctrl Pts',(32.3282169135405,-31.8347765477019,1.2489945238531));
#20745=CARTESIAN_POINT('Ctrl Pts',(36.1661501715419,-31.025453813021,1.09199439650085));
#20746=CARTESIAN_POINT('Ctrl Pts',(38.9584254909315,-33.7800977501094,0.934994269148596));
#20747=CARTESIAN_POINT('Ctrl Pts',(38.201061889907,-37.6287344800703,0.777994141796343));
#20748=CARTESIAN_POINT('Ctrl Pts',(34.5734381895487,-39.1199689001796,0.620994014444089));
#20749=CARTESIAN_POINT('Ctrl Pts',(31.3279885395076,-36.9171722692834,0.463993887091836));
#20750=CARTESIAN_POINT('Ctrl Pts',(31.3759276866332,-32.994453947074,0.306993759739581));
#20751=CARTESIAN_POINT('Ctrl Pts',(34.6722754393756,-30.8716903339078,0.149993632387328));
#20752=CARTESIAN_POINT('Ctrl Pts',(38.2651837481491,-32.4476574497985,-0.00700649496492499));
#20753=CARTESIAN_POINT('Ctrl Pts',(38.9246971357756,-36.3188846782332,-0.164006622317179));
#20754=CARTESIAN_POINT('Ctrl Pts',(37.0258557525633,-38.0994349533404,-0.268673373885348));
#20755=CARTESIAN_POINT('Ctrl Pts',(35.9084720925035,-38.3981590173419,-0.321006749669432));
#20756=CARTESIAN_POINT('Ctrl Pts',(37.8143974874483,-32.5937287191406,8.10700224988981));
#20757=CARTESIAN_POINT('Ctrl Pts',(38.6056283266121,-33.5191597390956,8.05466887410573));
#20758=CARTESIAN_POINT('Ctrl Pts',(39.1911984442813,-36.1960819350737,7.95000212253756));
#20759=CARTESIAN_POINT('Ctrl Pts',(36.3106940741934,-39.1612015370487,7.7930019951853));
#20760=CARTESIAN_POINT('Ctrl Pts',(32.2540352290981,-38.3859857972091,7.63600186783306));
#20761=CARTESIAN_POINT('Ctrl Pts',(30.6601534543285,-34.5788711876989,7.47900174048079));
#20762=CARTESIAN_POINT('Ctrl Pts',(32.9576299321766,-31.1472373351772,7.32200161312855));
#20763=CARTESIAN_POINT('Ctrl Pts',(37.0866305057775,-31.1714790727616,7.16500148577629));
#20764=CARTESIAN_POINT('Ctrl Pts',(39.3444742481158,-34.6282630245248,7.00800135842403));
#20765=CARTESIAN_POINT('Ctrl Pts',(37.7066136711597,-38.4186497631728,6.85100123107179));
#20766=CARTESIAN_POINT('Ctrl Pts',(33.641693040528,-39.1433700868122,6.69400110371952));
#20767=CARTESIAN_POINT('Ctrl Pts',(30.7947860459719,-36.1527554141754,6.53700097636728));
#20768=CARTESIAN_POINT('Ctrl Pts',(31.718731394466,-32.1284217844307,6.38000084901502));
#20769=CARTESIAN_POINT('Ctrl Pts',(35.5850234445937,-30.6790758307459,6.22300072166277));
#20770=CARTESIAN_POINT('Ctrl Pts',(38.9267185335935,-33.1043361203307,6.06600059431051));
#20771=CARTESIAN_POINT('Ctrl Pts',(38.747287852214,-37.2294603242033,5.90900046695826));
#20772=CARTESIAN_POINT('Ctrl Pts',(35.2076280004405,-39.3554041176628,5.75200033960601));
#20773=CARTESIAN_POINT('Ctrl Pts',(31.481786229765,-37.5758162224347,5.59500021225375));
#20774=CARTESIAN_POINT('Ctrl Pts',(30.9107604489508,-33.4864687290921,5.4380000849015));
#20775=CARTESIAN_POINT('Ctrl Pts',(34.0065950288281,-30.7543194848738,5.28099995754925));
#20776=CARTESIAN_POINT('Ctrl Pts',(37.9932253643036,-31.8293125714861,5.123999830197));
#20777=CARTESIAN_POINT('Ctrl Pts',(39.2958018060318,-35.7474915521612,4.96699970284474));
#20778=CARTESIAN_POINT('Ctrl Pts',(36.7462915531952,-38.995387657759,4.80999957549249));
#20779=CARTESIAN_POINT('Ctrl Pts',(32.6308649129514,-38.6605813351003,4.65299944814023));
#20780=CARTESIAN_POINT('Ctrl Pts',(30.6398644329761,-35.0432966040406,4.49599932078798));
#20781=CARTESIAN_POINT('Ctrl Pts',(32.5586393455524,-31.3871873963525,4.33899919343573));
#20782=CARTESIAN_POINT('Ctrl Pts',(36.6666057781757,-30.9707219083004,4.18199906608348));
#20783=CARTESIAN_POINT('Ctrl Pts',(39.2801108208385,-34.167348741179,4.02499893873122));
#20784=CARTESIAN_POINT('Ctrl Pts',(38.0555994290271,-38.1106219453356,3.86799881137897));
#20785=CARTESIAN_POINT('Ctrl Pts',(34.0911027148519,-39.2645706097038,3.71099868402672));
#20786=CARTESIAN_POINT('Ctrl Pts',(30.9416229163962,-36.5944378951337,3.55399855667446));
#20787=CARTESIAN_POINT('Ctrl Pts',(31.4313287819664,-32.494557425059,3.39699842932221));
#20788=CARTESIAN_POINT('Ctrl Pts',(35.1210963673509,-30.6413313453092,3.23999830196996));
#20789=CARTESIAN_POINT('Ctrl Pts',(38.7022756737031,-32.6965652688994,3.0829981746177));
#20790=CARTESIAN_POINT('Ctrl Pts',(38.963588874858,-36.8173112029482,2.92599804726545));
#20791=CARTESIAN_POINT('Ctrl Pts',(35.6707138879638,-39.3084567691156,2.76899791991319));
#20792=CARTESIAN_POINT('Ctrl Pts',(31.7764033615041,-37.9361677720372,2.61199779256094));
#20793=CARTESIAN_POINT('Ctrl Pts',(30.7727227893853,-33.9309890559499,2.45499766520869));
#20794=CARTESIAN_POINT('Ctrl Pts',(33.5596824021932,-30.8844025266947,2.29799753785643));
#20795=CARTESIAN_POINT('Ctrl Pts',(37.6381883094267,-31.5283121023449,2.14099741050418));
#20796=CARTESIAN_POINT('Ctrl Pts',(39.3510060812057,-35.2853167815919,1.98399728315193));
#20797=CARTESIAN_POINT('Ctrl Pts',(37.1622336865094,-38.7864766566921,1.82699715579967));
#20798=CARTESIAN_POINT('Ctrl Pts',(33.0345681639462,-38.8922635836996,1.66999702844742));
#20799=CARTESIAN_POINT('Ctrl Pts',(30.6693190617512,-35.5078264672934,1.51299690109517));
#20800=CARTESIAN_POINT('Ctrl Pts',(32.187443504768,-31.6680042909403,1.35599677374291));
#20801=CARTESIAN_POINT('Ctrl Pts',(36.2275933836127,-30.8160392022689,1.19899664639066));
#20802=CARTESIAN_POINT('Ctrl Pts',(39.1669907193568,-33.715822398208,1.04199651903841));
#20803=CARTESIAN_POINT('Ctrl Pts',(38.3697224358239,-37.7672397035641,0.884996391686155));
#20804=CARTESIAN_POINT('Ctrl Pts',(34.5509631015021,-39.3370456789998,0.7279962643339));
#20805=CARTESIAN_POINT('Ctrl Pts',(31.1345141616793,-37.0181860368003,0.570996136981647));
#20806=CARTESIAN_POINT('Ctrl Pts',(31.1849791714726,-32.8887838589028,0.413996009629392));
#20807=CARTESIAN_POINT('Ctrl Pts',(34.6550079808865,-30.6541740890041,0.256995882277139));
#20808=CARTESIAN_POINT('Ctrl Pts',(38.4372228065685,-32.313177235829,0.0999957549248859));
#20809=CARTESIAN_POINT('Ctrl Pts',(39.1314852530455,-36.3883753089936,-0.0570043724273679));
#20810=CARTESIAN_POINT('Ctrl Pts',(37.1325959372044,-38.2627408840732,-0.161671123995537));
#20811=CARTESIAN_POINT('Ctrl Pts',(35.9563385206894,-38.5772044012455,-0.214004499779622));
#20812=CARTESIAN_POINT('Ctrl Pts',(37.9552630411254,-32.4732906012887,8.21400449977962));
#20813=CARTESIAN_POINT('Ctrl Pts',(38.7860963780679,-33.4450410745538,8.16167112399554));
#20814=CARTESIAN_POINT('Ctrl Pts',(39.400975311997,-36.2559479436168,8.05700437242737));
#20815=CARTESIAN_POINT('Ctrl Pts',(36.3762966222648,-39.369477006698,7.90000424507512));
#20816=CARTESIAN_POINT('Ctrl Pts',(32.1165948534739,-38.5554603530221,7.74300411772285));
#20817=CARTESIAN_POINT('Ctrl Pts',(30.4429364871958,-34.5577929485451,7.58600399037062));
#20818=CARTESIAN_POINT('Ctrl Pts',(32.8554057112908,-30.9543997746027,7.42900386301835));
#20819=CARTESIAN_POINT('Ctrl Pts',(37.191070039577,-30.9798548538712,7.2720037356661));
#20820=CARTESIAN_POINT('Ctrl Pts',(39.5619228399106,-34.6096569338406,7.11500360831384));
#20821=CARTESIAN_POINT('Ctrl Pts',(37.8420844548986,-38.5897592080416,6.9580034809616));
#20822=CARTESIAN_POINT('Ctrl Pts',(33.5737073836467,-39.3507530609551,6.80100335360933));
#20823=CARTESIAN_POINT('Ctrl Pts',(30.5843076772956,-36.2104528539991,6.64400322625709));
#20824=CARTESIAN_POINT('Ctrl Pts',(31.5544981186253,-31.9846942345494,6.48700309890483));
#20825=CARTESIAN_POINT('Ctrl Pts',(35.6143048989029,-30.4628059618972,6.33000297155259));
#20826=CARTESIAN_POINT('Ctrl Pts',(39.1232577157224,-33.0094548026823,6.17300284420032));
#20827=CARTESIAN_POINT('Ctrl Pts',(38.9348462125535,-37.3410487421046,6.01600271684808));
#20828=CARTESIAN_POINT('Ctrl Pts',(35.2180201477371,-39.5733997686886,5.85900258949581));
#20829=CARTESIAN_POINT('Ctrl Pts',(31.3056934308947,-37.7047403633785,5.70200246214358));
#20830=CARTESIAN_POINT('Ctrl Pts',(30.7060868035096,-33.4107138218927,5.54500233479131));
#20831=CARTESIAN_POINT('Ctrl Pts',(33.9568733594783,-30.5418156935059,5.38800220743906));
#20832=CARTESIAN_POINT('Ctrl Pts',(38.1430415683413,-31.6706140784174,5.2310020800868));
#20833=CARTESIAN_POINT('Ctrl Pts',(39.5108142563315,-35.7849048215497,5.07400195273456));
#20834=CARTESIAN_POINT('Ctrl Pts',(36.8336965226849,-39.1953638505585,4.9170018253823));
#20835=CARTESIAN_POINT('Ctrl Pts',(32.5122855270398,-38.8437998814671,4.76000169803005));
#20836=CARTESIAN_POINT('Ctrl Pts',(30.4216319645722,-35.0454636753686,4.60300157067779));
#20837=CARTESIAN_POINT('Ctrl Pts',(32.4364449427192,-31.2063597591713,4.44600144332554));
#20838=CARTESIAN_POINT('Ctrl Pts',(36.7500223342062,-30.7690494395616,4.28900131597329));
#20839=CARTESIAN_POINT('Ctrl Pts',(39.4943379096791,-34.1256730784068,4.13200118862103));
#20840=CARTESIAN_POINT('Ctrl Pts',(38.2085375649176,-38.266314055126,3.97500106126878));
#20841=CARTESIAN_POINT('Ctrl Pts',(34.0456108041041,-39.4780198835927,3.81800093391653));
#20842=CARTESIAN_POINT('Ctrl Pts',(30.7384939918355,-36.6742423214464,3.66100080656427));
#20843=CARTESIAN_POINT('Ctrl Pts',(31.2527104989195,-32.3691556091822,3.50400067921202));
#20844=CARTESIAN_POINT('Ctrl Pts',(35.1271574539286,-30.4231722984524,3.34700055185977));
#20845=CARTESIAN_POINT('Ctrl Pts',(38.8875810951892,-32.5812743015779,3.19000042450751));
#20846=CARTESIAN_POINT('Ctrl Pts',(39.1619734825387,-36.9082708310562,3.03300029715526));
#20847=CARTESIAN_POINT('Ctrl Pts',(35.7042842999643,-39.5241026226178,2.876000169803));
#20848=CARTESIAN_POINT('Ctrl Pts',(31.6150566692411,-38.083128143037,2.71900004245075));
#20849=CARTESIAN_POINT('Ctrl Pts',(30.5611401158378,-33.8774831744275,2.5619999150985));
#20850=CARTESIAN_POINT('Ctrl Pts',(33.487591968347,-30.6784096207976,2.40499978774624));
#20851=CARTESIAN_POINT('Ctrl Pts',(37.7702342832343,-31.3545480053834,2.24799966039399));
#20852=CARTESIAN_POINT('Ctrl Pts',(39.5687816027568,-35.2995973892856,2.09099953304174));
#20853=CARTESIAN_POINT('Ctrl Pts',(37.2704572927298,-38.9759964857528,1.93399940568948));
#20854=CARTESIAN_POINT('Ctrl Pts',(32.9361948371383,-39.087078234871,1.77699927833723));
#20855=CARTESIAN_POINT('Ctrl Pts',(30.4525608494213,-35.533244076855,1.61999915098498));
#20856=CARTESIAN_POINT('Ctrl Pts',(32.0466700959956,-31.5012320341786,1.46299902363273));
#20857=CARTESIAN_POINT('Ctrl Pts',(36.2890365956835,-30.606624591517,1.30599889628047));
#20858=CARTESIAN_POINT('Ctrl Pts',(39.3755559477821,-33.6515470463066,1.14899876892822));
#20859=CARTESIAN_POINT('Ctrl Pts',(38.5383829817409,-37.905744927058,0.991998641575965));
#20860=CARTESIAN_POINT('Ctrl Pts',(34.5284880134556,-39.55412245782,0.83499851422371));
#20861=CARTESIAN_POINT('Ctrl Pts',(30.9410397838509,-37.1191998043172,0.677998386871458));
#20862=CARTESIAN_POINT('Ctrl Pts',(30.9940306563121,-32.7831137707316,0.520998259519202));
#20863=CARTESIAN_POINT('Ctrl Pts',(34.6377405223973,-30.4366578441002,0.36399813216695));
#20864=CARTESIAN_POINT('Ctrl Pts',(38.6092618649879,-32.1786970218597,0.206998004814696));
#20865=CARTESIAN_POINT('Ctrl Pts',(39.3382733703155,-36.4578659397538,0.0499978774624431));
#20866=CARTESIAN_POINT('Ctrl Pts',(37.2393361218455,-38.4260468148059,-0.0546688741057264));
#20867=CARTESIAN_POINT('Ctrl Pts',(36.0042049488753,-38.756249785149,-0.107002249889811));
#20868=CARTESIAN_POINT('Ctrl Pts',(38.0961285948024,-32.3528524834367,8.32100674966943));
#20869=CARTESIAN_POINT('Ctrl Pts',(38.9665644295237,-33.3709224100119,8.26867337388535));
#20870=CARTESIAN_POINT('Ctrl Pts',(39.6107521797128,-36.3158139521599,8.16400662231718));
#20871=CARTESIAN_POINT('Ctrl Pts',(36.4418991703362,-39.5777524763472,8.00700649496493));
#20872=CARTESIAN_POINT('Ctrl Pts',(31.9791544778497,-38.724934908835,7.85000636761268));
#20873=CARTESIAN_POINT('Ctrl Pts',(30.2257195200631,-34.5367147093914,7.69300624026041));
#20874=CARTESIAN_POINT('Ctrl Pts',(32.753181490405,-30.7615622140283,7.53600611290817));
#20875=CARTESIAN_POINT('Ctrl Pts',(37.2955095733766,-30.7882306349807,7.3790059855559));
#20876=CARTESIAN_POINT('Ctrl Pts',(39.7793714317054,-34.5910508431566,7.22200585820367));
#20877=CARTESIAN_POINT('Ctrl Pts',(37.9775552386376,-38.7608686529102,7.0650057308514));
#20878=CARTESIAN_POINT('Ctrl Pts',(33.5057217267653,-39.5581360350982,6.90800560349915));
#20879=CARTESIAN_POINT('Ctrl Pts',(30.3738293086194,-36.2681502938228,6.7510054761469));
#20880=CARTESIAN_POINT('Ctrl Pts',(31.3902648427845,-31.8409666846681,6.59400534879465));
#20881=CARTESIAN_POINT('Ctrl Pts',(35.6435863532121,-30.2465360930486,6.43700522144239));
#20882=CARTESIAN_POINT('Ctrl Pts',(39.3197968978512,-32.9145734850341,6.28000509409014));
#20883=CARTESIAN_POINT('Ctrl Pts',(39.1224045728929,-37.4526371600059,6.12300496673789));
#20884=CARTESIAN_POINT('Ctrl Pts',(35.2284122950338,-39.7913954197145,5.96600483938562));
#20885=CARTESIAN_POINT('Ctrl Pts',(31.1296006320244,-37.8336645043222,5.80900471203338));
#20886=CARTESIAN_POINT('Ctrl Pts',(30.5014131580684,-33.3349589146933,5.65200458468112));
#20887=CARTESIAN_POINT('Ctrl Pts',(33.9071516901285,-30.3293119021379,5.49500445732887));
#20888=CARTESIAN_POINT('Ctrl Pts',(38.292857772379,-31.5119155853487,5.33800432997662));
#20889=CARTESIAN_POINT('Ctrl Pts',(39.7258267066312,-35.8223180909381,5.18100420262436));
#20890=CARTESIAN_POINT('Ctrl Pts',(36.9211014921746,-39.3953400433581,5.02400407527211));
#20891=CARTESIAN_POINT('Ctrl Pts',(32.3937061411281,-39.0270184278339,4.86700394791986));
#20892=CARTESIAN_POINT('Ctrl Pts',(30.2033994961682,-35.0476307466965,4.7100038205676));
#20893=CARTESIAN_POINT('Ctrl Pts',(32.314250539886,-31.02553212199,4.55300369321535));
#20894=CARTESIAN_POINT('Ctrl Pts',(36.8334388902368,-30.5673769708228,4.39600356586309));
#20895=CARTESIAN_POINT('Ctrl Pts',(39.7085649985197,-34.0839974156347,4.23900343851085));
#20896=CARTESIAN_POINT('Ctrl Pts',(38.3614757008081,-38.4220061649164,4.08200331115859));
#20897=CARTESIAN_POINT('Ctrl Pts',(34.0001188933562,-39.6914691574817,3.92500318380634));
#20898=CARTESIAN_POINT('Ctrl Pts',(30.5353650672746,-36.754046747759,3.76800305645408));
#20899=CARTESIAN_POINT('Ctrl Pts',(31.0740922158726,-32.2437537933055,3.61100292910183));
#20900=CARTESIAN_POINT('Ctrl Pts',(35.1332185405061,-30.2050132515957,3.45400280174957));
#20901=CARTESIAN_POINT('Ctrl Pts',(39.0728865166754,-32.4659833342563,3.29700267439732));
#20902=CARTESIAN_POINT('Ctrl Pts',(39.3603580902194,-36.9992304591644,3.14000254704507));
#20903=CARTESIAN_POINT('Ctrl Pts',(35.7378547119649,-39.73974847612,2.98300241969282));
#20904=CARTESIAN_POINT('Ctrl Pts',(31.453709976978,-38.2300885140369,2.82600229234056));
#20905=CARTESIAN_POINT('Ctrl Pts',(30.3495574422904,-33.8239772929051,2.66900216498831));
#20906=CARTESIAN_POINT('Ctrl Pts',(33.4155015345008,-30.4724167149005,2.51200203763606));
#20907=CARTESIAN_POINT('Ctrl Pts',(37.9022802570419,-31.180783908422,2.3550019102838));
#20908=CARTESIAN_POINT('Ctrl Pts',(39.7865571243079,-35.3138779969793,2.19800178293155));
#20909=CARTESIAN_POINT('Ctrl Pts',(37.3786808989502,-39.1655163148135,2.04100165557929));
#20910=CARTESIAN_POINT('Ctrl Pts',(32.8378215103303,-39.2818928860424,1.88400152822704));
#20911=CARTESIAN_POINT('Ctrl Pts',(30.2358026370915,-35.5586616864166,1.72700140087479));
#20912=CARTESIAN_POINT('Ctrl Pts',(31.9058966872231,-31.3344597774169,1.57000127352254));
#20913=CARTESIAN_POINT('Ctrl Pts',(36.3504798077544,-30.397209980765,1.41300114617028));
#20914=CARTESIAN_POINT('Ctrl Pts',(39.5841211762074,-33.5872716944053,1.25600101881803));
#20915=CARTESIAN_POINT('Ctrl Pts',(38.7070435276578,-38.0442501505519,1.09900089146578));
#20916=CARTESIAN_POINT('Ctrl Pts',(34.5060129254091,-39.7711992366401,0.942000764113522));
#20917=CARTESIAN_POINT('Ctrl Pts',(30.7475654060226,-37.220213571834,0.785000636761267));
#20918=CARTESIAN_POINT('Ctrl Pts',(30.8030821411515,-32.6774436825603,0.628000509409014));
#20919=CARTESIAN_POINT('Ctrl Pts',(34.6204730639081,-30.2191415991965,0.471000382056761));
#20920=CARTESIAN_POINT('Ctrl Pts',(38.7813009234074,-32.0442168078902,0.314000254704507));
#20921=CARTESIAN_POINT('Ctrl Pts',(39.5450614875854,-36.5273565705141,0.157000127352254));
#20922=CARTESIAN_POINT('Ctrl Pts',(37.3460763064866,-38.5893527455387,0.0523333757840845));
#20923=CARTESIAN_POINT('Ctrl Pts',(36.0520713770612,-38.9352951690526,0.));
#20924=CARTESIAN_POINT('Ctrl Pts',(36.0520713770612,-38.9352951690526,0.));
#20925=CARTESIAN_POINT('Ctrl Pts',(36.1681792863691,-38.8956805730896,-1.36202072051053E-17));
#20926=CARTESIAN_POINT('Ctrl Pts',(36.2820221354364,-38.8505155517789,2.68655360649277E-15));
#20927=CARTESIAN_POINT('Ctrl Pts',(36.3933740322884,-38.80015771728,1.94289029309402E-15));
#20928=CARTESIAN_POINT('Ctrl Pts',(36.5072231634749,-38.7486705323445,1.18254920758684E-15));
#20929=CARTESIAN_POINT('Ctrl Pts',(36.6184689861953,-38.6917545108625,4.54098351417643E-16));
#20930=CARTESIAN_POINT('Ctrl Pts',(36.7268457946485,-38.6297432931302,1.66533453693773E-16));
#20931=CARTESIAN_POINT('Ctrl Pts',(36.8407841942848,-38.56454983515,-1.35788460984399E-16));
#20932=CARTESIAN_POINT('Ctrl Pts',(36.9515525365026,-38.4937243961273,-1.82271800722416E-15));
#20933=CARTESIAN_POINT('Ctrl Pts',(37.0588029145039,-38.4176084656939,-1.99840144432528E-15));
#20934=CARTESIAN_POINT('Ctrl Pts',(37.1526469952551,-38.3510070265646,-2.15212445178876E-15));
#20935=CARTESIAN_POINT('Ctrl Pts',(37.2437973301633,-38.2803539972376,-9.7785017405382E-16));
#20936=CARTESIAN_POINT('Ctrl Pts',(37.3319893511255,-38.2058560072044,-8.88178419700125E-16));
#20937=CARTESIAN_POINT('Ctrl Pts',(37.3493647837374,-38.1911785478217,-8.70511452689226E-16));
#20938=CARTESIAN_POINT('Ctrl Pts',(37.3666252839799,-38.1763517900465,-1.48427532953915E-15));
#20939=CARTESIAN_POINT('Ctrl Pts',(37.3837686739948,-38.1613772431262,-1.55431223447522E-15));
#20940=CARTESIAN_POINT('Ctrl Pts',(37.3963029962073,-38.1504286620158,-1.60551944217877E-15));
#20941=CARTESIAN_POINT('Ctrl Pts',(37.4087735029071,-38.139402069251,-1.97641509759958E-15));
#20942=CARTESIAN_POINT('Ctrl Pts',(37.4211705433933,-38.1283061781123,-1.88737914186277E-15));
#20943=CARTESIAN_POINT('Ctrl Pts',(37.5137497678178,-38.0454437403337,-1.22247208301798E-15));
#20944=CARTESIAN_POINT('Ctrl Pts',(37.6023731431382,-37.9585995914834,-1.41571360075421E-15));
#20945=CARTESIAN_POINT('Ctrl Pts',(37.6867792446409,-37.8680946551148,-1.63757896132211E-15));
#20946=CARTESIAN_POINT('Ctrl Pts',(37.7709936181979,-37.7777953001582,-1.85894035607411E-15));
#20947=CARTESIAN_POINT('Ctrl Pts',(37.8510103725839,-37.6838510649778,4.27670315709133E-16));
#20948=CARTESIAN_POINT('Ctrl Pts',(37.9265294316329,-37.5865486541875,7.49400541621981E-16));
#20949=CARTESIAN_POINT('Ctrl Pts',(38.0010161819357,-37.4905763199493,1.06673287208574E-15));
#20950=CARTESIAN_POINT('Ctrl Pts',(38.0711277582919,-37.3913363066692,-2.10142620498032E-15));
#20951=CARTESIAN_POINT('Ctrl Pts',(38.1365301844556,-37.2890828938187,-2.44249065417534E-15));
#20952=CARTESIAN_POINT('Ctrl Pts',(38.1898358473465,-37.2057421635956,-2.72047218512562E-15));
#20953=CARTESIAN_POINT('Ctrl Pts',(38.2400125268915,-37.1203991308186,-6.32482117348439E-16));
#20954=CARTESIAN_POINT('Ctrl Pts',(38.2868534572638,-37.0331856293588,-5.55111512312578E-16));
#20955=CARTESIAN_POINT('Ctrl Pts',(38.2987532893997,-37.0110292370944,-5.35455685563087E-16));
#20956=CARTESIAN_POINT('Ctrl Pts',(38.3104377056016,-36.9887521084602,-5.70989169773688E-17));
#20957=CARTESIAN_POINT('Ctrl Pts',(38.3219030525931,-36.9663563797929,-2.77555756156289E-17));
#20958=CARTESIAN_POINT('Ctrl Pts',(38.3300600637675,-36.9504229580542,-6.87928085047562E-18));
#20959=CARTESIAN_POINT('Ctrl Pts',(38.3381024804697,-36.9344366850298,-1.37102362174578E-15));
#20960=CARTESIAN_POINT('Ctrl Pts',(38.3460266349626,-36.9184039879293,-1.33226762955019E-15));
#20961=CARTESIAN_POINT('Ctrl Pts',(38.3989875306322,-36.8112498430667,-1.07324288929609E-15));
#20962=CARTESIAN_POINT('Ctrl Pts',(38.4467095755205,-36.7019458397232,2.38645293041498E-15));
#20963=CARTESIAN_POINT('Ctrl Pts',(38.4889139708526,-36.5907545955107,1.9151347174784E-15));
#20964=CARTESIAN_POINT('Ctrl Pts',(38.5302822088046,-36.4817662825029,1.45315430452751E-15));
#20965=CARTESIAN_POINT('Ctrl Pts',(38.5663495354543,-36.3709641352684,1.27266374069395E-15));
#20966=CARTESIAN_POINT('Ctrl Pts',(38.5968051838807,-36.2585816849604,1.52655665885959E-15));
#20967=CARTESIAN_POINT('Ctrl Pts',(38.6012594551821,-36.2421452618648,1.56368960455097E-15));
#20968=CARTESIAN_POINT('Ctrl Pts',(38.6055936009628,-36.2256750205659,1.48568813827467E-15));
#20969=CARTESIAN_POINT('Ctrl Pts',(38.6098065549286,-36.2091716785531,1.47104550762833E-15));
#20970=CARTESIAN_POINT('Ctrl Pts',(38.6394751128162,-36.092951477284,1.34152120378576E-15));
#20971=CARTESIAN_POINT('Ctrl Pts',(38.6631376928158,-35.9750893748381,9.72065328759131E-16));
#20972=CARTESIAN_POINT('Ctrl Pts',(38.6808851493713,-35.856021209443,1.41553435639707E-15));
#20973=CARTESIAN_POINT('Ctrl Pts',(38.6908686963668,-35.7890413229915,1.66500074413739E-15));
#20974=CARTESIAN_POINT('Ctrl Pts',(38.6989794822973,-35.7216798344703,1.48644827793188E-15));
#20975=CARTESIAN_POINT('Ctrl Pts',(38.7052266318381,-35.6540157826807,1.55431223447522E-15));
#20976=CARTESIAN_POINT('Ctrl Pts',(38.7081091139172,-35.6227950770761,1.58562517764618E-15));
#20977=CARTESIAN_POINT('Ctrl Pts',(38.7105947647117,-35.591509978624,7.00070747597251E-16));
#20978=CARTESIAN_POINT('Ctrl Pts',(38.7126841330784,-35.5601683863959,6.66133814775094E-16));
#20979=CARTESIAN_POINT('Ctrl Pts',(38.7138852254902,-35.5421513870013,6.46624860231182E-16));
#20980=CARTESIAN_POINT('Ctrl Pts',(38.7149548469422,-35.5241227721236,2.63074882680395E-16));
#20981=CARTESIAN_POINT('Ctrl Pts',(38.7158930667035,-35.5060923822785,2.77555756156289E-16));
#20982=CARTESIAN_POINT('Ctrl Pts',(38.7222040106739,-35.3848107969113,3.74961486578641E-16));
#20983=CARTESIAN_POINT('Ctrl Pts',(38.7225824292358,-35.263331928612,-1.41858650592555E-15));
#20984=CARTESIAN_POINT('Ctrl Pts',(38.717186529709,-35.1421030264707,-9.99200722162641E-16));
#20985=CARTESIAN_POINT('Ctrl Pts',(38.7119025633842,-35.0233889115555,-5.88514728574682E-16));
#20986=CARTESIAN_POINT('Ctrl Pts',(38.7010808603444,-34.9049135759813,2.80055440532142E-15));
#20987=CARTESIAN_POINT('Ctrl Pts',(38.6848166129475,-34.7871029976449,2.56739074444567E-15));
#20988=CARTESIAN_POINT('Ctrl Pts',(38.6687112711112,-34.6704434566446,2.3365051479245E-15));
#20989=CARTESIAN_POINT('Ctrl Pts',(38.6472688652681,-34.5544349100609,2.77413847088875E-15));
#20990=CARTESIAN_POINT('Ctrl Pts',(38.6205350417295,-34.4395098718885,3.02535774210355E-15));
#20991=CARTESIAN_POINT('Ctrl Pts',(38.6031281553353,-34.3646800563773,3.18893125068641E-15));
#20992=CARTESIAN_POINT('Ctrl Pts',(38.583477007896,-34.2903100135713,5.83132516188889E-16));
#20993=CARTESIAN_POINT('Ctrl Pts',(38.5615843988617,-34.2165260396906,2.91433543964104E-16));
#20994=CARTESIAN_POINT('Ctrl Pts',(38.5541960449916,-34.1916253022719,1.92990492842735E-16));
#20995=CARTESIAN_POINT('Ctrl Pts',(38.5465523399986,-34.1667913689833,-1.55624678416612E-15));
#20996=CARTESIAN_POINT('Ctrl Pts',(38.5386532038413,-34.1420292711584,-1.62370117351429E-15));
#20997=CARTESIAN_POINT('Ctrl Pts',(38.5335667843701,-34.1260844369365,-1.66713646980058E-15));
#20998=CARTESIAN_POINT('Ctrl Pts',(38.5283752457655,-34.1101719998602,9.92420310992954E-16));
#20999=CARTESIAN_POINT('Ctrl Pts',(38.5230814471938,-34.0943013261403,9.71445146547012E-16));
#21000=CARTESIAN_POINT('Ctrl Pts',(38.4861837828756,-33.9836830652666,8.25248693044116E-16));
#21001=CARTESIAN_POINT('Ctrl Pts',(38.4442854059965,-33.8749762815042,4.28212832527473E-15));
#21002=CARTESIAN_POINT('Ctrl Pts',(38.3974511090383,-33.7686001708186,3.23352455922077E-15));
#21003=CARTESIAN_POINT('Ctrl Pts',(38.359337050901,-33.6820305940251,2.38016393467622E-15));
#21004=CARTESIAN_POINT('Ctrl Pts',(38.3179530879923,-33.5970047635678,1.69064823388315E-15));
#21005=CARTESIAN_POINT('Ctrl Pts',(38.2733131581435,-33.5137642691618,1.70696790036118E-15));
#21006=CARTESIAN_POINT('Ctrl Pts',(38.251698175988,-33.473458609917,1.71487000282641E-15));
#21007=CARTESIAN_POINT('Ctrl Pts',(38.2293195396252,-33.4335717773559,1.04902033086069E-15));
#21008=CARTESIAN_POINT('Ctrl Pts',(38.2061773582038,-33.3941327240688,1.01307850997046E-15));
#21009=CARTESIAN_POINT('Ctrl Pts',(38.1925909929398,-33.3709787536688,9.91977702834968E-16));
#21010=CARTESIAN_POINT('Ctrl Pts',(38.1787393972074,-33.347976051224,-1.47665884113671E-16));
#21011=CARTESIAN_POINT('Ctrl Pts',(38.1646366459175,-33.3251529677485,-1.38777878078145E-17));
#21012=CARTESIAN_POINT('Ctrl Pts',(38.1062051944783,-33.230590859521,5.40441897174675E-16));
#21013=CARTESIAN_POINT('Ctrl Pts',(38.0434224756675,-33.1390339550006,1.08623518571526E-16));
#21014=CARTESIAN_POINT('Ctrl Pts',(37.9763225348264,-33.0508729636923,6.24500451351651E-16));
#21015=CARTESIAN_POINT('Ctrl Pts',(37.9162918094667,-32.9720000438309,1.08602792936337E-15));
#21016=CARTESIAN_POINT('Ctrl Pts',(37.8528049873413,-32.8958452375375,9.00746847309969E-16));
#21017=CARTESIAN_POINT('Ctrl Pts',(37.7858629582169,-32.8227148526165,3.72098185597025E-16));
#21018=CARTESIAN_POINT('Ctrl Pts',(37.7510080319419,-32.784637814794,1.2084137301326E-16));
#21019=CARTESIAN_POINT('Ctrl Pts',(37.7152160018646,-32.7473811866193,3.2434591796547E-16));
#21020=CARTESIAN_POINT('Ctrl Pts',(37.6785242770714,-32.7109603660126,2.77555756156289E-16));
#21021=CARTESIAN_POINT('Ctrl Pts',(37.6735319337713,-32.7141668369925,8.));
#21022=CARTESIAN_POINT('Ctrl Pts',(37.7506744257016,-32.7912795331857,8.));
#21023=CARTESIAN_POINT('Ctrl Pts',(37.8237045554225,-32.8720144016735,8.));
#21024=CARTESIAN_POINT('Ctrl Pts',(37.8926300182219,-32.9559529391151,8.));
#21025=CARTESIAN_POINT('Ctrl Pts',(37.9633153902931,-33.0420347223805,8.));
#21026=CARTESIAN_POINT('Ctrl Pts',(38.0296841818896,-33.1314863178634,8.));
#21027=CARTESIAN_POINT('Ctrl Pts',(38.0917148195566,-33.2239024768849,8.));
#21028=CARTESIAN_POINT('Ctrl Pts',(38.1550365108844,-33.3182421083212,8.));
#21029=CARTESIAN_POINT('Ctrl Pts',(38.2138380035849,-33.4156715766502,8.));
#21030=CARTESIAN_POINT('Ctrl Pts',(38.268059557232,-33.515799249106,8.));
#21031=CARTESIAN_POINT('Ctrl Pts',(38.3198487844224,-33.6114352910132,8.));
#21032=CARTESIAN_POINT('Ctrl Pts',(38.3674597504585,-33.7095337219438,8.));
#21033=CARTESIAN_POINT('Ctrl Pts',(38.410804885236,-33.8097778917925,8.));
#21034=CARTESIAN_POINT('Ctrl Pts',(38.4178421610283,-33.8260529794907,8.));
#21035=CARTESIAN_POINT('Ctrl Pts',(38.4247669147912,-33.8423846664997,8.));
#21036=CARTESIAN_POINT('Ctrl Pts',(38.4315786781863,-33.8587716403974,8.));
#21037=CARTESIAN_POINT('Ctrl Pts',(38.4380889335058,-33.8744332800934,8.));
#21038=CARTESIAN_POINT('Ctrl Pts',(38.4444929624372,-33.8901382301107,8.));
#21039=CARTESIAN_POINT('Ctrl Pts',(38.4507885504088,-33.9058798359799,8.));
#21040=CARTESIAN_POINT('Ctrl Pts',(38.4941738374283,-34.014361218793,8.));
#21041=CARTESIAN_POINT('Ctrl Pts',(38.5324452713943,-34.124659589853,8.));
#21042=CARTESIAN_POINT('Ctrl Pts',(38.5655742382515,-34.2363431431182,8.));
#21043=CARTESIAN_POINT('Ctrl Pts',(38.5991377517882,-34.3494916293961,8.));
#21044=CARTESIAN_POINT('Ctrl Pts',(38.6274234029538,-34.4640626260336,8.));
#21045=CARTESIAN_POINT('Ctrl Pts',(38.6503587972893,-34.5796396359417,8.));
#21046=CARTESIAN_POINT('Ctrl Pts',(38.6743337296149,-34.7004551296896,8.));
#21047=CARTESIAN_POINT('Ctrl Pts',(38.692463198861,-34.8223707151795,8.));
#21048=CARTESIAN_POINT('Ctrl Pts',(38.7046087858744,-34.9449340325394,8.));
#21049=CARTESIAN_POINT('Ctrl Pts',(38.7137179761345,-35.0368565205594,8.));
#21050=CARTESIAN_POINT('Ctrl Pts',(38.7194601094409,-35.1291439544571,8.));
#21051=CARTESIAN_POINT('Ctrl Pts',(38.721753661108,-35.2216089483748,8.));
#21052=CARTESIAN_POINT('Ctrl Pts',(38.7223012285573,-35.2436842395473,8.));
#21053=CARTESIAN_POINT('Ctrl Pts',(38.7226520798176,-35.2657741780712,8.));
#21054=CARTESIAN_POINT('Ctrl Pts',(38.7228050031224,-35.2878471504668,8.));
#21055=CARTESIAN_POINT('Ctrl Pts',(38.723639797835,-35.4083415425535,8.));
#21056=CARTESIAN_POINT('Ctrl Pts',(38.7185864406144,-35.528481112922,8.));
#21057=CARTESIAN_POINT('Ctrl Pts',(38.7075759731584,-35.6478398239672,8.));
#21058=CARTESIAN_POINT('Ctrl Pts',(38.6966361565965,-35.766432645673,8.));
#21059=CARTESIAN_POINT('Ctrl Pts',(38.6798156826268,-35.8842554734363,8.));
#21060=CARTESIAN_POINT('Ctrl Pts',(38.6569974768235,-36.0009032638125,8.));
#21061=CARTESIAN_POINT('Ctrl Pts',(38.6541238330716,-36.0155934720123,8.));
#21062=CARTESIAN_POINT('Ctrl Pts',(38.6511549977698,-36.0302650508608,8.));
#21063=CARTESIAN_POINT('Ctrl Pts',(38.6480906778903,-36.0449171950576,8.));
#21064=CARTESIAN_POINT('Ctrl Pts',(38.6241801879288,-36.1592459728997,8.));
#21065=CARTESIAN_POINT('Ctrl Pts',(38.5944604969197,-36.2723920187216,8.));
#21066=CARTESIAN_POINT('Ctrl Pts',(38.5592377490131,-36.3840888412668,8.));
#21067=CARTESIAN_POINT('Ctrl Pts',(38.5372725083531,-36.4537440423509,8.));
#21068=CARTESIAN_POINT('Ctrl Pts',(38.5131661119788,-36.5228355678477,8.));
#21069=CARTESIAN_POINT('Ctrl Pts',(38.4869829521143,-36.5912966040202,8.));
#21070=CARTESIAN_POINT('Ctrl Pts',(38.4780335436947,-36.614696597631,8.));
#21071=CARTESIAN_POINT('Ctrl Pts',(38.4688414510417,-36.6380229129432,8.));
#21072=CARTESIAN_POINT('Ctrl Pts',(38.4594090583389,-36.6612728133014,8.));
#21073=CARTESIAN_POINT('Ctrl Pts',(38.4526597990907,-36.677909059263,8.));
#21074=CARTESIAN_POINT('Ctrl Pts',(38.4457869585498,-36.6945073015523,8.));
#21075=CARTESIAN_POINT('Ctrl Pts',(38.4387984803451,-36.7110502346119,8.));
#21076=CARTESIAN_POINT('Ctrl Pts',(38.3928771569434,-36.8197539261443,8.));
#21077=CARTESIAN_POINT('Ctrl Pts',(38.3419028069428,-36.9262312105814,8.));
#21078=CARTESIAN_POINT('Ctrl Pts',(38.286233868877,-37.0302277419135,8.));
#21079=CARTESIAN_POINT('Ctrl Pts',(38.2286497374683,-37.1378020936858,8.));
#21080=CARTESIAN_POINT('Ctrl Pts',(38.1660422723199,-37.2427227531059,8.));
#21081=CARTESIAN_POINT('Ctrl Pts',(38.0987528117336,-37.3447008755076,8.));
#21082=CARTESIAN_POINT('Ctrl Pts',(38.0308301924039,-37.447638558876,8.));
#21083=CARTESIAN_POINT('Ctrl Pts',(37.9581366181552,-37.5475788135467,8.));
#21084=CARTESIAN_POINT('Ctrl Pts',(37.8809726402855,-37.6442062900679,8.));
#21085=CARTESIAN_POINT('Ctrl Pts',(37.8265596140724,-37.7123442160536,8.));
#21086=CARTESIAN_POINT('Ctrl Pts',(37.7699226008246,-37.7788344950898,8.));
#21087=CARTESIAN_POINT('Ctrl Pts',(37.7111539331996,-37.8435580680838,8.));
#21088=CARTESIAN_POINT('Ctrl Pts',(37.6849210722466,-37.8724490496109,8.));
#21089=CARTESIAN_POINT('Ctrl Pts',(37.6582633448569,-37.9009879055023,8.));
#21090=CARTESIAN_POINT('Ctrl Pts',(37.6311883528209,-37.9291634733987,8.));
#21091=CARTESIAN_POINT('Ctrl Pts',(37.6195660136439,-37.9412582509764,8.));
#21092=CARTESIAN_POINT('Ctrl Pts',(37.6078682053827,-37.9532845462101,8.));
#21093=CARTESIAN_POINT('Ctrl Pts',(37.5961020337617,-37.9652350938879,8.));
#21094=CARTESIAN_POINT('Ctrl Pts',(37.507659771091,-38.055063247923,8.));
#21095=CARTESIAN_POINT('Ctrl Pts',(37.415258178228,-38.1407187695167,8.));
#21096=CARTESIAN_POINT('Ctrl Pts',(37.3192259922681,-38.2218835091588,8.));
#21097=CARTESIAN_POINT('Ctrl Pts',(37.2371862486548,-38.2912220789739,8.));
#21098=CARTESIAN_POINT('Ctrl Pts',(37.152495821289,-38.3572831262055,8.));
#21099=CARTESIAN_POINT('Ctrl Pts',(37.0653354498859,-38.4198507239943,8.));
#21100=CARTESIAN_POINT('Ctrl Pts',(37.0262246732672,-38.4479261819266,8.));
#21101=CARTESIAN_POINT('Ctrl Pts',(36.9866162962358,-38.4752979774627,8.));
#21102=CARTESIAN_POINT('Ctrl Pts',(36.9465254062051,-38.5019452444609,8.));
#21103=CARTESIAN_POINT('Ctrl Pts',(36.9192921690604,-38.5200463976374,8.));
#21104=CARTESIAN_POINT('Ctrl Pts',(36.8918306415648,-38.5378166037371,8.));
#21105=CARTESIAN_POINT('Ctrl Pts',(36.8641755127457,-38.555230549143,8.));
#21106=CARTESIAN_POINT('Ctrl Pts',(36.7573712570443,-38.6224832996203,8.));
#21107=CARTESIAN_POINT('Ctrl Pts',(36.6476202687202,-38.6844692470865,8.));
#21108=CARTESIAN_POINT('Ctrl Pts',(36.5352245224892,-38.7408547353335,8.));
#21109=CARTESIAN_POINT('Ctrl Pts',(36.4331307539574,-38.7920720382892,8.));
#21110=CARTESIAN_POINT('Ctrl Pts',(36.3288540451722,-38.8386685245707,8.));
#21111=CARTESIAN_POINT('Ctrl Pts',(36.2225973607791,-38.8803650263204,8.));
#21112=CARTESIAN_POINT('Ctrl Pts',(36.1671668634624,-38.9021166727374,8.));
#21113=CARTESIAN_POINT('Ctrl Pts',(36.1111972101676,-38.9225343520043,8.));
#21114=CARTESIAN_POINT('Ctrl Pts',(36.054732523776,-38.9416301760088,8.));
#21115=CARTESIAN_POINT('Ctrl Pts',(31.4836965554877,-35.0029832498286,6.38741669750802));
#21116=CARTESIAN_POINT('Ctrl Pts',(31.4810524495825,-35.31689356108,6.4016107071645));
#21117=CARTESIAN_POINT('Ctrl Pts',(31.519709060091,-35.6301638289998,6.41580471682099));
#21118=CARTESIAN_POINT('Ctrl Pts',(31.6022835043847,-35.9313947240647,6.42999872647747));
#21119=CARTESIAN_POINT('Ctrl Pts',(31.9067358422351,-37.0420343537909,6.48233210226155));
#21120=CARTESIAN_POINT('Ctrl Pts',(32.8082072698223,-37.98901073323,6.53466547804564));
#21121=CARTESIAN_POINT('Ctrl Pts',(33.9025203486177,-38.3477577905554,6.58699885382972));
#21122=CARTESIAN_POINT('Ctrl Pts',(34.9968334274131,-38.7065048478808,6.6393322296138));
#21123=CARTESIAN_POINT('Ctrl Pts',(36.2839881574169,-38.4770225830925,6.69166560539789));
#21124=CARTESIAN_POINT('Ctrl Pts',(37.1868793172355,-37.7621695835158,6.74399898118197));
#21125=CARTESIAN_POINT('Ctrl Pts',(38.0897704770541,-37.0473165839391,6.79633235696606));
#21126=CARTESIAN_POINT('Ctrl Pts',(38.6083980666875,-35.847092849574,6.84866573275014));
#21127=CARTESIAN_POINT('Ctrl Pts',(38.5102394141138,-34.6996866784653,6.90099910853423));
#21128=CARTESIAN_POINT('Ctrl Pts',(38.41208076154,-33.5522805073566,6.95333248431831));
#21129=CARTESIAN_POINT('Ctrl Pts',(37.697135866759,-32.4576918995043,7.0056658601024));
#21130=CARTESIAN_POINT('Ctrl Pts',(36.6859406162159,-31.9065595295948,7.05799923588648));
#21131=CARTESIAN_POINT('Ctrl Pts',(35.6747453656728,-31.3554271596853,7.11033261167057));
#21132=CARTESIAN_POINT('Ctrl Pts',(34.3672997593676,-31.3477510277185,7.16266598745465));
#21133=CARTESIAN_POINT('Ctrl Pts',(33.3498296676148,-31.8872253835852,7.21499936323873));
#21134=CARTESIAN_POINT('Ctrl Pts',(32.332359575862,-32.426699739452,7.26733273902282));
#21135=CARTESIAN_POINT('Ctrl Pts',(31.6048649986616,-33.5133245831523,7.3196661148069));
#21136=CARTESIAN_POINT('Ctrl Pts',(31.4934685739382,-34.6593973074264,7.37199949059099));
#21137=CARTESIAN_POINT('Ctrl Pts',(31.4825295909021,-34.7719401481876,7.37713855956333));
#21138=CARTESIAN_POINT('Ctrl Pts',(31.4775316317653,-34.8850562438399,7.38227762853568));
#21139=CARTESIAN_POINT('Ctrl Pts',(31.478260520576,-34.9982347527286,7.38741669750802));
#21140=CARTESIAN_POINT('Ctrl Pts',(33.9479286229388,-38.9352951690526,8.));
#21141=CARTESIAN_POINT('Ctrl Pts',(32.6539236935135,-38.5893527455387,7.94766662421592));
#21142=CARTESIAN_POINT('Ctrl Pts',(30.4549361873396,-36.5273716142364,7.84299987264774));
#21143=CARTESIAN_POINT('Ctrl Pts',(31.2187010881653,-32.044211167377,7.68599974529549));
#21144=CARTESIAN_POINT('Ctrl Pts',(35.3795267558193,-30.2191465582126,7.52899961794324));
#21145=CARTESIAN_POINT('Ctrl Pts',(39.1969165266342,-32.6774422642514,7.37199949059099));
#21146=CARTESIAN_POINT('Ctrl Pts',(39.2524336251343,-37.2202141105436,7.21499936323873));
#21147=CARTESIAN_POINT('Ctrl Pts',(35.4939867861423,-39.7711972931265,7.05799923588648));
#21148=CARTESIAN_POINT('Ctrl Pts',(31.292957592828,-38.0442496611363,6.90099910853423));
#21149=CARTESIAN_POINT('Ctrl Pts',(30.4158800177777,-33.5872718945856,6.74399898118197));
#21150=CARTESIAN_POINT('Ctrl Pts',(33.6495206016122,-30.3972113452741,6.58699885382972));
#21151=CARTESIAN_POINT('Ctrl Pts',(38.09410244091,-31.3344607296745,6.42999872647747));
#21152=CARTESIAN_POINT('Ctrl Pts',(39.7641960678496,-35.558661561786,6.27299859912521));
#21153=CARTESIAN_POINT('Ctrl Pts',(37.1621778889461,-39.2818916953666,6.11599847177296));
#21154=CARTESIAN_POINT('Ctrl Pts',(32.6213197580022,-39.1655151793351,5.95899834442071));
#21155=CARTESIAN_POINT('Ctrl Pts',(30.2134441875202,-35.3138779065921,5.80199821706845));
#21156=CARTESIAN_POINT('Ctrl Pts',(32.0977205408613,-31.1807849590781,5.6449980897162));
#21157=CARTESIAN_POINT('Ctrl Pts',(36.584498029893,-30.4724179566463,5.48799796236395));
#21158=CARTESIAN_POINT('Ctrl Pts',(39.6504412814188,-33.8239776163473,5.33099783501169));
#21159=CARTESIAN_POINT('Ctrl Pts',(38.5462890493217,-38.2300876270061,5.17399770765944));
#21160=CARTESIAN_POINT('Ctrl Pts',(34.2621454906851,-39.7397471751372,5.01699758030718));
#21161=CARTESIAN_POINT('Ctrl Pts',(30.6396431067263,-36.9992299102556,4.85999745295493));
#21162=CARTESIAN_POINT('Ctrl Pts',(30.9271146014312,-32.4659840299328,4.70299732560268));
#21163=CARTESIAN_POINT('Ctrl Pts',(34.8667814960507,-30.2050145678827,4.54599719825042));
#21164=CARTESIAN_POINT('Ctrl Pts',(38.9259067064028,-32.2437545499559,4.38899707089817));
#21165=CARTESIAN_POINT('Ctrl Pts',(39.4646337070995,-36.7540462662356,4.23199694354592));
#21166=CARTESIAN_POINT('Ctrl Pts',(35.9998808321606,-39.6914678695931,4.07499681619366));
#21167=CARTESIAN_POINT('Ctrl Pts',(31.6385252219761,-38.4220052255121,3.91799668884141));
#21168=CARTESIAN_POINT('Ctrl Pts',(30.291436294066,-34.0839976670965,3.76099656148916));
#21169=CARTESIAN_POINT('Ctrl Pts',(33.1665616130745,-30.567378187653,3.6039964341369));
#21170=CARTESIAN_POINT('Ctrl Pts',(37.6857487228281,-31.0255332130596,3.44699630678465));
#21171=CARTESIAN_POINT('Ctrl Pts',(39.7965991870786,-35.0476307336073,3.28999617943239));
#21172=CARTESIAN_POINT('Ctrl Pts',(37.606293143399,-39.0270173223719,3.13299605208014));
#21173=CARTESIAN_POINT('Ctrl Pts',(33.0788990351993,-39.3953388367078,2.97599592472789));
#21174=CARTESIAN_POINT('Ctrl Pts',(30.2741745906988,-35.8223178652953,2.81899579737564));
#21175=CARTESIAN_POINT('Ctrl Pts',(31.7071431315558,-31.5119165427019,2.66199567002338));
#21176=CARTESIAN_POINT('Ctrl Pts',(36.092848009894,-30.329313184686,2.50499554267113));
#21177=CARTESIAN_POINT('Ctrl Pts',(39.4985856069267,-33.3349593710879,2.34799541531888));
#21178=CARTESIAN_POINT('Ctrl Pts',(38.8703983056154,-37.8336637277424,2.19099528796662));
#21179=CARTESIAN_POINT('Ctrl Pts',(34.7715877673847,-39.7913941019012,2.03399516061437));
#21180=CARTESIAN_POINT('Ctrl Pts',(30.8775965593863,-37.4526364914204,1.87699503326212));
#21181=CARTESIAN_POINT('Ctrl Pts',(30.6802042867265,-32.914574048659,1.71999490590986));
#21182=CARTESIAN_POINT('Ctrl Pts',(34.3564138261785,-30.2465374145616,1.56299477855761));
#21183=CARTESIAN_POINT('Ctrl Pts',(38.6097341605507,-31.8409675209513,1.40599465120535));
#21184=CARTESIAN_POINT('Ctrl Pts',(39.6261694334752,-36.2681500029269,1.2489945238531));
#21185=CARTESIAN_POINT('Ctrl Pts',(36.4942778376799,-39.5581346787212,1.09199439650085));
#21186=CARTESIAN_POINT('Ctrl Pts',(32.0224456319375,-38.7608678116187,0.934994269148595));
#21187=CARTESIAN_POINT('Ctrl Pts',(30.2206297689144,-34.5910506117954,0.777994141796339));
#21188=CARTESIAN_POINT('Ctrl Pts',(32.704491289799,-30.7882324000235,0.620994014444087));
#21189=CARTESIAN_POINT('Ctrl Pts',(37.2468174060219,-30.7615623188695,0.463993887091833));
#21190=CARTESIAN_POINT('Ctrl Pts',(39.7742801854456,-34.536716632844,0.306993759739581));
#21191=CARTESIAN_POINT('Ctrl Pts',(38.0208425645948,-38.7249309242138,0.149993632387326));
#21192=CARTESIAN_POINT('Ctrl Pts',(33.5581056824257,-39.5777559852671,-0.00700649496492666));
#21193=CARTESIAN_POINT('Ctrl Pts',(30.3892373827997,-36.3158028716181,-0.16400662231718));
#21194=CARTESIAN_POINT('Ctrl Pts',(31.0334355704763,-33.370922410012,-0.26867337388535));
#21195=CARTESIAN_POINT('Ctrl Pts',(31.9038714051976,-32.3528524834368,-0.321006749669435));
#21196=CARTESIAN_POINT('Ctrl Pts',(33.9957950511247,-38.756249785149,8.10700224988981));
#21197=CARTESIAN_POINT('Ctrl Pts',(32.7606638781546,-38.426046814806,8.05466887410573));
#21198=CARTESIAN_POINT('Ctrl Pts',(30.6617244103942,-36.4578802990271,7.95000212253756));
#21199=CARTESIAN_POINT('Ctrl Pts',(31.3907400550635,-32.1786916379746,7.79300199518531));
#21200=CARTESIAN_POINT('Ctrl Pts',(35.3622593055321,-30.4366625774945,7.63600186783305));
#21201=CARTESIAN_POINT('Ctrl Pts',(39.0059680720859,-32.7831124169518,7.4790017404808));
#21202=CARTESIAN_POINT('Ctrl Pts',(39.0589592913856,-37.1192003185169,7.32200161312853));
#21203=CARTESIAN_POINT('Ctrl Pts',(35.4715117112195,-39.554120602731,7.16500148577629));
#21204=CARTESIAN_POINT('Ctrl Pts',(31.4616180877658,-37.9057444599095,7.00800135842404));
#21205=CARTESIAN_POINT('Ctrl Pts',(30.6244451918799,-33.6515472373793,6.85100123107178));
#21206=CARTESIAN_POINT('Ctrl Pts',(33.7109637950579,-30.6066258939446,6.69400110371953));
#21207=CARTESIAN_POINT('Ctrl Pts',(37.9533290718052,-31.5012329431111,6.53700097636728));
#21208=CARTESIAN_POINT('Ctrl Pts',(39.5474379144414,-35.5332439578948,6.38000084901502));
#21209=CARTESIAN_POINT('Ctrl Pts',(37.0638045894695,-39.0870770983678,6.22300072166277));
#21210=CARTESIAN_POINT('Ctrl Pts',(32.729543334333,-38.9759954019356,6.06600059431052));
#21211=CARTESIAN_POINT('Ctrl Pts',(30.4312196493866,-35.2995973030108,5.90900046695826));
#21212=CARTESIAN_POINT('Ctrl Pts',(32.2297664783665,-31.3545490082375,5.752000339606));
#21213=CARTESIAN_POINT('Ctrl Pts',(36.5124076158656,-30.6784108060473,5.59500021225375));
#21214=CARTESIAN_POINT('Ctrl Pts',(39.4388586659392,-33.8774834831539,5.4380000849015));
#21215=CARTESIAN_POINT('Ctrl Pts',(38.3849424013594,-38.0831272963638,5.28099995754925));
#21216=CARTESIAN_POINT('Ctrl Pts',(34.2957158934656,-39.5241013808263,5.123999830197));
#21217=CARTESIAN_POINT('Ctrl Pts',(30.8380276599492,-36.9082703071214,4.96699970284474));
#21218=CARTESIAN_POINT('Ctrl Pts',(31.1124199720466,-32.581274965603,4.80999957549249));
#21219=CARTESIAN_POINT('Ctrl Pts',(34.8728425809651,-30.4231735548519,4.65299944814024));
#21220=CARTESIAN_POINT('Ctrl Pts',(38.7472884723895,-32.3691563314071,4.49599932078798));
#21221=CARTESIAN_POINT('Ctrl Pts',(39.2615048383014,-36.674241861831,4.33899919343573));
#21222=CARTESIAN_POINT('Ctrl Pts',(35.954388933901,-39.4780186542996,4.18199906608348));
#21223=CARTESIAN_POINT('Ctrl Pts',(31.7914633158823,-38.2663131584621,4.02499893873122));
#21224=CARTESIAN_POINT('Ctrl Pts',(30.5056633240975,-34.1256733184278,3.86799881137897));
#21225=CARTESIAN_POINT('Ctrl Pts',(33.2499781462058,-30.7690506010293,3.71099868402671));
#21226=CARTESIAN_POINT('Ctrl Pts',(37.5635543535394,-31.2063608006002,3.55399855667446));
#21227=CARTESIAN_POINT('Ctrl Pts',(39.5783667785835,-35.0454636628748,3.39699842932221));
#21228=CARTESIAN_POINT('Ctrl Pts',(37.4877137900394,-38.8437988263006,3.23999830196995));
#21229=CARTESIAN_POINT('Ctrl Pts',(33.1663039806949,-39.1953626988076,3.0829981746177));
#21230=CARTESIAN_POINT('Ctrl Pts',(30.4891869819735,-35.784904606173,2.92599804726545));
#21231=CARTESIAN_POINT('Ctrl Pts',(31.856959294467,-31.6706149922136,2.76899791991319));
#21232=CARTESIAN_POINT('Ctrl Pts',(36.0431263541924,-30.5418169177014,2.61199779256094));
#21233=CARTESIAN_POINT('Ctrl Pts',(39.2939120176749,-33.4107142575226,2.45499766520869));
#21234=CARTESIAN_POINT('Ctrl Pts',(38.6943055550796,-37.704739622131,2.29799753785643));
#21235=CARTESIAN_POINT('Ctrl Pts',(34.7819799118415,-39.5733985108324,2.14099741050418));
#21236=CARTESIAN_POINT('Ctrl Pts',(31.0651548682101,-37.3410481039379,1.98399728315193));
#21237=CARTESIAN_POINT('Ctrl Pts',(30.8767434149602,-33.0094553406639,1.82699715579967));
#21238=CARTESIAN_POINT('Ctrl Pts',(34.3856952723259,-30.4628072232849,1.66999702844742));
#21239=CARTESIAN_POINT('Ctrl Pts',(38.4455009300555,-31.9846950327841,1.51299690109516));
#21240=CARTESIAN_POINT('Ctrl Pts',(39.4156911220303,-36.2104525763381,1.35599677374291));
#21241=CARTESIAN_POINT('Ctrl Pts',(36.4262922006151,-39.3507517662898,1.19899664639066));
#21242=CARTESIAN_POINT('Ctrl Pts',(32.1579163760677,-38.5897584050265,1.04199651903841));
#21243=CARTESIAN_POINT('Ctrl Pts',(30.4380783060842,-34.6096567130058,0.884996391686151));
#21244=CARTESIAN_POINT('Ctrl Pts',(32.8089307843264,-30.9798565386092,0.727996264333898));
#21245=CARTESIAN_POINT('Ctrl Pts',(37.1445932353457,-30.9543998746739,0.570996136981644));
#21246=CARTESIAN_POINT('Ctrl Pts',(39.5570632317115,-34.5577947844858,0.413996009629391));
#21247=CARTESIAN_POINT('Ctrl Pts',(37.8834023235315,-38.5554565496905,0.256995882277137));
#21248=CARTESIAN_POINT('Ctrl Pts',(33.6237080097094,-39.3694803559713,0.0999957549248841));
#21249=CARTESIAN_POINT('Ctrl Pts',(30.5990147253931,-36.25593736721,-0.0570043724273687));
#21250=CARTESIAN_POINT('Ctrl Pts',(31.2139036219321,-33.4450410745538,-0.161671123995539));
#21251=CARTESIAN_POINT('Ctrl Pts',(32.0447369588746,-32.4732906012887,-0.214004499779624));
#21252=CARTESIAN_POINT('Ctrl Pts',(34.0436614793107,-38.5772044012455,8.21400449977962));
#21253=CARTESIAN_POINT('Ctrl Pts',(32.8674040627957,-38.2627408840732,8.16167112399554));
#21254=CARTESIAN_POINT('Ctrl Pts',(30.8685126334489,-36.3883889838178,8.05700437242737));
#21255=CARTESIAN_POINT('Ctrl Pts',(31.5627790219617,-32.3131721085722,7.90000424507511));
#21256=CARTESIAN_POINT('Ctrl Pts',(35.3449918552448,-30.6541785967763,7.74300411772285));
#21257=CARTESIAN_POINT('Ctrl Pts',(38.8150196175374,-32.8887825696523,7.58600399037061));
#21258=CARTESIAN_POINT('Ctrl Pts',(38.8654849576371,-37.0181865264902,7.42900386301835));
#21259=CARTESIAN_POINT('Ctrl Pts',(35.4490366362965,-39.3370439123355,7.2720037356661));
#21260=CARTESIAN_POINT('Ctrl Pts',(31.6302785827036,-37.7672392586828,7.11500360831385));
#21261=CARTESIAN_POINT('Ctrl Pts',(30.833010365982,-33.715822580173,6.95800348096159));
#21262=CARTESIAN_POINT('Ctrl Pts',(33.7724069885036,-30.8160404426151,6.80100335360934));
#21263=CARTESIAN_POINT('Ctrl Pts',(37.8125557027003,-31.6680051565476,6.64400322625708));
#21264=CARTESIAN_POINT('Ctrl Pts',(39.3306797610333,-35.5078263540035,6.48700309890484));
#21265=CARTESIAN_POINT('Ctrl Pts',(36.9654312899929,-38.892262501369,6.33000297155257));
#21266=CARTESIAN_POINT('Ctrl Pts',(32.8377669106638,-38.7864756245362,6.17300284420034));
#21267=CARTESIAN_POINT('Ctrl Pts',(30.6489951112531,-35.2853166994296,6.01600271684807));
#21268=CARTESIAN_POINT('Ctrl Pts',(32.3618124158715,-31.5283130573969,5.85900258949582));
#21269=CARTESIAN_POINT('Ctrl Pts',(36.4403172018384,-30.8844036554483,5.70200246214356));
#21270=CARTESIAN_POINT('Ctrl Pts',(39.2272760504595,-33.9309893499606,5.54500233479132));
#21271=CARTESIAN_POINT('Ctrl Pts',(38.2235957533972,-37.9361669657214,5.38800220743906));
#21272=CARTESIAN_POINT('Ctrl Pts',(34.3292862962461,-39.3084555865154,5.23100208008681));
#21273=CARTESIAN_POINT('Ctrl Pts',(31.0364122131721,-36.8173107039871,5.07400195273455));
#21274=CARTESIAN_POINT('Ctrl Pts',(31.2977253426618,-32.6965659012732,4.9170018253823));
#21275=CARTESIAN_POINT('Ctrl Pts',(34.8789036658794,-30.6413325418211,4.76000169803005));
#21276=CARTESIAN_POINT('Ctrl Pts',(38.5686702383762,-32.4945581128583,4.60300157067779));
#21277=CARTESIAN_POINT('Ctrl Pts',(39.0583759695033,-36.5944374574263,4.44600144332554));
#21278=CARTESIAN_POINT('Ctrl Pts',(35.9088970356414,-39.2645694390062,4.28900131597328));
#21279=CARTESIAN_POINT('Ctrl Pts',(31.9444014097886,-38.1106210914121,4.13200118862103));
#21280=CARTESIAN_POINT('Ctrl Pts',(30.7198903541289,-34.1673489697591,3.97500106126878));
#21281=CARTESIAN_POINT('Ctrl Pts',(33.333394679337,-30.9707230144056,3.81800093391652));
#21282=CARTESIAN_POINT('Ctrl Pts',(37.4413599842507,-31.3871883881407,3.66100080656427));
#21283=CARTESIAN_POINT('Ctrl Pts',(39.3601343700882,-35.0432965921423,3.50400067921202));
#21284=CARTESIAN_POINT('Ctrl Pts',(37.36913443668,-38.6605803302294,3.34700055185977));
#21285=CARTESIAN_POINT('Ctrl Pts',(33.2537089261905,-38.9953865609073,3.19000042450751));
#21286=CARTESIAN_POINT('Ctrl Pts',(30.7041993732481,-35.7474913470507,3.03300029715526));
#21287=CARTESIAN_POINT('Ctrl Pts',(32.006775457378,-31.8293134417253,2.876000169803));
#21288=CARTESIAN_POINT('Ctrl Pts',(35.9934046984909,-30.7543206507168,2.71900004245075));
#21289=CARTESIAN_POINT('Ctrl Pts',(39.0892384284232,-33.4864691439573,2.5619999150985));
#21290=CARTESIAN_POINT('Ctrl Pts',(38.5182128045439,-37.5758155165195,2.40499978774624));
#21291=CARTESIAN_POINT('Ctrl Pts',(34.7923720562983,-39.3554029197635,2.24799966039399));
#21292=CARTESIAN_POINT('Ctrl Pts',(31.2527131770338,-37.2294597164554,2.09099953304174));
#21293=CARTESIAN_POINT('Ctrl Pts',(31.073282543194,-33.1043366326688,1.93399940568948));
#21294=CARTESIAN_POINT('Ctrl Pts',(34.4149767184733,-30.6790770320082,1.77699927833723));
#21295=CARTESIAN_POINT('Ctrl Pts',(38.2812676995604,-32.1284225446167,1.61999915098497));
#21296=CARTESIAN_POINT('Ctrl Pts',(39.2052128105854,-36.1527551497494,1.46299902363272));
#21297=CARTESIAN_POINT('Ctrl Pts',(36.3583065635504,-39.1433688538583,1.30599889628047));
#21298=CARTESIAN_POINT('Ctrl Pts',(32.2933871201978,-38.4186489984343,1.14899876892821));
#21299=CARTESIAN_POINT('Ctrl Pts',(30.655526843254,-34.6282628142162,0.991998641575962));
#21300=CARTESIAN_POINT('Ctrl Pts',(32.9133702788538,-31.1714806771949,0.834998514223709));
#21301=CARTESIAN_POINT('Ctrl Pts',(37.0423690646695,-31.1472374304784,0.677998386871454));
#21302=CARTESIAN_POINT('Ctrl Pts',(39.3398462779774,-34.5788729361276,0.520998259519202));
#21303=CARTESIAN_POINT('Ctrl Pts',(37.7459620824681,-38.385982175167,0.363998132166948));
#21304=CARTESIAN_POINT('Ctrl Pts',(33.6893103369932,-39.1612047266757,0.206998004814695));
#21305=CARTESIAN_POINT('Ctrl Pts',(30.8087920679866,-36.1960718628018,0.0499978774624421));
#21306=CARTESIAN_POINT('Ctrl Pts',(31.3943716733879,-33.5191597390956,-0.0546688741057282));
#21307=CARTESIAN_POINT('Ctrl Pts',(32.1856025125517,-32.5937287191406,-0.107002249889813));
#21308=CARTESIAN_POINT('Ctrl Pts',(34.0915279074966,-38.398159017342,8.32100674966943));
#21309=CARTESIAN_POINT('Ctrl Pts',(32.9741442474368,-38.0994349533405,8.26867337388535));
#21310=CARTESIAN_POINT('Ctrl Pts',(31.0753008565035,-36.3188976686085,8.16400662231718));
#21311=CARTESIAN_POINT('Ctrl Pts',(31.73481798886,-32.4476525791699,8.00700649496493));
#21312=CARTESIAN_POINT('Ctrl Pts',(35.3277244049576,-30.8716946160581,7.85000636761267));
#21313=CARTESIAN_POINT('Ctrl Pts',(38.6240711629891,-32.9944527223528,7.69300624026043));
#21314=CARTESIAN_POINT('Ctrl Pts',(38.6720106238885,-36.9171727344635,7.53600611290815));
#21315=CARTESIAN_POINT('Ctrl Pts',(35.4265615613737,-39.1199672219399,7.37900598555592));
#21316=CARTESIAN_POINT('Ctrl Pts',(31.7989390776415,-37.628734057456,7.22200585820365));
#21317=CARTESIAN_POINT('Ctrl Pts',(31.0415755400842,-33.7800979229667,7.06500573085141));
#21318=CARTESIAN_POINT('Ctrl Pts',(33.8338501819494,-31.0254549912856,6.90800560349915));
#21319=CARTESIAN_POINT('Ctrl Pts',(37.6717823335954,-31.8347773699841,6.75100547614689));
#21320=CARTESIAN_POINT('Ctrl Pts',(39.1139216076251,-35.4824087501123,6.59400534879465));
#21321=CARTESIAN_POINT('Ctrl Pts',(36.8670579905162,-38.6974479043702,6.43700522144239));
#21322=CARTESIAN_POINT('Ctrl Pts',(32.9459904869947,-38.5969558471367,6.28000509409014));
#21323=CARTESIAN_POINT('Ctrl Pts',(30.8667705731195,-35.2710360958482,6.12300496673788));
#21324=CARTESIAN_POINT('Ctrl Pts',(32.4938583533767,-31.7020771065563,5.96600483938563));
#21325=CARTESIAN_POINT('Ctrl Pts',(36.3682267878111,-31.0903965048492,5.80900471203338));
#21326=CARTESIAN_POINT('Ctrl Pts',(39.0156934349799,-33.9844952167673,5.65200458468112));
#21327=CARTESIAN_POINT('Ctrl Pts',(38.0622491054349,-37.789206635079,5.49500445732887));
#21328=CARTESIAN_POINT('Ctrl Pts',(34.3628566990267,-39.0928097922045,5.33800432997662));
#21329=CARTESIAN_POINT('Ctrl Pts',(31.234796766395,-36.7263511008529,5.18100420262436));
#21330=CARTESIAN_POINT('Ctrl Pts',(31.4830307132771,-32.8118568369433,5.02400407527211));
#21331=CARTESIAN_POINT('Ctrl Pts',(34.8849647507938,-30.8594915287904,4.86700394791986));
#21332=CARTESIAN_POINT('Ctrl Pts',(38.3900520043628,-32.6199598943095,4.7100038205676));
#21333=CARTESIAN_POINT('Ctrl Pts',(38.8552471007052,-36.5146330530217,4.55300369321535));
#21334=CARTESIAN_POINT('Ctrl Pts',(35.8634051373818,-39.0511202237127,4.39600356586309));
#21335=CARTESIAN_POINT('Ctrl Pts',(32.0973395036949,-37.9549290243621,4.23900343851084));
#21336=CARTESIAN_POINT('Ctrl Pts',(30.9341173841603,-34.2090246210904,4.08200331115859));
#21337=CARTESIAN_POINT('Ctrl Pts',(33.4168112124683,-31.1723954277819,3.92500318380634));
#21338=CARTESIAN_POINT('Ctrl Pts',(37.319165614962,-31.5680159756812,3.76800305645408));
#21339=CARTESIAN_POINT('Ctrl Pts',(39.141901961593,-35.0411295214099,3.61100292910183));
#21340=CARTESIAN_POINT('Ctrl Pts',(37.2505550833205,-38.4773618341581,3.45400280174957));
#21341=CARTESIAN_POINT('Ctrl Pts',(33.3411138716861,-38.7954104230071,3.29700267439732));
#21342=CARTESIAN_POINT('Ctrl Pts',(30.9192117645227,-35.7100780879284,3.14000254704507));
#21343=CARTESIAN_POINT('Ctrl Pts',(32.1565916202891,-31.988011891237,2.98300241969282));
#21344=CARTESIAN_POINT('Ctrl Pts',(35.9436830427893,-30.9668243837322,2.82600229234056));
#21345=CARTESIAN_POINT('Ctrl Pts',(38.8845648391714,-33.5622240303919,2.66900216498831));
#21346=CARTESIAN_POINT('Ctrl Pts',(38.3421200540082,-37.4468914109081,2.51200203763606));
#21347=CARTESIAN_POINT('Ctrl Pts',(34.802764200755,-39.1374073286946,2.3550019102838));
#21348=CARTESIAN_POINT('Ctrl Pts',(31.4402714858577,-37.1178713289729,2.19800178293155));
#21349=CARTESIAN_POINT('Ctrl Pts',(31.2698216714276,-33.1992179246737,2.04100165557929));
#21350=CARTESIAN_POINT('Ctrl Pts',(34.4442581646208,-30.8953468407316,1.88400152822704));
#21351=CARTESIAN_POINT('Ctrl Pts',(38.1170344690652,-32.2721500564494,1.72700140087478));
#21352=CARTESIAN_POINT('Ctrl Pts',(38.9947344991405,-36.0950577231607,1.57000127352253));
#21353=CARTESIAN_POINT('Ctrl Pts',(36.2903209264856,-38.9359859414268,1.41300114617028));
#21354=CARTESIAN_POINT('Ctrl Pts',(32.428857864328,-38.247539591842,1.25600101881803));
#21355=CARTESIAN_POINT('Ctrl Pts',(30.8729753804238,-34.6468689154266,1.09900089146577));
#21356=CARTESIAN_POINT('Ctrl Pts',(33.0178097733811,-31.3631048157807,0.942000764113519));
#21357=CARTESIAN_POINT('Ctrl Pts',(36.9401448939934,-31.3400749862829,0.785000636761266));
#21358=CARTESIAN_POINT('Ctrl Pts',(39.1226293242432,-34.5999510877694,0.628000509409013));
#21359=CARTESIAN_POINT('Ctrl Pts',(37.6085218414048,-38.2165078006437,0.471000382056759));
#21360=CARTESIAN_POINT('Ctrl Pts',(33.754912664277,-38.9529290973799,0.314000254704506));
#21361=CARTESIAN_POINT('Ctrl Pts',(31.0185694105801,-36.1362063583937,0.157000127352253));
#21362=CARTESIAN_POINT('Ctrl Pts',(31.5748397248436,-33.5932784036374,0.0523333757840826));
#21363=CARTESIAN_POINT('Ctrl Pts',(32.3264680662287,-32.7141668369925,-2.22044604925031E-15));
#21364=CARTESIAN_POINT('Ctrl Pts',(32.3264680662287,-32.7141668369925,-2.27595720048157E-15));
#21365=CARTESIAN_POINT('Ctrl Pts',(32.2493253090815,-32.7912797983002,-2.16394166852401E-15));
#21366=CARTESIAN_POINT('Ctrl Pts',(32.1762949026186,-32.8720149145437,3.46363794187806E-16));
#21367=CARTESIAN_POINT('Ctrl Pts',(32.1073691591848,-32.9559536860909,1.66533453693773E-16));
#21368=CARTESIAN_POINT('Ctrl Pts',(32.0366835341849,-33.0420356669728,-1.78884963425382E-17));
#21369=CARTESIAN_POINT('Ctrl Pts',(31.9703144812951,-33.1314874423946,-2.24888209125886E-15));
#21370=CARTESIAN_POINT('Ctrl Pts',(31.9082835820817,-33.2239037683368,-2.33146835171283E-15));
#21371=CARTESIAN_POINT('Ctrl Pts',(31.8449616802408,-33.3182434860262,-2.41577341812641E-15));
#21372=CARTESIAN_POINT('Ctrl Pts',(31.7861599686898,-33.4156730215343,-2.34515801197777E-15));
#21373=CARTESIAN_POINT('Ctrl Pts',(31.7319381963941,-33.5158007480848,-2.77555756156289E-15));
#21374=CARTESIAN_POINT('Ctrl Pts',(31.6801489223982,-33.611436542441,-3.18664851741706E-15));
#21375=CARTESIAN_POINT('Ctrl Pts',(31.6325378836028,-33.7095346984804,-3.69832300465041E-15));
#21376=CARTESIAN_POINT('Ctrl Pts',(31.5891926568309,-33.8097785742014,-3.99680288865056E-15));
#21377=CARTESIAN_POINT('Ctrl Pts',(31.5821541452564,-33.8260564375806,-4.04527083482939E-15));
#21378=CARTESIAN_POINT('Ctrl Pts',(31.5752281942475,-33.8423909194022,-5.19848407519141E-15));
#21379=CARTESIAN_POINT('Ctrl Pts',(31.568415272417,-33.8587807065962,-5.21804821573824E-15));
#21380=CARTESIAN_POINT('Ctrl Pts',(31.561906348996,-33.8744391674425,-5.23673938757109E-15));
#21381=CARTESIAN_POINT('Ctrl Pts',(31.5555036120846,-33.8901409126424,-5.57046258471252E-15));
#21382=CARTESIAN_POINT('Ctrl Pts',(31.5492092706946,-33.9058793019477,-5.49560397189452E-15));
#21383=CARTESIAN_POINT('Ctrl Pts',(31.5058237133564,-34.0143606742329,-4.97961946494936E-15));
#21384=CARTESIAN_POINT('Ctrl Pts',(31.4675520206245,-34.1246590298884,-6.38605598306829E-15));
#21385=CARTESIAN_POINT('Ctrl Pts',(31.4344228151864,-34.2363425690307,-5.19029264012261E-15));
#21386=CARTESIAN_POINT('Ctrl Pts',(31.4008590997118,-34.3494909069217,-3.9788461207494E-15));
#21387=CARTESIAN_POINT('Ctrl Pts',(31.3725732548101,-34.4640617531158,-1.67269218670119E-15));
#21388=CARTESIAN_POINT('Ctrl Pts',(31.3496376837557,-34.5796386183165,-1.85962356624714E-15));
#21389=CARTESIAN_POINT('Ctrl Pts',(31.3256626239872,-34.7004536721242,-2.05502707229468E-15));
#21390=CARTESIAN_POINT('Ctrl Pts',(31.3075330179638,-34.8223688186784,-6.90474885500916E-16));
#21391=CARTESIAN_POINT('Ctrl Pts',(31.2953872940185,-34.9449317101526,1.11022302462516E-16));
#21392=CARTESIAN_POINT('Ctrl Pts',(31.2862780010595,-35.0368538787582,7.12145193435089E-16));
#21393=CARTESIAN_POINT('Ctrl Pts',(31.2805357649583,-35.1291410005731,-7.33619512718545E-16));
#21394=CARTESIAN_POINT('Ctrl Pts',(31.2782421142109,-35.2216056948398,-3.88578058618805E-16));
#21395=CARTESIAN_POINT('Ctrl Pts',(31.2776945327762,-35.2436805246709,-3.0620357564075E-16));
#21396=CARTESIAN_POINT('Ctrl Pts',(31.2773436607928,-35.2657700018002,-4.90649572448904E-16));
#21397=CARTESIAN_POINT('Ctrl Pts',(31.2771907100455,-35.287842514156,-5.27355936696949E-16));
#21398=CARTESIAN_POINT('Ctrl Pts',(31.2763557493203,-35.4083367336975,-7.27736602069211E-16));
#21399=CARTESIAN_POINT('Ctrl Pts',(31.2814089690861,-35.5284761575602,-1.32546033095374E-15));
#21400=CARTESIAN_POINT('Ctrl Pts',(31.2924193361456,-35.6478347566642,-1.0547118733939E-15));
#21401=CARTESIAN_POINT('Ctrl Pts',(31.3033590399359,-35.7664273260093,-7.85701048289603E-16));
#21402=CARTESIAN_POINT('Ctrl Pts',(31.3201794237171,-35.8842499373544,-3.19095490877261E-16));
#21403=CARTESIAN_POINT('Ctrl Pts',(31.3429975699143,-36.0008975571309,1.94289029309402E-16));
#21404=CARTESIAN_POINT('Ctrl Pts',(31.3458712257766,-36.0155878441288,2.58943292776536E-16));
#21405=CARTESIAN_POINT('Ctrl Pts',(31.3488400749734,-36.030259502248,-2.41414676176044E-15));
#21406=CARTESIAN_POINT('Ctrl Pts',(31.3519044105546,-36.0449117261916,-2.44249065417534E-15));
#21407=CARTESIAN_POINT('Ctrl Pts',(31.375814852164,-36.1592403092631,-2.71916393553799E-15));
#21408=CARTESIAN_POINT('Ctrl Pts',(31.4055345217229,-36.272386206175,5.65793814005205E-16));
#21409=CARTESIAN_POINT('Ctrl Pts',(31.4407572695548,-36.384082920097,4.44089209850063E-16));
#21410=CARTESIAN_POINT('Ctrl Pts',(31.4627225424769,-36.453738155898,3.68192949317207E-16));
#21411=CARTESIAN_POINT('Ctrl Pts',(31.4868289857256,-36.52282973013,-1.13814971295829E-15));
#21412=CARTESIAN_POINT('Ctrl Pts',(31.513012205469,-36.5912908274846,-1.69309011255336E-15));
#21413=CARTESIAN_POINT('Ctrl Pts',(31.5219624105717,-36.6146928715758,-1.88278528544959E-15));
#21414=CARTESIAN_POINT('Ctrl Pts',(31.531155343526,-36.6380212260425,4.03667916851762E-15));
#21415=CARTESIAN_POINT('Ctrl Pts',(31.5405886194687,-36.6612731534534,4.32986979603811E-15));
#21416=CARTESIAN_POINT('Ctrl Pts',(31.5473370498667,-36.6779072490427,4.53961416853196E-15));
#21417=CARTESIAN_POINT('Ctrl Pts',(31.5542090296369,-36.6945033501966,3.07759665647771E-15));
#21418=CARTESIAN_POINT('Ctrl Pts',(31.561196617679,-36.7110441569158,2.94209101525666E-15));
#21419=CARTESIAN_POINT('Ctrl Pts',(31.6071179522689,-36.8197477489354,2.0515691568155E-15));
#21420=CARTESIAN_POINT('Ctrl Pts',(31.6580923235038,-36.9262249725842,4.21341387307547E-15));
#21421=CARTESIAN_POINT('Ctrl Pts',(31.7137612878297,-37.0302214764794,3.42781358853017E-15));
#21422=CARTESIAN_POINT('Ctrl Pts',(31.7713455134326,-37.1377959250922,2.61518514166327E-15));
#21423=CARTESIAN_POINT('Ctrl Pts',(31.8339530898433,-37.2427167108642,9.07249106506457E-16));
#21424=CARTESIAN_POINT('Ctrl Pts',(31.9012426720394,-37.3446949826671,6.80011602582908E-16));
#21425=CARTESIAN_POINT('Ctrl Pts',(31.9691654564611,-37.4476328810058,4.50635769240332E-16));
#21426=CARTESIAN_POINT('Ctrl Pts',(32.0418592122967,-37.5475733704053,-1.57902851375934E-15));
#21427=CARTESIAN_POINT('Ctrl Pts',(32.1190233809196,-37.6442010945393,-1.81799020282369E-15));
#21428=CARTESIAN_POINT('Ctrl Pts',(32.1734366012044,-37.712339269715,-1.98649684598102E-15));
#21429=CARTESIAN_POINT('Ctrl Pts',(32.2300738179544,-37.7788298007494,1.23701449661782E-16));
#21430=CARTESIAN_POINT('Ctrl Pts',(32.2888426956766,-37.8435536257978,-3.88578058618805E-16));
#21431=CARTESIAN_POINT('Ctrl Pts',(32.3150744390812,-37.8724433857632,-6.17236238483284E-16));
#21432=CARTESIAN_POINT('Ctrl Pts',(32.3417310110036,-37.9009810526196,1.30430196317008E-16));
#21433=CARTESIAN_POINT('Ctrl Pts',(32.3688048104485,-37.9291554653168,-2.77555756156289E-17));
#21434=CARTESIAN_POINT('Ctrl Pts',(32.3804263297313,-37.9412494265322,-9.56573491554205E-17));
#21435=CARTESIAN_POINT('Ctrl Pts',(32.392123309834,-37.9532749179279,-6.28475541027777E-16));
#21436=CARTESIAN_POINT('Ctrl Pts',(32.4038886430803,-37.9652246721857,-5.96744875736022E-16));
#21437=CARTESIAN_POINT('Ctrl Pts',(32.4923309120516,-38.05505326931,-3.5821937240873E-16));
#21438=CARTESIAN_POINT('Ctrl Pts',(32.5847325176906,-38.1407092470896,2.11600168392725E-15));
#21439=CARTESIAN_POINT('Ctrl Pts',(32.6807647145451,-38.221874449736,1.96370697480575E-15));
#21440=CARTESIAN_POINT('Ctrl Pts',(32.7628051861864,-38.2912140225467,1.8336013417573E-15));
#21441=CARTESIAN_POINT('Ctrl Pts',(32.8474963866317,-38.3572760203649,1.20960812321559E-15));
#21442=CARTESIAN_POINT('Ctrl Pts',(32.9346575664231,-38.4198445069104,5.62050406216485E-16));
#21443=CARTESIAN_POINT('Ctrl Pts',(32.973768957553,-38.4479205443796,2.71475138541893E-16));
#21444=CARTESIAN_POINT('Ctrl Pts',(33.0133779626213,-38.4752928979382,3.47992543175087E-15));
#21445=CARTESIAN_POINT('Ctrl Pts',(33.0534694930906,-38.5019407001488,3.78169717762944E-15));
#21446=CARTESIAN_POINT('Ctrl Pts',(33.0807047104967,-38.5200432439556,3.98669855846499E-15));
#21447=CARTESIAN_POINT('Ctrl Pts',(33.108168250427,-38.5378147929466,1.27528005472796E-15));
#21448=CARTESIAN_POINT('Ctrl Pts',(33.1358254185318,-38.5552300293176,1.47104550762833E-15));
#21449=CARTESIAN_POINT('Ctrl Pts',(33.2426299049644,-38.6224829515854,2.22703862229035E-15));
#21450=CARTESIAN_POINT('Ctrl Pts',(33.3523811032195,-38.6844690524263,5.56024339803508E-15));
#21451=CARTESIAN_POINT('Ctrl Pts',(33.4647770313827,-38.7408546683214,3.76781938982163E-15));
#21452=CARTESIAN_POINT('Ctrl Pts',(33.5668706528472,-38.7920719305417,2.13969049592827E-15));
#21453=CARTESIAN_POINT('Ctrl Pts',(33.6711471781243,-38.8386683831236,1.86420798495096E-15));
#21454=CARTESIAN_POINT('Ctrl Pts',(33.7774036389012,-38.880364855251,2.14498557804532E-15));
#21455=CARTESIAN_POINT('Ctrl Pts',(33.8328341927383,-38.9021165541705,2.26717202503918E-15));
#21456=CARTESIAN_POINT('Ctrl Pts',(33.8888038950002,-38.9225342787199,1.50877474080585E-16));
#21457=CARTESIAN_POINT('Ctrl Pts',(33.94526862329,-38.9416301412996,1.94289029309402E-16));
#21458=CARTESIAN_POINT('Ctrl Pts',(31.4846885160394,-34.9971888045819,7.11258330249198));
#21459=CARTESIAN_POINT('Ctrl Pts',(31.4819573643756,-34.6461972356202,7.09672411194512));
#21460=CARTESIAN_POINT('Ctrl Pts',(31.5304047798457,-34.2959415119622,7.08086492139826));
#21461=CARTESIAN_POINT('Ctrl Pts',(31.6331819033213,-33.9624301234347,7.0650057308514));
#21462=CARTESIAN_POINT('Ctrl Pts',(31.9723337540393,-32.8618836124063,7.01267235506732));
#21463=CARTESIAN_POINT('Ctrl Pts',(32.9030919679943,-31.943669301846,6.96033897928324));
#21464=CARTESIAN_POINT('Ctrl Pts',(34.0081264335795,-31.6194492096822,6.90800560349915));
#21465=CARTESIAN_POINT('Ctrl Pts',(35.1131608991647,-31.2952291175184,6.85567222771506));
#21466=CARTESIAN_POINT('Ctrl Pts',(36.3924716163801,-31.5650032437512,6.80333885193098));
#21467=CARTESIAN_POINT('Ctrl Pts',(37.2724835206594,-32.3078288702224,6.75100547614689));
#21468=CARTESIAN_POINT('Ctrl Pts',(38.1524954249387,-33.0506544966935,6.69867210036281));
#21469=CARTESIAN_POINT('Ctrl Pts',(38.6332085162819,-34.2665316234029,6.64633872457873));
#21470=CARTESIAN_POINT('Ctrl Pts',(38.4990877924354,-35.4103100458006,6.59400534879464));
#21471=CARTESIAN_POINT('Ctrl Pts',(38.3649670685888,-36.5540884681983,6.54167197301056));
#21472=CARTESIAN_POINT('Ctrl Pts',(37.6160125295525,-37.6257681862843,6.48933859722647));
#21473=CARTESIAN_POINT('Ctrl Pts',(36.5880240094475,-38.1448593691216,6.43700522144239));
#21474=CARTESIAN_POINT('Ctrl Pts',(35.5600354893424,-38.663950551959,6.3846718456583));
#21475=CARTESIAN_POINT('Ctrl Pts',(34.2530129881685,-38.6304531995479,6.33233846987422));
#21476=CARTESIAN_POINT('Ctrl Pts',(33.2529650852691,-38.0593845647942,6.28000509409014));
#21477=CARTESIAN_POINT('Ctrl Pts',(32.2529171823696,-37.4883159300405,6.22767171830605));
#21478=CARTESIAN_POINT('Ctrl Pts',(31.5598438777445,-36.3796760129444,6.17533834252196));
#21479=CARTESIAN_POINT('Ctrl Pts',(31.4844885221415,-35.230529556181,6.12300496673788));
#21480=CARTESIAN_POINT('Ctrl Pts',(31.4794864356562,-35.1542492451791,6.11953107865591));
#21481=CARTESIAN_POINT('Ctrl Pts',(31.4772062002897,-35.0777904501775,6.11605719057394));
#21482=CARTESIAN_POINT('Ctrl Pts',(31.4775766908735,-35.0013091813966,6.11258330249198));
#21483=CARTESIAN_POINT('Ctrl Pts',(33.9479286229388,-38.9352951690526,8.));
#21484=CARTESIAN_POINT('Ctrl Pts',(33.8318204065611,-38.8956804683211,8.));
#21485=CARTESIAN_POINT('Ctrl Pts',(33.7179772526967,-38.8505153756638,8.));
#21486=CARTESIAN_POINT('Ctrl Pts',(33.6066250571068,-38.8001574942087,8.));
#21487=CARTESIAN_POINT('Ctrl Pts',(33.4927757454994,-38.7486703178014,8.));
#21488=CARTESIAN_POINT('Ctrl Pts',(33.3815297429693,-38.6917543422691,8.));
#21489=CARTESIAN_POINT('Ctrl Pts',(33.2731527586738,-38.6297431972011,8.));
#21490=CARTESIAN_POINT('Ctrl Pts',(33.1592144063828,-38.5645499484809,8.));
#21491=CARTESIAN_POINT('Ctrl Pts',(33.0484461029789,-38.4937247712042,8.));
#21492=CARTESIAN_POINT('Ctrl Pts',(32.9411957572322,-38.4176091405434,8.));
#21493=CARTESIAN_POINT('Ctrl Pts',(32.8473517047039,-38.3510079637152,8.));
#21494=CARTESIAN_POINT('Ctrl Pts',(32.7562013929947,-38.2803552258207,8.));
#21495=CARTESIAN_POINT('Ctrl Pts',(32.668009391503,-38.2058575466902,8.));
#21496=CARTESIAN_POINT('Ctrl Pts',(32.6506323829748,-38.1911788141103,8.));
#21497=CARTESIAN_POINT('Ctrl Pts',(32.6333703275703,-38.1763507567444,8.));
#21498=CARTESIAN_POINT('Ctrl Pts',(32.6162254037543,-38.1613748841763,8.));
#21499=CARTESIAN_POINT('Ctrl Pts',(32.603691142847,-38.1504263669302,8.));
#21500=CARTESIAN_POINT('Ctrl Pts',(32.5912206997708,-38.139399841404,8.));
#21501=CARTESIAN_POINT('Ctrl Pts',(32.5788237219142,-38.1283040179759,8.));
#21502=CARTESIAN_POINT('Ctrl Pts',(32.4862445714949,-38.0454417334689,8.));
#21503=CARTESIAN_POINT('Ctrl Pts',(32.3976212761744,-37.9585977539474,8.));
#21504=CARTESIAN_POINT('Ctrl Pts',(32.3132152636303,-37.8680929905958,8.));
#21505=CARTESIAN_POINT('Ctrl Pts',(32.2290010683149,-37.7777939042141,8.));
#21506=CARTESIAN_POINT('Ctrl Pts',(32.1489844921721,-37.6838499490402,8.));
#21507=CARTESIAN_POINT('Ctrl Pts',(32.0734656135458,-37.5865478166696,8.));
#21508=CARTESIAN_POINT('Ctrl Pts',(31.9989790801238,-37.4905758071975,8.));
#21509=CARTESIAN_POINT('Ctrl Pts',(31.9288677181994,-37.3913361205739,8.));
#21510=CARTESIAN_POINT('Ctrl Pts',(31.8634655056288,-37.2890830233624,8.));
#21511=CARTESIAN_POINT('Ctrl Pts',(31.8101602412414,-37.2057429012617,8.));
#21512=CARTESIAN_POINT('Ctrl Pts',(31.7599839333137,-37.1204004861509,8.));
#21513=CARTESIAN_POINT('Ctrl Pts',(31.7131433458597,-37.0331876031136,8.));
#21514=CARTESIAN_POINT('Ctrl Pts',(31.7012416847729,-37.011027800414,8.));
#21515=CARTESIAN_POINT('Ctrl Pts',(31.6895555071392,-36.9887472225083,8.));
#21516=CARTESIAN_POINT('Ctrl Pts',(31.6780884679743,-36.9663480066189,8.));
#21517=CARTESIAN_POINT('Ctrl Pts',(31.6699335871488,-36.9504186168665,8.));
#21518=CARTESIAN_POINT('Ctrl Pts',(31.6618932487394,-36.9344364128785,8.));
#21519=CARTESIAN_POINT('Ctrl Pts',(31.6539711105215,-36.918407803011,8.));
#21520=CARTESIAN_POINT('Ctrl Pts',(31.6010103294039,-36.8112539418358,8.));
#21521=CARTESIAN_POINT('Ctrl Pts',(31.553288398372,-36.7019501913722,8.));
#21522=CARTESIAN_POINT('Ctrl Pts',(31.5110841176717,-36.5907591572156,8.));
#21523=CARTESIAN_POINT('Ctrl Pts',(31.4697159940302,-36.4817710552385,8.));
#21524=CARTESIAN_POINT('Ctrl Pts',(31.433648781936,-36.3709690780795,8.));
#21525=CARTESIAN_POINT('Ctrl Pts',(31.4031932495943,-36.2585867452464,8.));
#21526=CARTESIAN_POINT('Ctrl Pts',(31.3987391935523,-36.2421510709998,8.));
#21527=CARTESIAN_POINT('Ctrl Pts',(31.3944052523692,-36.2256815804349,8.));
#21528=CARTESIAN_POINT('Ctrl Pts',(31.3901924922002,-36.2091789909079,8.));
#21529=CARTESIAN_POINT('Ctrl Pts',(31.3605239499998,-36.0929588041061,8.));
#21530=CARTESIAN_POINT('Ctrl Pts',(31.3368613966103,-35.9750966537399,8.));
#21531=CARTESIAN_POINT('Ctrl Pts',(31.319113975657,-35.8560283881328,8.));
#21532=CARTESIAN_POINT('Ctrl Pts',(31.3091304483948,-35.7890484433355,8.));
#21533=CARTESIAN_POINT('Ctrl Pts',(31.3010196851544,-35.7216868798927,8.));
#21534=CARTESIAN_POINT('Ctrl Pts',(31.2947725609189,-35.6540227383851,8.));
#21535=CARTESIAN_POINT('Ctrl Pts',(31.2918900964785,-35.6228020559662,8.));
#21536=CARTESIAN_POINT('Ctrl Pts',(31.2894044622378,-35.591516977816,8.));
#21537=CARTESIAN_POINT('Ctrl Pts',(31.2873151093096,-35.5601754031315,8.));
#21538=CARTESIAN_POINT('Ctrl Pts',(31.2861140199798,-35.542158326923,8.));
#21539=CARTESIAN_POINT('Ctrl Pts',(31.2850444024964,-35.5241296340464,8.));
#21540=CARTESIAN_POINT('Ctrl Pts',(31.2841061875917,-35.5060991653233,8.));
#21541=CARTESIAN_POINT('Ctrl Pts',(31.2777952935748,-35.3848173815625,8.));
#21542=CARTESIAN_POINT('Ctrl Pts',(31.2774169324427,-35.2633382728991,8.));
#21543=CARTESIAN_POINT('Ctrl Pts',(31.2828128947659,-35.142109099441,8.));
#21544=CARTESIAN_POINT('Ctrl Pts',(31.2880969228261,-35.0233947134034,8.));
#21545=CARTESIAN_POINT('Ctrl Pts',(31.2989186932579,-34.9049190770275,8.));
#21546=CARTESIAN_POINT('Ctrl Pts',(31.3151830117592,-34.7871081783408,8.));
#21547=CARTESIAN_POINT('Ctrl Pts',(31.3312884180702,-34.67044836311,8.));
#21548=CARTESIAN_POINT('Ctrl Pts',(31.3527308881008,-34.5544395226326,8.));
#21549=CARTESIAN_POINT('Ctrl Pts',(31.3794647737014,-34.4395141802506,8.));
#21550=CARTESIAN_POINT('Ctrl Pts',(31.396871707047,-34.3646841385402,8.));
#21551=CARTESIAN_POINT('Ctrl Pts',(31.416522902222,-34.2903138655065,8.));
#21552=CARTESIAN_POINT('Ctrl Pts',(31.4384155592443,-34.2165296601315,8.));
#21553=CARTESIAN_POINT('Ctrl Pts',(31.4458038981696,-34.1916289495378,8.));
#21554=CARTESIAN_POINT('Ctrl Pts',(31.4534475860939,-34.1667950423673,8.));
#21555=CARTESIAN_POINT('Ctrl Pts',(31.461346703037,-34.1420329699976,8.));
#21556=CARTESIAN_POINT('Ctrl Pts',(31.46643308557,-34.1260882291753,8.));
#21557=CARTESIAN_POINT('Ctrl Pts',(31.471624585416,-34.1101758846519,8.));
#21558=CARTESIAN_POINT('Ctrl Pts',(31.476918343353,-34.0943053028287,8.));
#21559=CARTESIAN_POINT('Ctrl Pts',(31.513816049212,-33.9836867088362,8.));
#21560=CARTESIAN_POINT('Ctrl Pts',(31.5557144650388,-33.8749795921173,8.));
#21561=CARTESIAN_POINT('Ctrl Pts',(31.6025487964097,-33.7686031580514,8.));
#21562=CARTESIAN_POINT('Ctrl Pts',(31.6406629208299,-33.6820332311479,8.));
#21563=CARTESIAN_POINT('Ctrl Pts',(31.682046953583,-33.5970070600165,8.));
#21564=CARTESIAN_POINT('Ctrl Pts',(31.7266869557237,-33.5137662402706,8.));
#21565=CARTESIAN_POINT('Ctrl Pts',(31.7483019580961,-33.4734604510681,8.));
#21566=CARTESIAN_POINT('Ctrl Pts',(31.7706806142055,-33.4335734915742,8.));
#21567=CARTESIAN_POINT('Ctrl Pts',(31.7938228147784,-33.3941343150086,8.));
#21568=CARTESIAN_POINT('Ctrl Pts',(31.8074092885987,-33.3709801063925,8.));
#21569=CARTESIAN_POINT('Ctrl Pts',(31.8212609965416,-33.347977169053,8.));
#21570=CARTESIAN_POINT('Ctrl Pts',(31.8353638634359,-33.3251538546887,8.));
#21571=CARTESIAN_POINT('Ctrl Pts',(31.8937952976074,-33.2305915929272,8.));
#21572=CARTESIAN_POINT('Ctrl Pts',(31.9565779834776,-33.1390345522359,8.));
#21573=CARTESIAN_POINT('Ctrl Pts',(32.0236778740976,-33.0508734495428,8.));
#21574=CARTESIAN_POINT('Ctrl Pts',(32.0837087245751,-32.972000206609,8.));
#21575=CARTESIAN_POINT('Ctrl Pts',(32.1471956775548,-32.8958451124639,8.));
#21576=CARTESIAN_POINT('Ctrl Pts',(32.2141378419758,-32.8227144830143,8.));
#21577=CARTESIAN_POINT('Ctrl Pts',(32.2489927811285,-32.7846373807617,8.));
#21578=CARTESIAN_POINT('Ctrl Pts',(32.2847848221939,-32.7473806972021,8.));
#21579=CARTESIAN_POINT('Ctrl Pts',(32.3214765561793,-32.7109598296518,8.));
#21580=CARTESIAN_POINT('Origin',(0.,0.,8.));
#21581=CARTESIAN_POINT('',(-50.,50.,8.));
#21582=CARTESIAN_POINT('',(-50.,-50.,8.));
#21583=CARTESIAN_POINT('',(-50.,50.,8.));
#21584=CARTESIAN_POINT('',(50.,-50.,8.));
#21585=CARTESIAN_POINT('',(-50.,-50.,8.));
#21586=CARTESIAN_POINT('',(50.,50.,8.));
#21587=CARTESIAN_POINT('',(50.,-50.,8.));
#21588=CARTESIAN_POINT('',(50.,50.,8.));
#21589=CARTESIAN_POINT('Ctrl Pts',(-32.3264680662287,-32.7141668369925,
8.));
#21590=CARTESIAN_POINT('Ctrl Pts',(-32.2493255072635,-32.7912796001948,
8.));
#21591=CARTESIAN_POINT('Ctrl Pts',(-32.1762953075955,-32.8720145313034,
8.));
#21592=CARTESIAN_POINT('Ctrl Pts',(-32.1073697738656,-32.9559531279149,
8.));
#21593=CARTESIAN_POINT('Ctrl Pts',(-32.0366843378685,-33.0420349611253,
8.));
#21594=CARTESIAN_POINT('Ctrl Pts',(-31.9703154802321,-33.1314866020839,
8.));
#21595=CARTESIAN_POINT('Ctrl Pts',(-31.9082847764611,-33.2239028032894,
8.));
#21596=CARTESIAN_POINT('Ctrl Pts',(-31.8449630319238,-33.3182424565268,
8.));
#21597=CARTESIAN_POINT('Ctrl Pts',(-31.786161483907,-33.415671941835,8.));
#21598=CARTESIAN_POINT('Ctrl Pts',(-31.7319398749946,-33.5157996279616,
8.));
#21599=CARTESIAN_POINT('Ctrl Pts',(-31.6801506359753,-33.6114356072929,
8.));
#21600=CARTESIAN_POINT('Ctrl Pts',(-31.6325396515499,-33.709533968736,8.));
#21601=CARTESIAN_POINT('Ctrl Pts',(-31.5891944935205,-33.8097780642334,
8.));
#21602=CARTESIAN_POINT('Ctrl Pts',(-31.582156905406,-33.8260538534356,8.));
#21603=CARTESIAN_POINT('Ctrl Pts',(-31.5752318490596,-33.8423862467834,
8.));
#21604=CARTESIAN_POINT('Ctrl Pts',(-31.568419792889,-33.8587739316911,8.));
#21605=CARTESIAN_POINT('Ctrl Pts',(-31.5619098742369,-33.8744347678579,
8.));
#21606=CARTESIAN_POINT('Ctrl Pts',(-31.5555061718916,-33.8901389077819,
8.));
#21607=CARTESIAN_POINT('Ctrl Pts',(-31.5492108990198,-33.9058797005882,
8.));
#21608=CARTESIAN_POINT('Ctrl Pts',(-31.5058255436634,-34.0143610807278,
8.));
#21609=CARTESIAN_POINT('Ctrl Pts',(-31.4675540442795,-34.1246594478804,
8.));
#21610=CARTESIAN_POINT('Ctrl Pts',(-31.434425017105,-34.2363429975606,8.));
#21611=CARTESIAN_POINT('Ctrl Pts',(-31.4008614525105,-34.3494914463237,
8.));
#21612=CARTESIAN_POINT('Ctrl Pts',(-31.3725757523594,-34.4640624049253,
8.));
#21613=CARTESIAN_POINT('Ctrl Pts',(-31.3496403133382,-34.5796393782454,
8.));
#21614=CARTESIAN_POINT('Ctrl Pts',(-31.3256653487767,-34.7004547608028,
8.));
#21615=CARTESIAN_POINT('Ctrl Pts',(-31.307535844936,-34.8223702353544,8.));
#21616=CARTESIAN_POINT('Ctrl Pts',(-31.2953902232888,-34.9449334450722,
8.));
#21617=CARTESIAN_POINT('Ctrl Pts',(-31.2862810070535,-35.0368558523606,
8.));
#21618=CARTESIAN_POINT('Ctrl Pts',(-31.2805388477475,-35.1291432073786,
8.));
#21619=CARTESIAN_POINT('Ctrl Pts',(-31.2782452710195,-35.2216081255571,
8.));
#21620=CARTESIAN_POINT('Ctrl Pts',(-31.2776977000309,-35.243683300125,8.));
#21621=CARTESIAN_POINT('Ctrl Pts',(-31.2773468435284,-35.2657731220308,
8.));
#21622=CARTESIAN_POINT('Ctrl Pts',(-31.277193913283,-35.2878459781507,8.));
#21623=CARTESIAN_POINT('Ctrl Pts',(-31.2763590765867,-35.4083403266138,
8.));
#21624=CARTESIAN_POINT('Ctrl Pts',(-31.2814123990406,-35.5284798599375,
8.));
#21625=CARTESIAN_POINT('Ctrl Pts',(-31.2924228410947,-35.6478385426709,
8.));
#21626=CARTESIAN_POINT('Ctrl Pts',(-31.303362629127,-35.7664313005734,8.));
#21627=CARTESIAN_POINT('Ctrl Pts',(-31.3201830802735,-35.8842540736147,
8.));
#21628=CARTESIAN_POINT('Ctrl Pts',(-31.3430012709811,-36.000901820846,8.));
#21629=CARTESIAN_POINT('Ctrl Pts',(-31.3458749177941,-36.0155920489787,
8.));
#21630=CARTESIAN_POINT('Ctrl Pts',(-31.3488437566082,-36.0302636478795,
8.));
#21631=CARTESIAN_POINT('Ctrl Pts',(-31.3519080804568,-36.0449158122488,
8.));
#21632=CARTESIAN_POINT('Ctrl Pts',(-31.3758185581684,-36.1592445408324,
8.));
#21633=CARTESIAN_POINT('Ctrl Pts',(-31.4055382437248,-36.2723905489836,
8.));
#21634=CARTESIAN_POINT('Ctrl Pts',(-31.4407609915798,-36.3840873440382,
8.));
#21635=CARTESIAN_POINT('Ctrl Pts',(-31.4627262403709,-36.4537425538657,
8.));
#21636=CARTESIAN_POINT('Ctrl Pts',(-31.4868326485685,-36.5228340916482,
8.));
#21637=CARTESIAN_POINT('Ctrl Pts',(-31.5130158235422,-36.5912951432516,
8.));
#21638=CARTESIAN_POINT('Ctrl Pts',(-31.5219654331702,-36.6146956547323,
8.));
#21639=CARTESIAN_POINT('Ctrl Pts',(-31.5311577380477,-36.638022485054,8.));
#21640=CARTESIAN_POINT('Ctrl Pts',(-31.5405903538195,-36.6612728973655,
8.));
#21641=CARTESIAN_POINT('Ctrl Pts',(-31.5473394036631,-36.677908600056,8.));
#21642=CARTESIAN_POINT('Ctrl Pts',(-31.5542120267349,-36.6945063014083,
8.));
#21643=CARTESIAN_POINT('Ctrl Pts',(-31.5612002800447,-36.7110486972688,
8.));
#21644=CARTESIAN_POINT('Ctrl Pts',(-31.6071216062265,-36.8197523636167,
8.));
#21645=CARTESIAN_POINT('Ctrl Pts',(-31.6580959615467,-36.9262296326556,
8.));
#21646=CARTESIAN_POINT('Ctrl Pts',(-31.7137649062032,-37.0302261570189,
8.));
#21647=CARTESIAN_POINT('Ctrl Pts',(-31.7713490613653,-37.1378005332208,
8.));
#21648=CARTESIAN_POINT('Ctrl Pts',(-31.833956554581,-37.2427212245297,8.));
#21649=CARTESIAN_POINT('Ctrl Pts',(-31.9012460458509,-37.3446993846474,
8.));
#21650=CARTESIAN_POINT('Ctrl Pts',(-31.9691687068521,-37.4476371223012,
8.));
#21651=CARTESIAN_POINT('Ctrl Pts',(-32.0418623269422,-37.547577436253,8.));
#21652=CARTESIAN_POINT('Ctrl Pts',(-32.1190263529718,-37.6442049753141,
8.));
#21653=CARTESIAN_POINT('Ctrl Pts',(-32.1734394282079,-37.7123429642625,
8.));
#21654=CARTESIAN_POINT('Ctrl Pts',(-32.230076492864,-37.7788333069719,8.));
#21655=CARTESIAN_POINT('Ctrl Pts',(-32.288845213566,-37.8435569436544,8.));
#21656=CARTESIAN_POINT('Ctrl Pts',(-32.3150777918285,-37.8724476161826,
8.));
#21657=CARTESIAN_POINT('Ctrl Pts',(-32.3417352269367,-37.9009861713024,
8.));
#21658=CARTESIAN_POINT('Ctrl Pts',(-32.3688099173017,-37.9291614469859,
8.));
#21659=CARTESIAN_POINT('Ctrl Pts',(-32.3804320487223,-37.941256017686,8.));
#21660=CARTESIAN_POINT('Ctrl Pts',(-32.3921296471323,-37.9532821092146,
8.));
#21661=CARTESIAN_POINT('Ctrl Pts',(-32.4038956063136,-37.9652324558272,
8.));
#21662=CARTESIAN_POINT('Ctrl Pts',(-32.4923378704609,-38.0550607218847,
8.));
#21663=CARTESIAN_POINT('Ctrl Pts',(-32.5847394664431,-38.1407163588179,
8.));
#21664=CARTESIAN_POINT('Ctrl Pts',(-32.6807716550536,-38.2218812155311,
8.));
#21665=CARTESIAN_POINT('Ctrl Pts',(-32.7628115828128,-38.2912200390828,
8.));
#21666=CARTESIAN_POINT('Ctrl Pts',(-32.8475022057307,-38.3572813267927,
8.));
#21667=CARTESIAN_POINT('Ctrl Pts',(-32.9346627816287,-38.4198491494197,
8.));
#21668=CARTESIAN_POINT('Ctrl Pts',(-32.9737737137373,-38.447924753989,8.));
#21669=CARTESIAN_POINT('Ctrl Pts',(-33.0133822496832,-38.4752966907185,
8.));
#21670=CARTESIAN_POINT('Ctrl Pts',(-33.0534733017689,-38.5019440931387,
8.));
#21671=CARTESIAN_POINT('Ctrl Pts',(-33.0807070399686,-38.5200455981744,
8.));
#21672=CARTESIAN_POINT('Ctrl Pts',(-33.1081690766608,-38.5378161440549,
8.));
#21673=CARTESIAN_POINT('Ctrl Pts',(-33.1358247214715,-38.5552304161034,
8.));
#21674=CARTESIAN_POINT('Ctrl Pts',(-33.2426290354803,-38.6224832099845,
8.));
#21675=CARTESIAN_POINT('Ctrl Pts',(-33.3523800768607,-38.684469196206,8.));
#21676=CARTESIAN_POINT('Ctrl Pts',(-33.4647758690787,-38.7408547167133,
8.));
#21677=CARTESIAN_POINT('Ctrl Pts',(-33.5668696003918,-38.7920720093452,
8.));
#21678=CARTESIAN_POINT('Ctrl Pts',(-33.6711462627517,-38.8386684870918,
8.));
#21679=CARTESIAN_POINT('Ctrl Pts',(-33.777402890587,-38.880364981349,8.));
#21680=CARTESIAN_POINT('Ctrl Pts',(-33.8328334021929,-38.9021166410425,
8.));
#21681=CARTESIAN_POINT('Ctrl Pts',(-33.8888030678697,-38.9225343317631,
8.));
#21682=CARTESIAN_POINT('Ctrl Pts',(-33.9452677648582,-38.941630165528,8.));
#21683=CARTESIAN_POINT('Ctrl Pts',(-36.0520713770612,-38.9352951690526,
8.));
#21684=CARTESIAN_POINT('Ctrl Pts',(-36.1681793348248,-38.8956805565571,
8.));
#21685=CARTESIAN_POINT('Ctrl Pts',(-36.2820222319885,-38.8505155239877,
8.));
#21686=CARTESIAN_POINT('Ctrl Pts',(-36.39337417598,-38.8001576820793,8.));
#21687=CARTESIAN_POINT('Ctrl Pts',(-36.507223335641,-38.7486704984873,8.));
#21688=CARTESIAN_POINT('Ctrl Pts',(-36.6184691867386,-38.6917544842536,
8.));
#21689=CARTESIAN_POINT('Ctrl Pts',(-36.726846022942,-38.6297432779853,8.));
#21690=CARTESIAN_POINT('Ctrl Pts',(-36.8407844151035,-38.5645498530274,
8.));
#21691=CARTESIAN_POINT('Ctrl Pts',(-36.9515527511922,-38.4937244553102,
8.));
#21692=CARTESIAN_POINT('Ctrl Pts',(-37.0588031240991,-38.417608572184,8.));
#21693=CARTESIAN_POINT('Ctrl Pts',(-37.1526472003926,-38.3510071744486,
8.));
#21694=CARTESIAN_POINT('Ctrl Pts',(-37.2437975316357,-38.2803541911134,
8.));
#21695=CARTESIAN_POINT('Ctrl Pts',(-37.3319895495211,-38.2058562501456,
8.));
#21696=CARTESIAN_POINT('Ctrl Pts',(-37.3493652308069,-38.1911785898568,
8.));
#21697=CARTESIAN_POINT('Ctrl Pts',(-37.3666259764485,-38.1763516270108,
8.));
#21698=CARTESIAN_POINT('Ctrl Pts',(-37.3837696084918,-38.1613768709081,
8.));
#21699=CARTESIAN_POINT('Ctrl Pts',(-37.3963039208792,-38.1504283000079,
8.));
#21700=CARTESIAN_POINT('Ctrl Pts',(-37.4087744173897,-38.1394017179875,
8.));
#21701=CARTESIAN_POINT('Ctrl Pts',(-37.421171447845,-38.1283058376695,8.));
#21702=CARTESIAN_POINT('Ctrl Pts',(-37.5137506606012,-38.0454434240953,
8.));
#21703=CARTESIAN_POINT('Ctrl Pts',(-37.6023740233075,-37.9585993019841,
8.));
#21704=CARTESIAN_POINT('Ctrl Pts',(-37.686780110783,-37.8680943929378,8.));
#21705=CARTESIAN_POINT('Ctrl Pts',(-37.7709944562299,-37.7777950803761,
8.));
#21706=CARTESIAN_POINT('Ctrl Pts',(-37.8510111825053,-37.6838508893952,
8.));
#21707=CARTESIAN_POINT('Ctrl Pts',(-37.9265302130999,-37.5865485225552,
8.));
#21708=CARTESIAN_POINT('Ctrl Pts',(-38.0010169291866,-37.4905762395914,
8.));
#21709=CARTESIAN_POINT('Ctrl Pts',(-38.0711284717142,-37.3913362778857,
8.));
#21710=CARTESIAN_POINT('Ctrl Pts',(-38.1365308641829,-37.2890829148734,
8.));
#21711=CARTESIAN_POINT('Ctrl Pts',(-38.1898364642257,-37.2057422805937,
8.));
#21712=CARTESIAN_POINT('Ctrl Pts',(-38.2400130851628,-37.1203993452656,
8.));
#21713=CARTESIAN_POINT('Ctrl Pts',(-38.2868539614533,-37.0331859413737,
8.));
#21714=CARTESIAN_POINT('Ctrl Pts',(-38.2987540819478,-37.0110290114177,
8.));
#21715=CARTESIAN_POINT('Ctrl Pts',(-38.3104387758635,-36.9887513389692,
8.));
#21716=CARTESIAN_POINT('Ctrl Pts',(-38.3219043896502,-36.9663550605045,
8.));
#21717=CARTESIAN_POINT('Ctrl Pts',(-38.3300610648434,-36.9504222746659,
8.));
#21718=CARTESIAN_POINT('Ctrl Pts',(-38.3381031537755,-36.9344366433847,
8.));
#21719=CARTESIAN_POINT('Ctrl Pts',(-38.3460269902799,-36.918404590898,8.));
#21720=CARTESIAN_POINT('Ctrl Pts',(-38.3989878678949,-36.8112504908368,
8.));
#21721=CARTESIAN_POINT('Ctrl Pts',(-38.4467098948397,-36.7019465274356,
8.));
#21722=CARTESIAN_POINT('Ctrl Pts',(-38.4889142721076,-36.5907553164102,
8.));
#21723=CARTESIAN_POINT('Ctrl Pts',(-38.5302824920512,-36.4817670367281,
8.));
#21724=CARTESIAN_POINT('Ctrl Pts',(-38.566349800654,-36.3709649163585,8.));
#21725=CARTESIAN_POINT('Ctrl Pts',(-38.5968054307926,-36.2585824846173,
8.));
#21726=CARTESIAN_POINT('Ctrl Pts',(-38.6012596681997,-36.2421461794391,
8.));
#21727=CARTESIAN_POINT('Ctrl Pts',(-38.6055937817646,-36.225676056354,8.));
#21728=CARTESIAN_POINT('Ctrl Pts',(-38.6098067052154,-36.2091728328306,
8.));
#21729=CARTESIAN_POINT('Ctrl Pts',(-38.6394752606328,-36.0929526338671,
8.));
#21730=CARTESIAN_POINT('Ctrl Pts',(-38.6631378364378,-35.9750905238851,
8.));
#21731=CARTESIAN_POINT('Ctrl Pts',(-38.6808852873793,-35.8560223427045,
8.));
#21732=CARTESIAN_POINT('Ctrl Pts',(-38.6908688312617,-35.7890424470708,
8.));
#21733=CARTESIAN_POINT('Ctrl Pts',(-38.6989796136129,-35.7216809467524,
8.));
#21734=CARTESIAN_POINT('Ctrl Pts',(-38.705226759162,-35.6540168808315,8.));
#21735=CARTESIAN_POINT('Ctrl Pts',(-38.7081092384591,-35.6227961788899,
8.));
#21736=CARTESIAN_POINT('Ctrl Pts',(-38.7105948866426,-35.5915110836458,
8.));
#21737=CARTESIAN_POINT('Ctrl Pts',(-38.7126842525742,-35.5601694941906,
8.));
#21738=CARTESIAN_POINT('Ctrl Pts',(-38.713885344499,-35.542152482698,8.));
#21739=CARTESIAN_POINT('Ctrl Pts',(-38.7149549653242,-35.5241238555354,
8.));
#21740=CARTESIAN_POINT('Ctrl Pts',(-38.7158931843189,-35.5060934532667,
8.));
#21741=CARTESIAN_POINT('Ctrl Pts',(-38.7222041204107,-35.3848118366399,
8.));
#21742=CARTESIAN_POINT('Ctrl Pts',(-38.7225825299149,-35.2633329304591,
8.));
#21743=CARTESIAN_POINT('Ctrl Pts',(-38.717186620484,-35.142103985552,8.));
#21744=CARTESIAN_POINT('Ctrl Pts',(-38.7119026444224,-35.0233898278976,
8.));
#21745=CARTESIAN_POINT('Ctrl Pts',(-38.7010809307532,-34.9049144449008,
8.));
#21746=CARTESIAN_POINT('Ctrl Pts',(-38.684816672141,-34.7871038160559,8.));
#21747=CARTESIAN_POINT('Ctrl Pts',(-38.668711320133,-34.6704442318052,8.));
#21748=CARTESIAN_POINT('Ctrl Pts',(-38.6472689041617,-34.5544356388673,
8.));
#21749=CARTESIAN_POINT('Ctrl Pts',(-38.6205350708283,-34.439510552711,8.));
#21750=CARTESIAN_POINT('Ctrl Pts',(-38.6031281770284,-34.364680701536,8.));
#21751=CARTESIAN_POINT('Ctrl Pts',(-38.5834770220596,-34.2903106224296,
8.));
#21752=CARTESIAN_POINT('Ctrl Pts',(-38.5615844054563,-34.2165266120474,
8.));
#21753=CARTESIAN_POINT('Ctrl Pts',(-38.5541960539989,-34.1916258790507,
8.));
#21754=CARTESIAN_POINT('Ctrl Pts',(-38.5465523517576,-34.1667919500715,
8.));
#21755=CARTESIAN_POINT('Ctrl Pts',(-38.5386532186941,-34.1420298564502,
8.));
#21756=CARTESIAN_POINT('Ctrl Pts',(-38.5335668050111,-34.1260850368347,
8.));
#21757=CARTESIAN_POINT('Ctrl Pts',(-38.5283752724802,-34.1101726142316,
8.));
#21758=CARTESIAN_POINT('Ctrl Pts',(-38.5230814802764,-34.094301954882,8.));
#21759=CARTESIAN_POINT('Ctrl Pts',(-38.4861838094094,-33.9836836414723,
8.));
#21760=CARTESIAN_POINT('Ctrl Pts',(-38.4442854263901,-33.8749768051962,
8.));
#21761=CARTESIAN_POINT('Ctrl Pts',(-38.3974511240065,-33.7686006435033,
8.));
#21762=CARTESIAN_POINT('Ctrl Pts',(-38.3593370554135,-33.6820310114798,
8.));
#21763=CARTESIAN_POINT('Ctrl Pts',(-38.3179530814865,-33.5970051272784,
8.));
#21764=CARTESIAN_POINT('Ctrl Pts',(-38.2733131402326,-33.5137645815446,
8.));
#21765=CARTESIAN_POINT('Ctrl Pts',(-38.2516981548861,-33.4734589017939,
8.));
#21766=CARTESIAN_POINT('Ctrl Pts',(-38.2293195154062,-33.4335720492035,
8.));
#21767=CARTESIAN_POINT('Ctrl Pts',(-38.2061773309613,-33.3941329764629,
8.));
#21768=CARTESIAN_POINT('Ctrl Pts',(-38.1925909485316,-33.3709789684133,
8.));
#21769=CARTESIAN_POINT('Ctrl Pts',(-38.1787393350554,-33.3479762288434,
8.));
#21770=CARTESIAN_POINT('Ctrl Pts',(-38.1646365654847,-33.3251531088758,
8.));
#21771=CARTESIAN_POINT('Ctrl Pts',(-38.1062051167558,-33.2305909764135,
8.));
#21772=CARTESIAN_POINT('Ctrl Pts',(-38.0434224031259,-33.139034050394,8.));
#21773=CARTESIAN_POINT('Ctrl Pts',(-37.9763224701899,-33.050873041493,8.));
#21774=CARTESIAN_POINT('Ctrl Pts',(-37.9162917251371,-32.972000070726,8.));
#21775=CARTESIAN_POINT('Ctrl Pts',(-37.8528048824192,-32.8958452190746,
8.));
#21776=CARTESIAN_POINT('Ctrl Pts',(-37.7858628320068,-32.8227147956203,
8.));
#21777=CARTESIAN_POINT('Ctrl Pts',(-37.7510079037,-32.7846377476237,8.));
#21778=CARTESIAN_POINT('Ctrl Pts',(-37.7152158718889,-32.7473811107005,
8.));
#21779=CARTESIAN_POINT('Ctrl Pts',(-37.6785241456451,-32.7109602826758,
8.));
#21780=CARTESIAN_POINT('Ctrl Pts',(-32.3264680662287,37.2858331630075,8.));
#21781=CARTESIAN_POINT('Ctrl Pts',(-32.2493254281347,37.208720320707,8.));
#21782=CARTESIAN_POINT('Ctrl Pts',(-32.1762951458997,37.1279853156793,8.));
#21783=CARTESIAN_POINT('Ctrl Pts',(-32.1073695284417,37.0440466492215,8.));
#21784=CARTESIAN_POINT('Ctrl Pts',(-32.036684016981,36.9579647570495,8.));
#21785=CARTESIAN_POINT('Ctrl Pts',(-31.9703150813857,36.8685130624034,8.));
#21786=CARTESIAN_POINT('Ctrl Pts',(-31.9082842995806,36.7760968113946,8.));
#21787=CARTESIAN_POINT('Ctrl Pts',(-31.8449624922372,36.6817571324243,8.));
#21788=CARTESIAN_POINT('Ctrl Pts',(-31.7861608789268,36.5843276270745,8.));
#21789=CARTESIAN_POINT('Ctrl Pts',(-31.7319392047808,36.4841999248104,8.));
#21790=CARTESIAN_POINT('Ctrl Pts',(-31.680149951798,36.3885640193387,8.));
#21791=CARTESIAN_POINT('Ctrl Pts',(-31.6325389456654,36.2904657399127,8.));
#21792=CARTESIAN_POINT('Ctrl Pts',(-31.5891937601898,36.1902217321721,8.));
#21793=CARTESIAN_POINT('Ctrl Pts',(-31.5821558034642,36.1739451150407,8.));
#21794=CARTESIAN_POINT('Ctrl Pts',(-31.575230390001,36.1576118880571,8.));
#21795=CARTESIAN_POINT('Ctrl Pts',(-31.56841798829,36.1412233640005,8.));
#21796=CARTESIAN_POINT('Ctrl Pts',(-31.5619084669515,36.125563476111,8.));
#21797=CARTESIAN_POINT('Ctrl Pts',(-31.5555051500235,36.1098602922108,8.));
#21798=CARTESIAN_POINT('Ctrl Pts',(-31.5492102490141,36.0941204589327,8.));
#21799=CARTESIAN_POINT('Ctrl Pts',(-31.5058248130015,35.9856390819387,8.));
#21800=CARTESIAN_POINT('Ctrl Pts',(-31.467553236408,35.8753407193868,8.));
#21801=CARTESIAN_POINT('Ctrl Pts',(-31.4344241380457,35.7636571739254,8.));
#21802=CARTESIAN_POINT('Ctrl Pts',(-31.4008605131946,35.650508769435,8.));
#21803=CARTESIAN_POINT('Ctrl Pts',(-31.3725747552338,35.5359378557202,8.));
#21804=CARTESIAN_POINT('Ctrl Pts',(-31.3496392634799,35.4203609255757,8.));
#21805=CARTESIAN_POINT('Ctrl Pts',(-31.3256642608852,35.2995456742689,8.));
#21806=CARTESIAN_POINT('Ctrl Pts',(-31.3075347162269,35.1776303306686,8.));
#21807=CARTESIAN_POINT('Ctrl Pts',(-31.2953890537165,35.0550672480091,8.));
#21808=CARTESIAN_POINT('Ctrl Pts',(-31.2862798068337,34.9631449360145,8.));
#21809=CARTESIAN_POINT('Ctrl Pts',(-31.2805376168519,34.8708576741034,8.));
#21810=CARTESIAN_POINT('Ctrl Pts',(-31.2782440105566,34.778392845323,8.));
#21811=CARTESIAN_POINT('Ctrl Pts',(-31.2776964353943,34.7563178084142,8.));
#21812=CARTESIAN_POINT('Ctrl Pts',(-31.2773455727076,34.7342281241833,8.));
#21813=CARTESIAN_POINT('Ctrl Pts',(-31.2771926342729,34.7121554053342,8.));
#21814=CARTESIAN_POINT('Ctrl Pts',(-31.2763577480363,34.5916611083402,8.));
#21815=CARTESIAN_POINT('Ctrl Pts',(-31.2814110294711,34.4715216187175,8.));
#21816=CARTESIAN_POINT('Ctrl Pts',(-31.2924214415633,34.3521629693739,8.));
#21817=CARTESIAN_POINT('Ctrl Pts',(-31.3033611959409,34.2335702867641,8.));
#21818=CARTESIAN_POINT('Ctrl Pts',(-31.3201816201703,34.115747578293,8.));
#21819=CARTESIAN_POINT('Ctrl Pts',(-31.3429997930851,33.999099881963,8.));
#21820=CARTESIAN_POINT('Ctrl Pts',(-31.345873443513,33.984409630306,8.));
#21821=CARTESIAN_POINT('Ctrl Pts',(-31.3488422864746,33.96973800774,8.));
#21822=CARTESIAN_POINT('Ctrl Pts',(-31.35190661501,33.9550858195635,8.));
#21823=CARTESIAN_POINT('Ctrl Pts',(-31.3758170782861,33.8407571491025,8.));
#21824=CARTESIAN_POINT('Ctrl Pts',(-31.4055367574321,33.7276111853924,8.));
#21825=CARTESIAN_POINT('Ctrl Pts',(-31.4407595052535,33.6159144227599,8.));
#21826=CARTESIAN_POINT('Ctrl Pts',(-31.4627247636627,33.5462592025841,8.));
#21827=CARTESIAN_POINT('Ctrl Pts',(-31.4868311858377,33.4771676502711,8.));
#21828=CARTESIAN_POINT('Ctrl Pts',(-31.5130143786684,33.4087065804238,8.));
#21829=CARTESIAN_POINT('Ctrl Pts',(-31.5219642258836,33.3853054574484,8.));
#21830=CARTESIAN_POINT('Ctrl Pts',(-31.5311567813561,33.3619780190094,8.));
#21831=CARTESIAN_POINT('Ctrl Pts',(-31.5405896605283,33.3387270021894,8.));
#21832=CARTESIAN_POINT('Ctrl Pts',(-31.5473384631411,33.3220919409105,8.));
#21833=CARTESIAN_POINT('Ctrl Pts',(-31.5542108294608,33.3054948782145,8.));
#21834=CARTESIAN_POINT('Ctrl Pts',(-31.5611988172515,33.288953116597,8.));
#21835=CARTESIAN_POINT('Ctrl Pts',(-31.6071201467481,33.1802494799514,8.));
#21836=CARTESIAN_POINT('Ctrl Pts',(-31.6580945083799,33.0737722290612,8.));
#21837=CARTESIAN_POINT('Ctrl Pts',(-31.7137634608477,32.9697757128959,8.));
#21838=CARTESIAN_POINT('Ctrl Pts',(-31.7713476440883,32.8622013078145,8.));
#21839=CARTESIAN_POINT('Ctrl Pts',(-31.8339551704749,32.7572805788209,8.));
#21840=CARTESIAN_POINT('Ctrl Pts',(-31.9012446980031,32.6553023741411,8.));
#21841=CARTESIAN_POINT('Ctrl Pts',(-31.9691674082359,32.552364572362,8.));
#21842=CARTESIAN_POINT('Ctrl Pts',(-32.0418610824791,32.4524241883893,8.));
#21843=CARTESIAN_POINT('Ctrl Pts',(-32.1190251653974,32.3557965754622,8.));
#21844=CARTESIAN_POINT('Ctrl Pts',(-32.1734382985285,32.2876585121627,8.));
#21845=CARTESIAN_POINT('Ctrl Pts',(-32.2300754238941,32.2211680942644,8.));
#21846=CARTESIAN_POINT('Ctrl Pts',(-32.2888442072745,32.1564443823762,8.));
#21847=CARTESIAN_POINT('Ctrl Pts',(-32.3150764518969,32.1275540745384,8.));
#21848=CARTESIAN_POINT('Ctrl Pts',(-32.341733542045,32.0990158743987,8.));
#21849=CARTESIAN_POINT('Ctrl Pts',(-32.3688078763672,32.0708409435943,8.));
#21850=CARTESIAN_POINT('Ctrl Pts',(-32.3804297629888,32.0587466166393,8.));
#21851=CARTESIAN_POINT('Ctrl Pts',(-32.3921271141324,32.0467207651166,8.));
#21852=CARTESIAN_POINT('Ctrl Pts',(-32.4038928229971,32.0347706553995,8.));
#21853=CARTESIAN_POINT('Ctrl Pts',(-32.4923350889694,31.9449422571145,8.));
#21854=CARTESIAN_POINT('Ctrl Pts',(-32.5847366887113,31.8592864840437,8.));
#21855=CARTESIAN_POINT('Ctrl Pts',(-32.6807688805232,31.7781214891551,8.));
#21856=CARTESIAN_POINT('Ctrl Pts',(-32.7628090255767,31.7087823662183,8.));
#21857=CARTESIAN_POINT('Ctrl Pts',(-32.8474998792406,31.6427207947673,8.));
#21858=CARTESIAN_POINT('Ctrl Pts',(-32.9346606964287,31.5801527068548,8.));
#21859=CARTESIAN_POINT('Ctrl Pts',(-32.9737718119822,31.5520769292834,8.));
#21860=CARTESIAN_POINT('Ctrl Pts',(-33.0133805354119,31.5247048259746,8.));
#21861=CARTESIAN_POINT('Ctrl Pts',(-33.0534717786847,31.4980572637843,8.));
#21862=CARTESIAN_POINT('Ctrl Pts',(-33.0807061080661,31.4799553435978,8.));
#21863=CARTESIAN_POINT('Ctrl Pts',(-33.1081687455454,31.4621843968183,8.));
#21864=CARTESIAN_POINT('Ctrl Pts',(-33.1358249991596,31.4447697393726,8.));
#21865=CARTESIAN_POINT('Ctrl Pts',(-33.2426293820058,31.3775168942506,8.));
#21866=CARTESIAN_POINT('Ctrl Pts',(-33.3523804860194,31.3155308622806,8.));
#21867=CARTESIAN_POINT('Ctrl Pts',(-33.464776332519,31.2591453036981,8.));
#21868=CARTESIAN_POINT('Ctrl Pts',(-33.5668700198747,31.2079280232686,8.));
#21869=CARTESIAN_POINT('Ctrl Pts',(-33.671146627403,31.161331555616,8.));
#21870=CARTESIAN_POINT('Ctrl Pts',(-33.7774031884393,31.1196350702262,8.));
#21871=CARTESIAN_POINT('Ctrl Pts',(-33.8328337169093,31.0978833948665,8.));
#21872=CARTESIAN_POINT('Ctrl Pts',(-33.8888033971972,31.0774656906331,8.));
#21873=CARTESIAN_POINT('Ctrl Pts',(-33.9452681066883,31.058369845356,8.));
#21874=CARTESIAN_POINT('Ctrl Pts',(-36.0520713770612,31.0647048309474,8.));
#21875=CARTESIAN_POINT('Ctrl Pts',(-36.168179415234,31.1043194708775,8.));
#21876=CARTESIAN_POINT('Ctrl Pts',(-36.2820223922111,31.1494845221288,8.));
#21877=CARTESIAN_POINT('Ctrl Pts',(-36.3933744144291,31.1998423763314,8.));
#21878=CARTESIAN_POINT('Ctrl Pts',(-36.5072236213378,31.25132955769,8.));
#21879=CARTESIAN_POINT('Ctrl Pts',(-36.6184695195224,31.3082455598905,8.));
#21880=CARTESIAN_POINT('Ctrl Pts',(-36.7268464017735,31.3702567471293,8.));
#21881=CARTESIAN_POINT('Ctrl Pts',(-36.8407847815347,31.4354501172862,8.));
#21882=CARTESIAN_POINT('Ctrl Pts',(-36.9515531074568,31.5062754464572,8.));
#21883=CARTESIAN_POINT('Ctrl Pts',(-37.0588034719145,31.5823912510781,8.));
#21884=CARTESIAN_POINT('Ctrl Pts',(-37.152647540815,31.6489925801213,8.));
#21885=CARTESIAN_POINT('Ctrl Pts',(-37.2437978659804,31.7196454871349,8.));
#21886=CARTESIAN_POINT('Ctrl Pts',(-37.3319898787643,31.7941433466814,8.));
#21887=CARTESIAN_POINT('Ctrl Pts',(-37.3493659727369,31.8088213403836,8.));
#21888=CARTESIAN_POINT('Ctrl Pts',(-37.3666271256303,31.8236486435546,8.));
#21889=CARTESIAN_POINT('Ctrl Pts',(-37.3837711593319,31.8386237468057,8.));
#21890=CARTESIAN_POINT('Ctrl Pts',(-37.3963054555396,31.8495723008716,8.));
#21891=CARTESIAN_POINT('Ctrl Pts',(-37.4087759352647,31.8605988651726,8.));
#21892=CARTESIAN_POINT('Ctrl Pts',(-37.4211729491963,31.8716947276461,8.));
#21893=CARTESIAN_POINT('Ctrl Pts',(-37.5137521425834,31.9545571010691,8.));
#21894=CARTESIAN_POINT('Ctrl Pts',(-37.6023754843508,32.0414011788236,8.));
#21895=CARTESIAN_POINT('Ctrl Pts',(-37.6867815485414,32.1319060425465,8.));
#21896=CARTESIAN_POINT('Ctrl Pts',(-37.7709958473242,32.2222052847627,8.));
#21897=CARTESIAN_POINT('Ctrl Pts',(-37.8510125269352,32.3161494024035,8.));
#21898=CARTESIAN_POINT('Ctrl Pts',(-37.9265315102947,32.413451696318,8.));
#21899=CARTESIAN_POINT('Ctrl Pts',(-38.0010181696068,32.5094238942302,8.));
#21900=CARTESIAN_POINT('Ctrl Pts',(-38.0711296560004,32.6086637703888,8.));
#21901=CARTESIAN_POINT('Ctrl Pts',(-38.1365319925539,32.7109170507384,8.));
#21902=CARTESIAN_POINT('Ctrl Pts',(-38.189837488265,32.7942575257788,8.));
#21903=CARTESIAN_POINT('Ctrl Pts',(-38.2400140119095,32.8796002993686,8.));
#21904=CARTESIAN_POINT('Ctrl Pts',(-38.2868547984211,32.966813541324,8.));
#21905=CARTESIAN_POINT('Ctrl Pts',(-38.2987553976748,32.9889713640128,8.));
#21906=CARTESIAN_POINT('Ctrl Pts',(-38.3104405526761,33.0112499393599,8.));
#21907=CARTESIAN_POINT('Ctrl Pts',(-38.3219066094193,33.0336471306571,8.));
#21908=CARTESIAN_POINT('Ctrl Pts',(-38.3300627268695,33.0495788608817,8.));
#21909=CARTESIAN_POINT('Ctrl Pts',(-38.3381042716881,33.0655634268488,8.));
#21910=CARTESIAN_POINT('Ctrl Pts',(-38.3460275803167,33.0815944092568,8.));
#21911=CARTESIAN_POINT('Ctrl Pts',(-38.3989884279579,33.1887484350122,8.));
#21912=CARTESIAN_POINT('Ctrl Pts',(-38.4467104251109,33.2980523321741,8.));
#21913=CARTESIAN_POINT('Ctrl Pts',(-38.4889147723839,33.409243488173,8.));
#21914=CARTESIAN_POINT('Ctrl Pts',(-38.5302829624144,33.5182317125689,8.));
#21915=CARTESIAN_POINT('Ctrl Pts',(-38.5663502410402,33.6290337883757,8.));
#21916=CARTESIAN_POINT('Ctrl Pts',(-38.596805840802,33.7414161893267,8.));
#21917=CARTESIAN_POINT('Ctrl Pts',(-38.6012600218942,33.7578522985917,8.));
#21918=CARTESIAN_POINT('Ctrl Pts',(-38.6055940819337,33.7743222252706,8.));
#21919=CARTESIAN_POINT('Ctrl Pts',(-38.6098069546845,33.7908252519299,8.));
#21920=CARTESIAN_POINT('Ctrl Pts',(-38.6394755059943,33.9070454470715,8.));
#21921=CARTESIAN_POINT('Ctrl Pts',(-38.6631380748325,34.0249075695662,8.));
#21922=CARTESIAN_POINT('Ctrl Pts',(-38.6808855164532,34.1439757769513,8.));
#21923=CARTESIAN_POINT('Ctrl Pts',(-38.6908690551697,34.2109556878445,8.));
#21924=CARTESIAN_POINT('Ctrl Pts',(-38.6989798315808,34.2783172077624,8.));
#21925=CARTESIAN_POINT('Ctrl Pts',(-38.7052269705051,34.3459812971573,8.));
#21926=CARTESIAN_POINT('Ctrl Pts',(-38.7081094451816,34.3772019929916,8.));
#21927=CARTESIAN_POINT('Ctrl Pts',(-38.7105950890294,34.4084870828833,8.));
#21928=CARTESIAN_POINT('Ctrl Pts',(-38.712684450918,34.4398286677084,8.));
#21929=CARTESIAN_POINT('Ctrl Pts',(-38.7138855420385,34.457845699339,8.));
#21930=CARTESIAN_POINT('Ctrl Pts',(-38.7149551618269,34.47587434695,8.));
#21931=CARTESIAN_POINT('Ctrl Pts',(-38.7158933795518,34.4939047698972,8.));
#21932=CARTESIAN_POINT('Ctrl Pts',(-38.722204302566,34.6151864384397,8.));
#21933=CARTESIAN_POINT('Ctrl Pts',(-38.7225826970351,34.7366654075262,8.));
#21934=CARTESIAN_POINT('Ctrl Pts',(-38.7171867711641,34.8578944234449,8.));
#21935=CARTESIAN_POINT('Ctrl Pts',(-38.7119027789398,34.9766086520668,8.));
#21936=CARTESIAN_POINT('Ctrl Pts',(-38.7010810476264,35.0950841138035,8.));
#21937=CARTESIAN_POINT('Ctrl Pts',(-38.6848167703974,35.2128948265086,8.));
#21938=CARTESIAN_POINT('Ctrl Pts',(-38.6687114015083,35.3295544825446,8.));
#21939=CARTESIAN_POINT('Ctrl Pts',(-38.6472689687305,35.445563152418,8.));
#21940=CARTESIAN_POINT('Ctrl Pts',(-38.6205351191465,35.5604883182129,8.));
#21941=CARTESIAN_POINT('Ctrl Pts',(-38.603128213054,35.6353182285994,8.));
#21942=CARTESIAN_POINT('Ctrl Pts',(-38.5834770455875,35.7096883679731,8.));
#21943=CARTESIAN_POINT('Ctrl Pts',(-38.5615844164204,35.7834724389555,8.));
#21944=CARTESIAN_POINT('Ctrl Pts',(-38.5541960688544,35.8083731649983,8.));
#21945=CARTESIAN_POINT('Ctrl Pts',(-38.546552371059,35.8332070872086,8.));
#21946=CARTESIAN_POINT('Ctrl Pts',(-38.5386532430018,35.8579691742342,8.));
#21947=CARTESIAN_POINT('Ctrl Pts',(-38.533566838996,35.8739139693719,8.));
#21948=CARTESIAN_POINT('Ctrl Pts',(-38.5283753166192,35.8898263677189,8.));
#21949=CARTESIAN_POINT('Ctrl Pts',(-38.5230815350611,35.9056970029845,8.));
#21950=CARTESIAN_POINT('Ctrl Pts',(-38.4861838533105,36.0163154036073,8.));
#21951=CARTESIAN_POINT('Ctrl Pts',(-38.4442854600859,36.1250223270562,8.));
#21952=CARTESIAN_POINT('Ctrl Pts',(-38.3974511486834,36.2313985734173,8.));
#21953=CARTESIAN_POINT('Ctrl Pts',(-38.3593370627389,36.3179682970844,8.));
#21954=CARTESIAN_POINT('Ctrl Pts',(-38.3179530705292,36.4029942704614,8.));
#21955=CARTESIAN_POINT('Ctrl Pts',(-38.2733131103528,36.4862349013589,8.));
#21956=CARTESIAN_POINT('Ctrl Pts',(-38.2516981197193,36.52654061512,8.));
#21957=CARTESIAN_POINT('Ctrl Pts',(-38.2293194750761,36.5664275009295,8.));
#21958=CARTESIAN_POINT('Ctrl Pts',(-38.2061772856241,36.6058666059334,8.));
#21959=CARTESIAN_POINT('Ctrl Pts',(-38.1925908747914,36.6290206763194,8.));
#21960=CARTESIAN_POINT('Ctrl Pts',(-38.1787392319563,36.6520234773565,8.));
#21961=CARTESIAN_POINT('Ctrl Pts',(-38.1646364321387,36.6748466577435,8.));
#21962=CARTESIAN_POINT('Ctrl Pts',(-38.1062049879234,36.7694088304221,8.));
#21963=CARTESIAN_POINT('Ctrl Pts',(-38.0434222829092,36.8609657921147,8.));
#21964=CARTESIAN_POINT('Ctrl Pts',(-37.9763223631119,36.9491268302023,8.));
#21965=CARTESIAN_POINT('Ctrl Pts',(-37.9162915853069,37.0279998855573,8.));
#21966=CARTESIAN_POINT('Ctrl Pts',(-37.8528047083354,37.1041548125789,8.));
#21967=CARTESIAN_POINT('Ctrl Pts',(-37.7858626225071,37.1772853000647,8.));
#21968=CARTESIAN_POINT('Ctrl Pts',(-37.7510076908282,37.2153623649398,8.));
#21969=CARTESIAN_POINT('Ctrl Pts',(-37.7152156561398,37.2526190163742,8.));
#21970=CARTESIAN_POINT('Ctrl Pts',(-37.6785239274887,37.2890398567007,8.));
#21971=CARTESIAN_POINT('Ctrl Pts',(37.6735319337713,37.2858331630076,8.));
#21972=CARTESIAN_POINT('Ctrl Pts',(37.7506743707736,37.2087205217211,8.));
#21973=CARTESIAN_POINT('Ctrl Pts',(37.8237044431802,37.1279857045437,8.));
#21974=CARTESIAN_POINT('Ctrl Pts',(37.8926298478593,37.044047215584,8.));
#21975=CARTESIAN_POINT('Ctrl Pts',(37.9633151675467,36.957965473245,8.));
#21976=CARTESIAN_POINT('Ctrl Pts',(38.0296839050274,36.8685139150261,8.));
#21977=CARTESIAN_POINT('Ctrl Pts',(38.0917144885261,36.7760977905708,8.));
#21978=CARTESIAN_POINT('Ctrl Pts',(38.1550361362519,36.681758176998,8.));
#21979=CARTESIAN_POINT('Ctrl Pts',(38.213837583624,36.5843287225808,8.));
#21980=CARTESIAN_POINT('Ctrl Pts',(38.2680590919843,36.4842010613249,8.));
#21981=CARTESIAN_POINT('Ctrl Pts',(38.3198483094818,36.3885649681376,8.));
#21982=CARTESIAN_POINT('Ctrl Pts',(38.367459260449,36.2904664802624,8.));
#21983=CARTESIAN_POINT('Ctrl Pts',(38.4108043761726,36.1902222494829,8.));
#21984=CARTESIAN_POINT('Ctrl Pts',(38.4178413961439,36.1739477363751,8.));
#21985=CARTESIAN_POINT('Ctrl Pts',(38.4247659020623,36.1576166279166,8.));
#21986=CARTESIAN_POINT('Ctrl Pts',(38.4315774256463,36.1412302363951,8.));
#21987=CARTESIAN_POINT('Ctrl Pts',(38.4380879567714,36.1255679384209,8.));
#21988=CARTESIAN_POINT('Ctrl Pts',(38.444492253249,36.1098623247479,8.));
#21989=CARTESIAN_POINT('Ctrl Pts',(38.4507880993566,36.0941200527897,8.));
#21990=CARTESIAN_POINT('Ctrl Pts',(38.4941733303702,35.9856386677758,8.));
#21991=CARTESIAN_POINT('Ctrl Pts',(38.5324447107219,35.8753402935035,8.));
#21992=CARTESIAN_POINT('Ctrl Pts',(38.5655736281431,35.7636567372894,8.));
#21993=CARTESIAN_POINT('Ctrl Pts',(38.5991370998293,35.6505082202659,8.));
#21994=CARTESIAN_POINT('Ctrl Pts',(38.6274227108421,35.5359371924552,8.));
#21995=CARTESIAN_POINT('Ctrl Pts',(38.6503580685478,35.4203601525596,8.));
#21996=CARTESIAN_POINT('Ctrl Pts',(38.6743329744418,35.2995445677074,8.));
#21997=CARTESIAN_POINT('Ctrl Pts',(38.6924624153241,35.1776288913195,8.));
#21998=CARTESIAN_POINT('Ctrl Pts',(38.7046079739425,35.0550654857614,8.));
#21999=CARTESIAN_POINT('Ctrl Pts',(38.7137171429063,34.9631429315928,8.));
#22000=CARTESIAN_POINT('Ctrl Pts',(38.7194592548969,34.8708554330634,8.));
#22001=CARTESIAN_POINT('Ctrl Pts',(38.7217527860176,34.7783903770868,8.));
#22002=CARTESIAN_POINT('Ctrl Pts',(38.7223003505608,34.7563149905001,8.));
#22003=CARTESIAN_POINT('Ctrl Pts',(38.7226511975219,34.7342249565511,8.));
#22004=CARTESIAN_POINT('Ctrl Pts',(38.7228041151383,34.7121518890107,8.));
#22005=CARTESIAN_POINT('Ctrl Pts',(38.7236388754478,34.5916574611757,8.));
#22006=CARTESIAN_POINT('Ctrl Pts',(38.7185854897377,34.4715178604479,8.));
#22007=CARTESIAN_POINT('Ctrl Pts',(38.7075750014661,34.3521591261975,8.));
#22008=CARTESIAN_POINT('Ctrl Pts',(38.6966351615249,34.2335662521979,8.));
#22009=CARTESIAN_POINT('Ctrl Pts',(38.6798146688512,34.1157433795803,8.));
#22010=CARTESIAN_POINT('Ctrl Pts',(38.6569964506754,33.9990955538343,8.));
#22011=CARTESIAN_POINT('Ctrl Pts',(38.6541228094095,33.9844053618549,8.));
#22012=CARTESIAN_POINT('Ctrl Pts',(38.6511539769623,33.9697337993248,8.));
#22013=CARTESIAN_POINT('Ctrl Pts',(38.6480896603102,33.9550816715453,8.));
#22014=CARTESIAN_POINT('Ctrl Pts',(38.6241791602958,33.840752853322,8.));
#22015=CARTESIAN_POINT('Ctrl Pts',(38.5944594648021,33.7276067766126,8.));
#22016=CARTESIAN_POINT('Ctrl Pts',(38.5592367168361,33.6159099315205,8.));
#22017=CARTESIAN_POINT('Ctrl Pts',(38.5372714828272,33.5462547375853,8.));
#22018=CARTESIAN_POINT('Ctrl Pts',(38.5131650961288,33.4771632221397,8.));
#22019=CARTESIAN_POINT('Ctrl Pts',(38.4869819486326,33.4087021985955,8.));
#22020=CARTESIAN_POINT('Ctrl Pts',(38.4780327050517,33.385302629251,8.));
#22021=CARTESIAN_POINT('Ctrl Pts',(38.4688407862625,33.3619767358619,8.));
#22022=CARTESIAN_POINT('Ctrl Pts',(38.4594085763077,33.3387272549231,8.));
#22023=CARTESIAN_POINT('Ctrl Pts',(38.4526591454727,33.3220905638083,8.));
#22024=CARTESIAN_POINT('Ctrl Pts',(38.4457861267366,33.3054918782784,8.));
#22025=CARTESIAN_POINT('Ctrl Pts',(38.438797464252,33.2889485050412,8.));
#22026=CARTESIAN_POINT('Ctrl Pts',(38.3928761431039,33.180244792853,8.));
#22027=CARTESIAN_POINT('Ctrl Pts',(38.3419017974374,33.073767495779,8.));
#22028=CARTESIAN_POINT('Ctrl Pts',(38.2862328647479,32.9697709587171,8.));
#22029=CARTESIAN_POINT('Ctrl Pts',(38.2286487527766,32.8621966269402,8.));
#22030=CARTESIAN_POINT('Ctrl Pts',(38.1660413106006,32.757275993628,8.));
#22031=CARTESIAN_POINT('Ctrl Pts',(38.0987518751312,32.6552979021095,8.));
#22032=CARTESIAN_POINT('Ctrl Pts',(38.0308292899206,32.5523602632,8.));
#22033=CARTESIAN_POINT('Ctrl Pts',(37.9581357532083,32.4524200570822,8.));
#22034=CARTESIAN_POINT('Ctrl Pts',(37.8809718147757,32.3557926317859,8.));
#22035=CARTESIAN_POINT('Ctrl Pts',(37.8265588287192,32.2876547573834,8.));
#22036=CARTESIAN_POINT('Ctrl Pts',(37.7699218575833,32.221164530513,8.));
#22037=CARTESIAN_POINT('Ctrl Pts',(37.7111532334385,32.156441009698,8.));
#22038=CARTESIAN_POINT('Ctrl Pts',(37.6849201407301,32.1275497748485,8.));
#22039=CARTESIAN_POINT('Ctrl Pts',(37.6582621737227,32.0990106723795,8.));
#22040=CARTESIAN_POINT('Ctrl Pts',(37.6311869343715,32.0708348649218,8.));
#22041=CARTESIAN_POINT('Ctrl Pts',(37.6195644247842,32.0587399176506,8.));
#22042=CARTESIAN_POINT('Ctrl Pts',(37.6078664443942,32.0467134553255,8.));
#22043=CARTESIAN_POINT('Ctrl Pts',(37.5961000985213,32.0347627427216,8.));
#22044=CARTESIAN_POINT('Ctrl Pts',(37.5076578370054,31.9449346804806,8.));
#22045=CARTESIAN_POINT('Ctrl Pts',(37.4152562466455,31.8592792534028,8.));
#22046=CARTESIAN_POINT('Ctrl Pts',(37.3192240628069,31.7781146097001,8.));
#22047=CARTESIAN_POINT('Ctrl Pts',(37.2371844701374,31.7087762478888,8.));
#22048=CARTESIAN_POINT('Ctrl Pts',(37.1524942030697,31.6427153977926,8.));
#22049=CARTESIAN_POINT('Ctrl Pts',(37.0653339993003,31.5801479843188,8.));
#22050=CARTESIAN_POINT('Ctrl Pts',(37.026223350155,31.552072646602,8.));
#22051=CARTESIAN_POINT('Ctrl Pts',(36.9866151034059,31.5247009668187,8.));
#22052=CARTESIAN_POINT('Ctrl Pts',(36.9465243462331,31.4980538108418,8.));
#22053=CARTESIAN_POINT('Ctrl Pts',(36.9192915198287,31.4799529461023,8.));
#22054=CARTESIAN_POINT('Ctrl Pts',(36.891830409748,31.4621830185383,8.));
#22055=CARTESIAN_POINT('Ctrl Pts',(36.8641757039143,31.4447693408987,8.));
#22056=CARTESIAN_POINT('Ctrl Pts',(36.7573714959831,31.3775166259847,8.));
#22057=CARTESIAN_POINT('Ctrl Pts',(36.6476205511297,31.3155307102762,8.));
#22058=CARTESIAN_POINT('Ctrl Pts',(36.53522484258,31.2591452484686,8.));
#22059=CARTESIAN_POINT('Ctrl Pts',(36.4331310435836,31.2079279370747,8.));
#22060=CARTESIAN_POINT('Ctrl Pts',(36.328854296794,31.161331443821,8.));
#22061=CARTESIAN_POINT('Ctrl Pts',(36.2225975660985,31.1196349359533,8.));
#22062=CARTESIAN_POINT('Ctrl Pts',(36.1671670804927,31.0978833004188,8.));
#22063=CARTESIAN_POINT('Ctrl Pts',(36.1111974373468,31.0774656305418,8.));
#22064=CARTESIAN_POINT('Ctrl Pts',(36.0547327596422,31.0583698145405,8.));
#22065=CARTESIAN_POINT('Ctrl Pts',(33.9479286229388,31.0647048309474,8.));
#22066=CARTESIAN_POINT('Ctrl Pts',(33.8318204903556,31.1043195030892,8.));
#22067=CARTESIAN_POINT('Ctrl Pts',(33.7179774196666,31.1494845762766,8.));
#22068=CARTESIAN_POINT('Ctrl Pts',(33.6066253055996,31.1998424449166,8.));
#22069=CARTESIAN_POINT('Ctrl Pts',(33.4927760432216,31.2513296236524,8.));
#22070=CARTESIAN_POINT('Ctrl Pts',(33.3815300897553,31.3082456117247,8.));
#22071=CARTESIAN_POINT('Ctrl Pts',(33.2731531534421,31.3702567766217,8.));
#22072=CARTESIAN_POINT('Ctrl Pts',(33.1592147882362,31.4354500824416,8.));
#22073=CARTESIAN_POINT('Ctrl Pts',(33.0484464742462,31.5062753311388,8.));
#22074=CARTESIAN_POINT('Ctrl Pts',(32.9411961197039,31.5823910435948,8.));
#22075=CARTESIAN_POINT('Ctrl Pts',(32.8473520594793,31.6489922919938,8.));
#22076=CARTESIAN_POINT('Ctrl Pts',(32.7562017414451,31.719645109407,8.));
#22077=CARTESIAN_POINT('Ctrl Pts',(32.6680097346461,31.7941428733673,8.));
#22078=CARTESIAN_POINT('Ctrl Pts',(32.6506331562116,31.8088212584686,8.));
#22079=CARTESIAN_POINT('Ctrl Pts',(32.6333715252365,31.8236489611523,8.));
#22080=CARTESIAN_POINT('Ctrl Pts',(32.6162270200198,31.8386244719266,8.));
#22081=CARTESIAN_POINT('Ctrl Pts',(32.6036927426372,31.8495730063766,8.));
#22082=CARTESIAN_POINT('Ctrl Pts',(32.5912222824502,31.8605995500244,8.));
#22083=CARTESIAN_POINT('Ctrl Pts',(32.5788252877513,31.8716953917,8.));
#22084=CARTESIAN_POINT('Ctrl Pts',(32.4862461171128,31.9545577179984,8.));
#22085=CARTESIAN_POINT('Ctrl Pts',(32.397622799937,32.0414017436923,8.));
#22086=CARTESIAN_POINT('Ctrl Pts',(32.3132167630922,32.1319065542212,8.));
#22087=CARTESIAN_POINT('Ctrl Pts',(32.2290025191065,32.2222057138629,8.));
#22088=CARTESIAN_POINT('Ctrl Pts',(32.1489858942929,32.3161497454154,8.));
#22089=CARTESIAN_POINT('Ctrl Pts',(32.0734669664008,32.4134519537301,8.));
#22090=CARTESIAN_POINT('Ctrl Pts',(31.9989803737659,32.5094240517922,8.));
#22091=CARTESIAN_POINT('Ctrl Pts',(31.9288689532965,32.6086638275202,8.));
#22092=CARTESIAN_POINT('Ctrl Pts',(31.8634666824091,32.7109170108275,8.));
#22093=CARTESIAN_POINT('Ctrl Pts',(31.8101613092083,32.7942572989124,8.));
#22094=CARTESIAN_POINT('Ctrl Pts',(31.7599848998086,32.8795998826136,8.));
#22095=CARTESIAN_POINT('Ctrl Pts',(31.7131442187192,32.9668129344489,8.));
#22096=CARTESIAN_POINT('Ctrl Pts',(31.7012430571606,32.9889718056646,8.));
#22097=CARTESIAN_POINT('Ctrl Pts',(31.6895573606131,33.0112514414787,8.));
#22098=CARTESIAN_POINT('Ctrl Pts',(31.6780907836173,33.033649704911,8.));
#22099=CARTESIAN_POINT('Ctrl Pts',(31.6699353210994,33.0495801955843,8.));
#22100=CARTESIAN_POINT('Ctrl Pts',(31.6618944152098,33.0655635106099,8.));
#22101=CARTESIAN_POINT('Ctrl Pts',(31.6539717264445,33.0815932364824,8.));
#22102=CARTESIAN_POINT('Ctrl Pts',(31.6010109140258,33.1887471750268,8.));
#22103=CARTESIAN_POINT('Ctrl Pts',(31.5532889518817,33.2980509944504,8.));
#22104=CARTESIAN_POINT('Ctrl Pts',(31.5110846398564,33.4092420858783,8.));
#22105=CARTESIAN_POINT('Ctrl Pts',(31.469716484976,33.5182302453998,8.));
#22106=CARTESIAN_POINT('Ctrl Pts',(31.4336492415757,33.6290322689246,8.));
#22107=CARTESIAN_POINT('Ctrl Pts',(31.4031936775095,33.7414146337669,8.));
#22108=CARTESIAN_POINT('Ctrl Pts',(31.39873956261,33.7578505127609,8.));
#22109=CARTESIAN_POINT('Ctrl Pts',(31.3944055654848,33.7743202085893,8.));
#22110=CARTESIAN_POINT('Ctrl Pts',(31.3901927523269,33.7908230038594,8.));
#22111=CARTESIAN_POINT('Ctrl Pts',(31.3605242058421,33.9070431945601,8.));
#22112=CARTESIAN_POINT('Ctrl Pts',(31.3368616451868,34.0249053317963,8.));
#22113=CARTESIAN_POINT('Ctrl Pts',(31.3191142145135,34.1439735700009,8.));
#22114=CARTESIAN_POINT('Ctrl Pts',(31.3091306818643,34.210953498841,8.));
#22115=CARTESIAN_POINT('Ctrl Pts',(31.3010199124296,34.2783150418024,8.));
#22116=CARTESIAN_POINT('Ctrl Pts',(31.294772781286,34.3459791587903,8.));
#22117=CARTESIAN_POINT('Ctrl Pts',(31.2918903120279,34.3771998475526,8.));
#22118=CARTESIAN_POINT('Ctrl Pts',(31.2894046732663,34.4084849312592,8.));
#22119=CARTESIAN_POINT('Ctrl Pts',(31.2873153161224,34.4398265107474,8.));
#22120=CARTESIAN_POINT('Ctrl Pts',(31.2861142259533,34.4578435659536,8.));
#22121=CARTESIAN_POINT('Ctrl Pts',(31.2850446073883,34.4758722375043,8.));
#22122=CARTESIAN_POINT('Ctrl Pts',(31.2841063911591,34.4939026846615,8.));
#22123=CARTESIAN_POINT('Ctrl Pts',(31.2777954835053,34.6151844142158,8.));
#22124=CARTESIAN_POINT('Ctrl Pts',(31.2774171066952,34.7366634572185,8.));
#22125=CARTESIAN_POINT('Ctrl Pts',(31.2828130518753,34.8578925565699,8.));
#22126=CARTESIAN_POINT('Ctrl Pts',(31.2880970630825,34.976606868563,8.));
#22127=CARTESIAN_POINT('Ctrl Pts',(31.2989188151177,35.0950824227959,8.));
#22128=CARTESIAN_POINT('Ctrl Pts',(31.3151831142098,35.2128932340069,8.));
#22129=CARTESIAN_POINT('Ctrl Pts',(31.3312885029229,35.3295529743629,8.));
#22130=CARTESIAN_POINT('Ctrl Pts',(31.3527309554357,35.4455617346014,8.));
#22131=CARTESIAN_POINT('Ctrl Pts',(31.3794648241005,35.5604869939325,8.));
#22132=CARTESIAN_POINT('Ctrl Pts',(31.3968717446295,35.6353169738744,8.));
#22133=CARTESIAN_POINT('Ctrl Pts',(31.4165229267736,35.7096871840419,8.));
#22134=CARTESIAN_POINT('Ctrl Pts',(31.438415570696,35.7834713262069,8.));
#22135=CARTESIAN_POINT('Ctrl Pts',(31.4458039136858,35.8083720440668,8.));
#22136=CARTESIAN_POINT('Ctrl Pts',(31.4534476062533,35.833205958311,8.));
#22137=CARTESIAN_POINT('Ctrl Pts',(31.4613467284242,35.8579680375739,8.));
#22138=CARTESIAN_POINT('Ctrl Pts',(31.4664331210497,35.8739128039203,8.));
#22139=CARTESIAN_POINT('Ctrl Pts',(31.4716246314855,35.8898251737367,8.));
#22140=CARTESIAN_POINT('Ctrl Pts',(31.4769184005249,35.9056957806736,8.));
#22141=CARTESIAN_POINT('Ctrl Pts',(31.5138160950465,36.0163142837243,8.));
#22142=CARTESIAN_POINT('Ctrl Pts',(31.5557145002446,36.1250213095504,8.));
#22143=CARTESIAN_POINT('Ctrl Pts',(31.6025488222259,36.2313976553429,8.));
#22144=CARTESIAN_POINT('Ctrl Pts',(31.6406629285514,36.3179674866662,8.));
#22145=CARTESIAN_POINT('Ctrl Pts',(31.6820469422375,36.4029935647969,8.));
#22146=CARTESIAN_POINT('Ctrl Pts',(31.7266869246432,36.4862342957322,8.));
#22147=CARTESIAN_POINT('Ctrl Pts',(31.7483019214948,36.5265400494563,8.));
#22148=CARTESIAN_POINT('Ctrl Pts',(31.7706805722115,36.5664269742985,8.));
#22149=CARTESIAN_POINT('Ctrl Pts',(31.7938227675543,36.605866117211,8.));
#22150=CARTESIAN_POINT('Ctrl Pts',(31.8074092117442,36.6290202608064,8.));
#22151=CARTESIAN_POINT('Ctrl Pts',(31.8212608890592,36.6520231340321,8.));
#22152=CARTESIAN_POINT('Ctrl Pts',(31.8353637243995,36.6748463853764,8.));
#22153=CARTESIAN_POINT('Ctrl Pts',(31.8937951632988,36.7694086052589,8.));
#22154=CARTESIAN_POINT('Ctrl Pts',(31.9565778581775,36.8609656088156,8.));
#22155=CARTESIAN_POINT('Ctrl Pts',(32.0236777625255,36.9491266811452,8.));
#22156=CARTESIAN_POINT('Ctrl Pts',(32.0837085788304,37.0279998358789,8.));
#22157=CARTESIAN_POINT('Ctrl Pts',(32.1471954960693,37.1041548514456,8.));
#22158=CARTESIAN_POINT('Ctrl Pts',(32.2141376235347,37.177285414151,8.));
#22159=CARTESIAN_POINT('Ctrl Pts',(32.248992559173,37.2153624988329,8.));
#22160=CARTESIAN_POINT('Ctrl Pts',(32.2847845972398,37.2526191672925,8.));
#22161=CARTESIAN_POINT('Ctrl Pts',(32.321476328717,37.2890400220485,8.));
#22162=CARTESIAN_POINT('Origin',(-35.,-35.,10.2084234471775));
#22163=CARTESIAN_POINT('Ctrl Pts',(-39.0784093524563,-34.997955826836,7.70842344717746));
#22164=CARTESIAN_POINT('Ctrl Pts',(-39.0792534643083,-34.8668875745646,
7.70328437820511));
#22165=CARTESIAN_POINT('Ctrl Pts',(-39.0145241717454,-33.401902569157,7.64581193344868));
#22166=CARTESIAN_POINT('Ctrl Pts',(-37.2468182307978,-30.7615622415685,
7.53600611290816));
#22167=CARTESIAN_POINT('Ctrl Pts',(-32.7044906448315,-30.7882310811688,
7.37900598555592));
#22168=CARTESIAN_POINT('Ctrl Pts',(-30.2206288723714,-34.591050784955,7.22200585820366));
#22169=CARTESIAN_POINT('Ctrl Pts',(-32.0224449816578,-38.760868439734,7.06500573085141));
#22170=CARTESIAN_POINT('Ctrl Pts',(-36.4942781630208,-39.5581356918704,
6.90800560349915));
#22171=CARTESIAN_POINT('Ctrl Pts',(-38.8653532597229,-37.0673722499186,
6.78914484227451));
#22172=CARTESIAN_POINT('Ctrl Pts',(-39.0751760778997,-35.366983894328,6.72261745683394));
#22173=CARTESIAN_POINT('Ctrl Pts',(-39.0721140267755,-35.0034548068065,
6.70842344717746));
#22174=CARTESIAN_POINT('Ctrl Pts',(-39.0691247390887,-35.0040754761348,
7.79157655282255));
#22175=CARTESIAN_POINT('Ctrl Pts',(-39.0629617458988,-34.1015748206833,
7.75638428364687));
#22176=CARTESIAN_POINT('Ctrl Pts',(-38.3270258918815,-31.8449563360523,
7.6688586386871));
#22177=CARTESIAN_POINT('Ctrl Pts',(-34.6204730922247,-30.2191423808613,
7.52899961794324));
#22178=CARTESIAN_POINT('Ctrl Pts',(-30.8030823517117,-32.6774434597138,
7.37199949059099));
#22179=CARTESIAN_POINT('Ctrl Pts',(-30.7475655592404,-37.2202136561835,
7.21499936323873));
#22180=CARTESIAN_POINT('Ctrl Pts',(-34.5060129709306,-39.7711989299046,
7.05799923588648));
#22181=CARTESIAN_POINT('Ctrl Pts',(-38.2826810114871,-38.2186958612719,
6.91685829908109));
#22182=CARTESIAN_POINT('Ctrl Pts',(-39.0636923276262,-35.9315794222149,
6.82805073805978));
#22183=CARTESIAN_POINT('Ctrl Pts',(-39.0709664927331,-34.9967444357251,
6.79157655282255));
#22184=CARTESIAN_POINT('Ctrl Pts',(-32.3264680662287,-32.7141668369925,
8.));
#22185=CARTESIAN_POINT('Ctrl Pts',(-31.5748397248436,-33.5932784036375,
7.94766662421592));
#22186=CARTESIAN_POINT('Ctrl Pts',(-31.0185761455706,-36.1362135079881,
7.84299987264775));
#22187=CARTESIAN_POINT('Ctrl Pts',(-33.7549095310954,-38.9529268308332,
7.68599974529549));
#22188=CARTESIAN_POINT('Ctrl Pts',(-37.6085237505035,-38.2165103725086,
7.52899961794325));
#22189=CARTESIAN_POINT('Ctrl Pts',(-39.122629513254,-34.5999498459216,7.37199949059098));
#22190=CARTESIAN_POINT('Ctrl Pts',(-36.940145606194,-31.3400749195329,7.21499936323873));
#22191=CARTESIAN_POINT('Ctrl Pts',(-33.0178092164465,-31.3631036769391,
7.05799923588649));
#22192=CARTESIAN_POINT('Ctrl Pts',(-30.8729746062518,-34.6468690649513,
6.90099910853422));
#22193=CARTESIAN_POINT('Ctrl Pts',(-32.4288573028063,-38.2475401342247,
6.74399898118198));
#22194=CARTESIAN_POINT('Ctrl Pts',(-36.2903212074201,-38.9359868162892,
6.58699885382972));
#22195=CARTESIAN_POINT('Ctrl Pts',(-38.9947353103719,-36.0950579107052,
6.42999872647747));
#22196=CARTESIAN_POINT('Ctrl Pts',(-38.117035111845,-32.2721495171465,6.27299859912521));
#22197=CARTESIAN_POINT('Ctrl Pts',(-34.444258048923,-30.8953459884408,6.11599847177297));
#22198=CARTESIAN_POINT('Ctrl Pts',(-31.2698209074708,-33.1992175611906,
5.9589983444207));
#22199=CARTESIAN_POINT('Ctrl Pts',(-31.4402707556255,-37.1178717601522,
5.80199821706845));
#22200=CARTESIAN_POINT('Ctrl Pts',(-34.8027641605008,-39.1374081785836,
5.6449980897162));
#22201=CARTESIAN_POINT('Ctrl Pts',(-38.3421207391464,-37.4468919117391,
5.48799796236395));
#22202=CARTESIAN_POINT('Ctrl Pts',(-38.8845656356524,-33.5622237360543,
5.33099783501169));
#22203=CARTESIAN_POINT('Ctrl Pts',(-35.943683236251,-30.9668235565892,5.17399770765944));
#22204=CARTESIAN_POINT('Ctrl Pts',(-32.1565910373224,-31.9880112738199,
5.01699758030718));
#22205=CARTESIAN_POINT('Ctrl Pts',(-30.919210927847,-35.7100782334501,4.85999745295493));
#22206=CARTESIAN_POINT('Ctrl Pts',(-33.3411135315715,-38.7954112012017,
4.70299732560268));
#22207=CARTESIAN_POINT('Ctrl Pts',(-37.2505555447442,-38.477362547094,4.54599719825042));
#22208=CARTESIAN_POINT('Ctrl Pts',(-39.141902810795,-35.0411295298515,4.38899707089817));
#22209=CARTESIAN_POINT('Ctrl Pts',(-37.3191660904533,-31.5680152720272,
4.23199694354592));
#22210=CARTESIAN_POINT('Ctrl Pts',(-33.4168108878721,-31.1723946430222,
4.07499681619366));
#22211=CARTESIAN_POINT('Ctrl Pts',(-30.9341165505443,-34.2090244589174,
3.91799668884141));
#22212=CARTESIAN_POINT('Ctrl Pts',(-32.0973389085718,-37.9549296302039,
3.76099656148916));
#22213=CARTESIAN_POINT('Ctrl Pts',(-35.8634053144019,-39.0511210542994,
3.6039964341369));
#22214=CARTESIAN_POINT('Ctrl Pts',(-38.8552478911374,-36.5146333635664,
3.44699630678465));
#22215=CARTESIAN_POINT('Ctrl Pts',(-38.3900526994102,-32.6199594063295,
3.2899961794324));
#22216=CARTESIAN_POINT('Ctrl Pts',(-34.8849647272175,-30.8594906798889,
3.13299605208015));
#22217=CARTESIAN_POINT('Ctrl Pts',(-31.4830299921864,-32.8118563882867,
2.97599592472789));
#22218=CARTESIAN_POINT('Ctrl Pts',(-31.2347959944593,-36.726351454856,2.81899579737564));
#22219=CARTESIAN_POINT('Ctrl Pts',(-34.3628565683332,-39.0928106312356,
2.66199567002338));
#22220=CARTESIAN_POINT('Ctrl Pts',(-38.0622497333952,-37.7892072071444,
2.50499554267113));
#22221=CARTESIAN_POINT('Ctrl Pts',(-39.0156942580864,-33.9844950081716,
2.34799541531887));
#22222=CARTESIAN_POINT('Ctrl Pts',(-36.3682270687435,-31.0903957040226,
2.19099528796663));
#22223=CARTESIAN_POINT('Ctrl Pts',(-32.4938578387906,-31.7020764289629,
2.03399516061437));
#22224=CARTESIAN_POINT('Ctrl Pts',(-30.866769727096,-35.2710361541464,1.87699503326212));
#22225=CARTESIAN_POINT('Ctrl Pts',(-32.9459900633082,-38.5969565794207,
1.71999490590986));
#22226=CARTESIAN_POINT('Ctrl Pts',(-36.8670583779424,-38.6974486722808,
1.56299477855761));
#22227=CARTESIAN_POINT('Ctrl Pts',(-39.1139224428247,-35.4824088304557,
1.40599465120536));
#22228=CARTESIAN_POINT('Ctrl Pts',(-37.6717828958998,-31.8347767559132,
1.2489945238531));
#22229=CARTESIAN_POINT('Ctrl Pts',(-33.8338499179097,-31.0254541111767,
1.09199439650085));
#22230=CARTESIAN_POINT('Ctrl Pts',(-31.0415747701051,-33.7800977940573,
0.934994269148597));
#22231=CARTESIAN_POINT('Ctrl Pts',(-31.7989383549478,-37.6287343727556,
0.777994141796342));
#22232=CARTESIAN_POINT('Ctrl Pts',(-35.4265617474899,-39.1199684759325,
0.620994014444089));
#22233=CARTESIAN_POINT('Ctrl Pts',(-38.6720112486245,-36.9171723860524,
0.463993887091836));
#22234=CARTESIAN_POINT('Ctrl Pts',(-38.6240720221873,-32.9944536386984,
0.306993759739581));
#22235=CARTESIAN_POINT('Ctrl Pts',(-35.3277245214386,-30.8716914151866,
0.149993632387329));
#22236=CARTESIAN_POINT('Ctrl Pts',(-31.7348166906651,-32.4476562217995,
-0.00700649496492554));
#22237=CARTESIAN_POINT('Ctrl Pts',(-31.0753023569953,-36.3188879616356,
-0.164006622317179));
#22238=CARTESIAN_POINT('Ctrl Pts',(-32.9741442474368,-38.0994349533405,
-0.268673373885348));
#22239=CARTESIAN_POINT('Ctrl Pts',(-34.0915279074966,-38.3981590173419,
-0.321006749669432));
#22240=CARTESIAN_POINT('Ctrl Pts',(-32.1856025125516,-32.5937287191406,
8.10700224988981));
#22241=CARTESIAN_POINT('Ctrl Pts',(-31.3943716733878,-33.5191597390956,
8.05466887410573));
#22242=CARTESIAN_POINT('Ctrl Pts',(-30.8087991578366,-36.1960793891008,
7.95000212253755));
#22243=CARTESIAN_POINT('Ctrl Pts',(-33.6893070387277,-39.1612023407069,
7.79300199518531));
#22244=CARTESIAN_POINT('Ctrl Pts',(-37.7459640921552,-38.3859848825408,
7.63600186783305));
#22245=CARTESIAN_POINT('Ctrl Pts',(-39.3398464769469,-34.5788716288481,
7.4790017404808));
#22246=CARTESIAN_POINT('Ctrl Pts',(-37.0423698143953,-31.1472373602114,
7.32200161312854));
#22247=CARTESIAN_POINT('Ctrl Pts',(-32.9133696925748,-31.171479478349,7.1650014857763));
#22248=CARTESIAN_POINT('Ctrl Pts',(-30.6555260282916,-34.6282629716192,
7.00800135842403));
#22249=CARTESIAN_POINT('Ctrl Pts',(-32.2933865290902,-38.4186495693944,
6.85100123107179));
#22250=CARTESIAN_POINT('Ctrl Pts',(-36.358306859287,-39.1433697748163,6.69400110371953));
#22251=CARTESIAN_POINT('Ctrl Pts',(-39.2052136645597,-36.1527553471755,
6.53700097636729));
#22252=CARTESIAN_POINT('Ctrl Pts',(-38.2812683762075,-32.1284219768986,
6.38000084901502));
#22253=CARTESIAN_POINT('Ctrl Pts',(-34.4149765966796,-30.6790761348112,
6.22300072166278));
#22254=CARTESIAN_POINT('Ctrl Pts',(-31.073281738985,-33.1043362500341,6.06600059431052));
#22255=CARTESIAN_POINT('Ctrl Pts',(-31.2527124083266,-37.2294601703531,
5.90900046695826));
#22256=CARTESIAN_POINT('Ctrl Pts',(-34.792372013923,-39.3554038144322,5.75200033960602));
#22257=CARTESIAN_POINT('Ctrl Pts',(-38.5182135257814,-37.5758160437388,
5.59500021225375));
#22258=CARTESIAN_POINT('Ctrl Pts',(-39.0892392668699,-33.4864688341112,
5.43800008490151));
#22259=CARTESIAN_POINT('Ctrl Pts',(-35.9934049021458,-30.7543197799925,
5.28099995754925));
#22260=CARTESIAN_POINT('Ctrl Pts',(-32.0067748436954,-31.8293127917771,
5.12399983019699));
#22261=CARTESIAN_POINT('Ctrl Pts',(-30.7041984924888,-35.7474915002398,
4.96699970284474));
#22262=CARTESIAN_POINT('Ctrl Pts',(-33.2537085681557,-38.9953873801041,
4.80999957549249));
#22263=CARTESIAN_POINT('Ctrl Pts',(-37.3691349224156,-38.6605810807291,
4.65299944814024));
#22264=CARTESIAN_POINT('Ctrl Pts',(-39.3601352640338,-35.0432966010287,
4.49599932078798));
#22265=CARTESIAN_POINT('Ctrl Pts',(-37.4413604847951,-31.3871876474119,
4.33899919343573));
#22266=CARTESIAN_POINT('Ctrl Pts',(-33.3333943376382,-30.9707221882978,
4.18199906608348));
#22267=CARTESIAN_POINT('Ctrl Pts',(-30.7198894765905,-34.1673487990413,
4.02499893873122));
#22268=CARTESIAN_POINT('Ctrl Pts',(-31.9444007833091,-38.1106217291751,
3.86799881137897));
#22269=CARTESIAN_POINT('Ctrl Pts',(-35.9088972219885,-39.2645703133555,
3.71099868402671));
#22270=CARTESIAN_POINT('Ctrl Pts',(-39.0583768015825,-36.5944377843333,
3.55399855667446));
#22271=CARTESIAN_POINT('Ctrl Pts',(-38.5686709700449,-32.4945575991672,
3.39699842932221));
#22272=CARTESIAN_POINT('Ctrl Pts',(-34.8789036410609,-30.641331648192,3.23999830196996));
#22273=CARTESIAN_POINT('Ctrl Pts',(-31.2977245835776,-32.6965654289773,
3.0829981746177));
#22274=CARTESIAN_POINT('Ctrl Pts',(-31.0364114005639,-36.8173110766423,
2.92599804726545));
#22275=CARTESIAN_POINT('Ctrl Pts',(-34.3292861586667,-39.3084564697542,
2.76899791991319));
#22276=CARTESIAN_POINT('Ctrl Pts',(-38.2235964144439,-37.9361675679284,
2.61199779256094));
#22277=CARTESIAN_POINT('Ctrl Pts',(-39.2272769169348,-33.9309891303743,
2.45499766520869));
#22278=CARTESIAN_POINT('Ctrl Pts',(-36.4403174975728,-30.8844028124269,
2.29799753785644));
#22279=CARTESIAN_POINT('Ctrl Pts',(-32.3618118741726,-31.5283123441018,
2.14099741050418));
#22280=CARTESIAN_POINT('Ctrl Pts',(-30.6489942206534,-35.2853167607994,
1.98399728315193));
#22281=CARTESIAN_POINT('Ctrl Pts',(-32.8377664646538,-38.7864763954034,
1.82699715579967));
#22282=CARTESIAN_POINT('Ctrl Pts',(-36.9654316978321,-38.89226330974,1.66999702844742));
#22283=CARTESIAN_POINT('Ctrl Pts',(-39.3306806402386,-35.5078264385801,
1.51299690109516));
#22284=CARTESIAN_POINT('Ctrl Pts',(-37.8125562946319,-31.668004510122,1.35599677374291));
#22285=CARTESIAN_POINT('Ctrl Pts',(-33.7724067105519,-30.8160395161343,
1.19899664639066));
#22286=CARTESIAN_POINT('Ctrl Pts',(-30.8330095554335,-33.7158224444716,
1.04199651903841));
#22287=CARTESIAN_POINT('Ctrl Pts',(-31.630277821932,-37.7672395905951,0.884996391686153));
#22288=CARTESIAN_POINT('Ctrl Pts',(-35.4490368322191,-39.3370452323995,
0.727996264333899));
#22289=CARTESIAN_POINT('Ctrl Pts',(-38.8654856152897,-37.0181861597217,
0.570996136981647));
#22290=CARTESIAN_POINT('Ctrl Pts',(-38.815020522006,-32.8887835342792,0.413996009629392));
#22291=CARTESIAN_POINT('Ctrl Pts',(-35.3449919778631,-30.6541752272542,
0.256995882277139));
#22292=CARTESIAN_POINT('Ctrl Pts',(-31.5627776553664,-32.3131759431282,
0.0999957549248853));
#22293=CARTESIAN_POINT('Ctrl Pts',(-30.8685142129999,-36.3883787653949,
-0.0570043724273683));
#22294=CARTESIAN_POINT('Ctrl Pts',(-32.8674040627957,-38.2627408840732,
-0.161671123995537));
#22295=CARTESIAN_POINT('Ctrl Pts',(-34.0436614793107,-38.5772044012455,
-0.214004499779622));
#22296=CARTESIAN_POINT('Ctrl Pts',(-32.0447369588746,-32.4732906012887,
8.21400449977962));
#22297=CARTESIAN_POINT('Ctrl Pts',(-31.2139036219321,-33.4450410745538,
8.16167112399554));
#22298=CARTESIAN_POINT('Ctrl Pts',(-30.5990221701027,-36.2559452702134,
8.05700437242737));
#22299=CARTESIAN_POINT('Ctrl Pts',(-33.6237045463599,-39.3694778505807,
7.90000424507512));
#22300=CARTESIAN_POINT('Ctrl Pts',(-37.883404433807,-38.555459392573,7.74300411772286));
#22301=CARTESIAN_POINT('Ctrl Pts',(-39.5570634406398,-34.5577934117747,
7.58600399037061));
#22302=CARTESIAN_POINT('Ctrl Pts',(-37.1445940225965,-30.95439980089,7.42900386301835));
#22303=CARTESIAN_POINT('Ctrl Pts',(-32.8089301687032,-30.9798552797588,
7.2720037356661));
#22304=CARTESIAN_POINT('Ctrl Pts',(-30.4380774503315,-34.6096568782872,
7.11500360831385));
#22305=CARTESIAN_POINT('Ctrl Pts',(-32.157915755374,-38.5897590045642,6.9580034809616));
#22306=CARTESIAN_POINT('Ctrl Pts',(-36.4262925111539,-39.3507527333434,
6.80100335360934));
#22307=CARTESIAN_POINT('Ctrl Pts',(-39.4156920187475,-36.2104527836457,
6.64400322625709));
#22308=CARTESIAN_POINT('Ctrl Pts',(-38.4455016405701,-31.9846944366506,
6.48700309890483));
#22309=CARTESIAN_POINT('Ctrl Pts',(-34.3856951444362,-30.4628062811815,
6.33000297155259));
#22310=CARTESIAN_POINT('Ctrl Pts',(-30.8767425704992,-33.0094549388777,
6.17300284420032));
#22311=CARTESIAN_POINT('Ctrl Pts',(-31.0651540610276,-37.3410485805539,
6.01600271684808));
#22312=CARTESIAN_POINT('Ctrl Pts',(-34.7819798673453,-39.5733994502808,
5.85900258949582));
#22313=CARTESIAN_POINT('Ctrl Pts',(-38.6943063124164,-37.7047401757385,
5.70200246214356));
#22314=CARTESIAN_POINT('Ctrl Pts',(-39.2939128980875,-33.4107139321682,
5.54500233479131));
#22315=CARTESIAN_POINT('Ctrl Pts',(-36.0431265680407,-30.5418160033959,
5.38800220743906));
#22316=CARTESIAN_POINT('Ctrl Pts',(-31.8569586500684,-31.6706143097344,
5.2310020800868));
#22317=CARTESIAN_POINT('Ctrl Pts',(-30.4891860571307,-35.7849047670295,
5.07400195273456));
#22318=CARTESIAN_POINT('Ctrl Pts',(-33.1663036047398,-39.1953635590066,
4.9170018253823));
#22319=CARTESIAN_POINT('Ctrl Pts',(-37.487714300087,-38.8437996143642,4.76000169803005));
#22320=CARTESIAN_POINT('Ctrl Pts',(-39.5783677172726,-35.0454636722059,
4.60300157067779));
#22321=CARTESIAN_POINT('Ctrl Pts',(-37.563554879137,-31.2063600227966,4.44600144332554));
#22322=CARTESIAN_POINT('Ctrl Pts',(-33.2499777874043,-30.7690497335734,
4.28900131597329));
#22323=CARTESIAN_POINT('Ctrl Pts',(-30.5056624026368,-34.1256731391653,
4.13200118862103));
#22324=CARTESIAN_POINT('Ctrl Pts',(-31.7914626580464,-38.2663138281463,
3.97500106126878));
#22325=CARTESIAN_POINT('Ctrl Pts',(-35.9543891295751,-39.4780195724117,
3.81800093391652));
#22326=CARTESIAN_POINT('Ctrl Pts',(-39.2615057120276,-36.6742422051002,
3.66100080656427));
#22327=CARTESIAN_POINT('Ctrl Pts',(-38.7472892406796,-32.3691557920048,
3.50400067921202));
#22328=CARTESIAN_POINT('Ctrl Pts',(-34.8728425549044,-30.4231726164951,
3.34700055185977));
#22329=CARTESIAN_POINT('Ctrl Pts',(-31.1124191749688,-32.5812744696679,
3.19000042450751));
#22330=CARTESIAN_POINT('Ctrl Pts',(-30.8380268066686,-36.9082706984286,
3.03300029715526));
#22331=CARTESIAN_POINT('Ctrl Pts',(-34.295715749,-39.5241023082727,2.876000169803));
#22332=CARTESIAN_POINT('Ctrl Pts',(-38.3849430954928,-38.0831279287123,
2.71900004245075));
#22333=CARTESIAN_POINT('Ctrl Pts',(-39.438859575783,-33.8774832525769,2.5619999150985));
#22334=CARTESIAN_POINT('Ctrl Pts',(-36.5124079264021,-30.6784099208313,
2.40499978774625));
#22335=CARTESIAN_POINT('Ctrl Pts',(-32.2297659095544,-31.3545482592407,
2.24799966039399));
#22336=CARTESIAN_POINT('Ctrl Pts',(-30.4312187142109,-35.2995973674523,
2.09099953304174));
#22337=CARTESIAN_POINT('Ctrl Pts',(-32.7295428659994,-38.9759962113862,
1.93399940568948));
#22338=CARTESIAN_POINT('Ctrl Pts',(-37.0638050177218,-39.0870779471991,
1.77699927833723));
#22339=CARTESIAN_POINT('Ctrl Pts',(-39.5474388376525,-35.5332440467046,
1.61999915098498));
#22340=CARTESIAN_POINT('Ctrl Pts',(-37.953329693364,-31.5012322643307,1.46299902363272));
#22341=CARTESIAN_POINT('Ctrl Pts',(-33.7109635031942,-30.6066249210918,
1.30599889628047));
#22342=CARTESIAN_POINT('Ctrl Pts',(-30.624444340762,-33.6515470948858,1.14899876892822));
#22343=CARTESIAN_POINT('Ctrl Pts',(-31.4616172889162,-37.9057448084347,
0.991998641575964));
#22344=CARTESIAN_POINT('Ctrl Pts',(-35.4715119169482,-39.5541219888666,
0.83499851422371));
#22345=CARTESIAN_POINT('Ctrl Pts',(-39.0589599819549,-37.1191999333909,
0.677998386871458));
#22346=CARTESIAN_POINT('Ctrl Pts',(-39.0059690218246,-32.78311342986,0.520998259519202));
#22347=CARTESIAN_POINT('Ctrl Pts',(-35.3622594342876,-30.4366590393219,
0.36399813216695));
#22348=CARTESIAN_POINT('Ctrl Pts',(-31.3907386200676,-32.1786956644568,
0.206998004814696));
#22349=CARTESIAN_POINT('Ctrl Pts',(-30.6617260690046,-36.4578695691541,
0.0499978774624427));
#22350=CARTESIAN_POINT('Ctrl Pts',(-32.7606638781546,-38.426046814806,-0.0546688741057264));
#22351=CARTESIAN_POINT('Ctrl Pts',(-33.9957950511247,-38.756249785149,-0.107002249889811));
#22352=CARTESIAN_POINT('Ctrl Pts',(-31.9038714051976,-32.3528524834368,
8.32100674966943));
#22353=CARTESIAN_POINT('Ctrl Pts',(-31.0334355704763,-33.370922410012,8.26867337388535));
#22354=CARTESIAN_POINT('Ctrl Pts',(-30.3892451823686,-36.3158111513261,
8.16400662231718));
#22355=CARTESIAN_POINT('Ctrl Pts',(-33.5581020539921,-39.5777533604545,
8.00700649496493));
#22356=CARTESIAN_POINT('Ctrl Pts',(-38.0208447754587,-38.7249339026052,
7.85000636761267));
#22357=CARTESIAN_POINT('Ctrl Pts',(-39.7742804043327,-34.5367151947012,
7.69300624026042));
#22358=CARTESIAN_POINT('Ctrl Pts',(-37.2468182307978,-30.7615622415685,
7.53600611290816));
#22359=CARTESIAN_POINT('Ctrl Pts',(-32.7044906448315,-30.7882310811688,
7.37900598555592));
#22360=CARTESIAN_POINT('Ctrl Pts',(-30.2206288723714,-34.591050784955,7.22200585820366));
#22361=CARTESIAN_POINT('Ctrl Pts',(-32.0224449816578,-38.760868439734,7.06500573085141));
#22362=CARTESIAN_POINT('Ctrl Pts',(-36.4942781630208,-39.5581356918704,
6.90800560349915));
#22363=CARTESIAN_POINT('Ctrl Pts',(-39.6261703729353,-36.2681502201159,
6.75100547614691));
#22364=CARTESIAN_POINT('Ctrl Pts',(-38.6097349049326,-31.8409668964026,
6.59400534879464));
#22365=CARTESIAN_POINT('Ctrl Pts',(-34.3564136921927,-30.2465364275518,
6.4370052214424));
#22366=CARTESIAN_POINT('Ctrl Pts',(-30.6802034020135,-32.9145736277213,
6.28000509409013));
#22367=CARTESIAN_POINT('Ctrl Pts',(-30.8775957137286,-37.4526369907548,
6.12300496673789));
#22368=CARTESIAN_POINT('Ctrl Pts',(-34.7715877207675,-39.7913950861294,
5.96600483938563));
#22369=CARTESIAN_POINT('Ctrl Pts',(-38.8703990990513,-37.8336643077382,
5.80900471203337));
#22370=CARTESIAN_POINT('Ctrl Pts',(-39.498586529305,-33.3349590302252,5.65200458468112));
#22371=CARTESIAN_POINT('Ctrl Pts',(-36.0928482339355,-30.3293122267992,
5.49500445732888));
#22372=CARTESIAN_POINT('Ctrl Pts',(-31.7071424564414,-31.5119158276916,
5.33800432997661));
#22373=CARTESIAN_POINT('Ctrl Pts',(-30.2741736217725,-35.8223180338192,
5.18100420262437));
#22374=CARTESIAN_POINT('Ctrl Pts',(-33.0788986413239,-39.395339737909,5.02400407527211));
#22375=CARTESIAN_POINT('Ctrl Pts',(-37.6062936777584,-39.0270181479993,
4.86700394791986));
#22376=CARTESIAN_POINT('Ctrl Pts',(-39.7966001705114,-35.0476307433831,
4.7100038205676));
#22377=CARTESIAN_POINT('Ctrl Pts',(-37.6857492734788,-31.0255323981813,
4.55300369321535));
#22378=CARTESIAN_POINT('Ctrl Pts',(-33.1665612371704,-30.5673772788489,
4.39600356586309));
#22379=CARTESIAN_POINT('Ctrl Pts',(-30.291435328683,-34.0839974792893,4.23900343851084));
#22380=CARTESIAN_POINT('Ctrl Pts',(-31.6385245327839,-38.4220059271175,
4.08200331115859));
#22381=CARTESIAN_POINT('Ctrl Pts',(-35.9998810371616,-39.6914688314679,
3.92500318380634));
#22382=CARTESIAN_POINT('Ctrl Pts',(-39.4646346224728,-36.7540466258671,
3.76800305645408));
#22383=CARTESIAN_POINT('Ctrl Pts',(-38.9259075113142,-32.2437539848424,
3.61100292910183));
#22384=CARTESIAN_POINT('Ctrl Pts',(-34.8667814687478,-30.2050135847982,
3.45400280174957));
#22385=CARTESIAN_POINT('Ctrl Pts',(-30.9271137663599,-32.4659835103585,
3.29700267439732));
#22386=CARTESIAN_POINT('Ctrl Pts',(-30.6396422127733,-36.9992303202149,
3.14000254704507));
#22387=CARTESIAN_POINT('Ctrl Pts',(-34.2621453393335,-39.7397481467912,
2.98300241969281));
#22388=CARTESIAN_POINT('Ctrl Pts',(-38.5462897765416,-38.2300882894962,
2.82600229234056));
#22389=CARTESIAN_POINT('Ctrl Pts',(-39.6504422346313,-33.8239773747795,
2.66900216498831));
#22390=CARTESIAN_POINT('Ctrl Pts',(-36.5844983552314,-30.4724170292356,
2.51200203763606));
#22391=CARTESIAN_POINT('Ctrl Pts',(-32.0977199449364,-31.1807841743797,
2.3550019102838));
#22392=CARTESIAN_POINT('Ctrl Pts',(-30.2134432077683,-35.3138779741053,
2.19800178293155));
#22393=CARTESIAN_POINT('Ctrl Pts',(-32.621319267345,-39.1655160273689,2.04100165557929));
#22394=CARTESIAN_POINT('Ctrl Pts',(-37.1621783376115,-39.2818925846584,
1.88400152822705));
#22395=CARTESIAN_POINT('Ctrl Pts',(-39.7641970350665,-35.558661654829,1.72700140087479));
#22396=CARTESIAN_POINT('Ctrl Pts',(-38.0941030920961,-31.3344600185395,
1.57000127352254));
#22397=CARTESIAN_POINT('Ctrl Pts',(-33.6495202958365,-30.3972103260493,
1.41300114617028));
#22398=CARTESIAN_POINT('Ctrl Pts',(-30.4158791260905,-33.5872717453,1.25600101881803));
#22399=CARTESIAN_POINT('Ctrl Pts',(-31.2929567559004,-38.0442500262742,
1.09900089146578));
#22400=CARTESIAN_POINT('Ctrl Pts',(-35.4939870016774,-39.7711987453336,
0.942000764113521));
#22401=CARTESIAN_POINT('Ctrl Pts',(-39.2524343486202,-37.2202137070602,
0.785000636761268));
#22402=CARTESIAN_POINT('Ctrl Pts',(-39.1969175216432,-32.6774433254408,
0.628000509409014));
#22403=CARTESIAN_POINT('Ctrl Pts',(-35.3795268907121,-30.2191428513895,
0.471000382056761));
#22404=CARTESIAN_POINT('Ctrl Pts',(-31.2186995847689,-32.0442153857854,
0.314000254704507));
#22405=CARTESIAN_POINT('Ctrl Pts',(-30.4549379250093,-36.5273603729133,
0.157000127352253));
#22406=CARTESIAN_POINT('Ctrl Pts',(-32.6539236935135,-38.5893527455387,
0.0523333757840845));
#22407=CARTESIAN_POINT('Ctrl Pts',(-33.9479286229388,-38.9352951690526,
0.));
#22408=CARTESIAN_POINT('Ctrl Pts',(-33.9479286229388,-38.9352951690526,
5.55111512312578E-17));
#22409=CARTESIAN_POINT('Ctrl Pts',(-33.8318206360164,-38.8956805466085,
1.21569200333733E-16));
#22410=CARTESIAN_POINT('Ctrl Pts',(-33.7179777099102,-38.8505155072641,
1.50554103324791E-15));
#22411=CARTESIAN_POINT('Ctrl Pts',(-33.6066257375518,-38.8001576608968,
1.0547118733939E-15));
#22412=CARTESIAN_POINT('Ctrl Pts',(-33.492776560763,-38.7486704781164,5.93772317186044E-16));
#22413=CARTESIAN_POINT('Ctrl Pts',(-33.3815306925957,-38.6917544682482,
3.73522748729697E-15));
#22414=CARTESIAN_POINT('Ctrl Pts',(-33.2731538396993,-38.6297432688828,
2.72004641033163E-15));
#22415=CARTESIAN_POINT('Ctrl Pts',(-33.1592154520342,-38.5645498637963,
1.65276966251693E-15));
#22416=CARTESIAN_POINT('Ctrl Pts',(-33.048447119632,-38.4937244909346,-6.09647221355942E-16));
#22417=CARTESIAN_POINT('Ctrl Pts',(-32.9411967497889,-38.4176086362753,
-1.0547118733939E-15));
#22418=CARTESIAN_POINT('Ctrl Pts',(-32.8473526761762,-38.3510072634485,
-1.44414344392711E-15));
#22419=CARTESIAN_POINT('Ctrl Pts',(-32.7562023471369,-38.2803543077884,
-2.56653707031024E-15));
#22420=CARTESIAN_POINT('Ctrl Pts',(-32.6680103311015,-38.2058563963449,
-2.83106871279415E-15));
#22421=CARTESIAN_POINT('Ctrl Pts',(-32.6506345001076,-38.1911786151031,
-2.88318745685931E-15));
#22422=CARTESIAN_POINT('Ctrl Pts',(-32.6333736067294,-38.1763515287969,
-1.26352082166837E-15));
#22423=CARTESIAN_POINT('Ctrl Pts',(-32.6162298289787,-38.1613766467586,
-1.22124532708767E-15));
#22424=CARTESIAN_POINT('Ctrl Pts',(-32.6036955222168,-38.1504280817505,
-1.1903365025982E-15));
#22425=CARTESIAN_POINT('Ctrl Pts',(-32.5912250315541,-38.1394015059403,
9.6075348530294E-17));
#22426=CARTESIAN_POINT('Ctrl Pts',(-32.5788280068545,-38.1283056318751,
1.11022302462516E-16));
#22427=CARTESIAN_POINT('Ctrl Pts',(-32.4862488011484,-38.0454432328352,
2.22644014631185E-16));
#22428=CARTESIAN_POINT('Ctrl Pts',(-32.3976254460622,-37.9585991267844,
2.93313669984113E-16));
#22429=CARTESIAN_POINT('Ctrl Pts',(-32.3132193670584,-37.8680942341505,
1.66533453693773E-16));
#22430=CARTESIAN_POINT('Ctrl Pts',(-32.2290050385629,-37.7777949470768,
4.00412518592805E-17));
#22431=CARTESIAN_POINT('Ctrl Pts',(-32.1489883292395,-37.6838507826712,
-7.67367206503618E-16));
#22432=CARTESIAN_POINT('Ctrl Pts',(-32.0734693158047,-37.5865484422576,
-3.88578058618805E-16));
#22433=CARTESIAN_POINT('Ctrl Pts',(-31.9989826203281,-37.4905761901068,
-1.49668231824771E-17));
#22434=CARTESIAN_POINT('Ctrl Pts',(-31.9288710981801,-37.3913362593944,
6.39667558614738E-17));
#22435=CARTESIAN_POINT('Ctrl Pts',(-31.8634687260135,-37.2890829263301,
2.77555756156289E-16));
#22436=CARTESIAN_POINT('Ctrl Pts',(-31.8101631638829,-37.2057423498624,
4.51639376496992E-16));
#22437=CARTESIAN_POINT('Ctrl Pts',(-31.7599865782998,-37.1203994732574,
-1.91642689345195E-15));
#22438=CARTESIAN_POINT('Ctrl Pts',(-31.7131457346326,-37.0331861281649,
-2.08166817117217E-15));
#22439=CARTESIAN_POINT('Ctrl Pts',(-31.7012454402134,-37.0110288738836,
-2.12364905155618E-15));
#22440=CARTESIAN_POINT('Ctrl Pts',(-31.6895605787933,-36.988750873417,8.89729854294519E-16));
#22441=CARTESIAN_POINT('Ctrl Pts',(-31.6780948040882,-36.9663542633258,
9.71445146547012E-16));
#22442=CARTESIAN_POINT('Ctrl Pts',(-31.6699383315321,-36.9504218610016,
1.0295754129979E-15));
#22443=CARTESIAN_POINT('Ctrl Pts',(-31.661896440285,-36.9344366167593,-7.00903233658188E-16));
#22444=CARTESIAN_POINT('Ctrl Pts',(-31.6539727955662,-36.9184049530428,
-6.38378239159465E-16));
#22445=CARTESIAN_POINT('Ctrl Pts',(-31.6010119288307,-36.8112508799156,
-2.20467287978913E-16));
#22446=CARTESIAN_POINT('Ctrl Pts',(-31.5532899127003,-36.7019469405238,
-5.43579179869397E-17));
#22447=CARTESIAN_POINT('Ctrl Pts',(-31.5110855463215,-36.5907557494425,
2.77555756156289E-17));
#22448=CARTESIAN_POINT('Ctrl Pts',(-31.4697173372396,-36.4817674898051,
1.08242228141372E-16));
#22449=CARTESIAN_POINT('Ctrl Pts',(-31.433650039522,-36.3709653855926,-1.8533573671039E-16));
#22450=CARTESIAN_POINT('Ctrl Pts',(-31.4031944204139,-36.2585829650152,
-1.08246744900953E-15));
#22451=CARTESIAN_POINT('Ctrl Pts',(-31.3987402034729,-36.2421467310371,
-1.21367539645156E-15));
#22452=CARTESIAN_POINT('Ctrl Pts',(-31.3944061093602,-36.2256766793315,
1.54092145767103E-16));
#22453=CARTESIAN_POINT('Ctrl Pts',(-31.3901932043347,-36.2091735273543,
1.66533453693773E-16));
#22454=CARTESIAN_POINT('Ctrl Pts',(-31.3605246504064,-36.0929533297801,
3.08986100652746E-16));
#22455=CARTESIAN_POINT('Ctrl Pts',(-31.3368620771271,-35.9750912152647,
2.82593330474131E-15));
#22456=CARTESIAN_POINT('Ctrl Pts',(-31.319114629565,-35.8560230245863,3.49720252756924E-15));
#22457=CARTESIAN_POINT('Ctrl Pts',(-31.3091310875555,-35.7890431234222,
3.87481426369542E-15));
#22458=CARTESIAN_POINT('Ctrl Pts',(-31.3010203073581,-35.7216816160001,
-1.45794491220195E-16));
#22459=CARTESIAN_POINT('Ctrl Pts',(-31.294773164211,-35.6540175415704,-4.71844785465692E-16));
#22460=CARTESIAN_POINT('Ctrl Pts',(-31.2918906865937,-35.6227968418935,
-6.22286780009977E-16));
#22461=CARTESIAN_POINT('Ctrl Pts',(-31.2894050399855,-35.5915117486406,
3.58433295205778E-16));
#22462=CARTESIAN_POINT('Ctrl Pts',(-31.2873156755218,-35.5601701609149,
2.4980018054066E-16));
#22463=CARTESIAN_POINT('Ctrl Pts',(-31.286114583885,-35.5421531420771,1.87351370019253E-16));
#22464=CARTESIAN_POINT('Ctrl Pts',(-31.2850449634327,-35.5241245074566,
-4.29409397736477E-17));
#22465=CARTESIAN_POINT('Ctrl Pts',(-31.284106744896,-35.5060940976467,-5.55111512312578E-17));
#22466=CARTESIAN_POINT('Ctrl Pts',(-31.2777958135452,-35.3848124622,-1.40064737065375E-16));
#22467=CARTESIAN_POINT('Ctrl Pts',(-31.2774174094918,-35.2633335332142,
2.82866543587948E-15));
#22468=CARTESIAN_POINT('Ctrl Pts',(-31.282813324883,-35.142104562563,2.35922392732846E-15));
#22469=CARTESIAN_POINT('Ctrl Pts',(-31.2880973068045,-35.0233903791791,
1.89952056570822E-15));
#22470=CARTESIAN_POINT('Ctrl Pts',(-31.2989190268708,-34.9049149676345,
7.28996419448176E-16));
#22471=CARTESIAN_POINT('Ctrl Pts',(-31.3151832922329,-34.7871043083849,
6.93889390390723E-16));
#22472=CARTESIAN_POINT('Ctrl Pts',(-31.3312886503615,-34.670444698108,6.59125368578839E-16));
#22473=CARTESIAN_POINT('Ctrl Pts',(-31.3527310724264,-34.5544360772762,
1.70606179182567E-15));
#22474=CARTESIAN_POINT('Ctrl Pts',(-31.379464911652,-34.4395109622456,2.28983498828939E-15));
#22475=CARTESIAN_POINT('Ctrl Pts',(-31.3968718099089,-34.3646810896034,
2.66994053729605E-15));
#22476=CARTESIAN_POINT('Ctrl Pts',(-31.4165229694089,-34.2903109886468,
-2.96848706176688E-17));
#22477=CARTESIAN_POINT('Ctrl Pts',(-31.4384155905674,-34.2165269562934,
1.38777878078145E-17));
#22478=CARTESIAN_POINT('Ctrl Pts',(-31.4458039406444,-34.1916262257156,
2.85793700622958E-17));
#22479=CARTESIAN_POINT('Ctrl Pts',(-31.4534476413064,-34.1667922990885,
3.06223347651583E-15));
#22480=CARTESIAN_POINT('Ctrl Pts',(-31.4613467725894,-34.1420302077573,
3.1641356201817E-15));
#22481=CARTESIAN_POINT('Ctrl Pts',(-31.4664331829338,-34.1260853964884,
3.22975247083094E-15));
#22482=CARTESIAN_POINT('Ctrl Pts',(-31.4716247119601,-34.1101729821539,
1.52985938675526E-15));
#22483=CARTESIAN_POINT('Ctrl Pts',(-31.4769185004878,-34.0943023310132,
1.56819002228303E-15));
#22484=CARTESIAN_POINT('Ctrl Pts',(-31.5138161753674,-33.9836839859762,
1.8353543263008E-15));
#22485=CARTESIAN_POINT('Ctrl Pts',(-31.5557145621555,-33.8749771180903,
2.68190903327311E-15));
#22486=CARTESIAN_POINT('Ctrl Pts',(-31.60254886788,-33.7686009256992,2.26207941267376E-15));
#22487=CARTESIAN_POINT('Ctrl Pts',(-31.6406629427424,-33.6820312606289,
1.92041922701669E-15));
#22488=CARTESIAN_POINT('Ctrl Pts',(-31.6820469232643,-33.5970053442715,
1.26636124083292E-15));
#22489=CARTESIAN_POINT('Ctrl Pts',(-31.7266868713332,-33.5137647678308,
1.40165656858926E-15));
#22490=CARTESIAN_POINT('Ctrl Pts',(-31.7483018585373,-33.473459075901,1.46716754933025E-15));
#22491=CARTESIAN_POINT('Ctrl Pts',(-31.7706804998245,-33.4335722114158,
1.17298588323861E-16));
#22492=CARTESIAN_POINT('Ctrl Pts',(-31.7938226860146,-33.3941331271239,
-4.02455846426619E-16));
#22493=CARTESIAN_POINT('Ctrl Pts',(-31.8074090785167,-33.3709790968731,
-7.07595028060502E-16));
#22494=CARTESIAN_POINT('Ctrl Pts',(-31.8212607024029,-33.3479763354121,
-4.73580047421181E-16));
#22495=CARTESIAN_POINT('Ctrl Pts',(-31.8353634826968,-33.3251531939272,
-3.88578058618805E-16));
#22496=CARTESIAN_POINT('Ctrl Pts',(-31.8937949297824,-33.2305910468749,
-3.63929499130585E-17));
#22497=CARTESIAN_POINT('Ctrl Pts',(-31.9565776402818,-33.1390341079118,
1.65098064735663E-15));
#22498=CARTESIAN_POINT('Ctrl Pts',(-32.0236775684477,-33.0508730884183,
2.24126273096203E-15));
#22499=CARTESIAN_POINT('Ctrl Pts',(-32.0837083254303,-32.9720000868933,
2.76935689262062E-15));
#22500=CARTESIAN_POINT('Ctrl Pts',(-32.1471951806296,-32.895845207831,1.97196154581884E-15));
#22501=CARTESIAN_POINT('Ctrl Pts',(-32.2141372439519,-32.8227147610826,
2.21437451708439E-15));
#22502=CARTESIAN_POINT('Ctrl Pts',(-32.2489921734814,-32.7846377069649,
2.36892565463969E-15));
#22503=CARTESIAN_POINT('Ctrl Pts',(-32.2847842063358,-32.7473810647789,
1.32299506859179E-17));
#22504=CARTESIAN_POINT('Ctrl Pts',(-32.3214759334524,-32.7109602322923,
-5.55111512312578E-17));
#22505=CARTESIAN_POINT('Ctrl Pts',(-38.5163032009778,-35.0029832534533,
6.38741669750803));
#22506=CARTESIAN_POINT('Ctrl Pts',(-38.5189473067417,-35.316893543218,6.40161070716451));
#22507=CARTESIAN_POINT('Ctrl Pts',(-38.4802906988737,-35.6301637893069,
6.41580471682099));
#22508=CARTESIAN_POINT('Ctrl Pts',(-38.3977162601254,-35.9313946627094,
6.42999872647747));
#22509=CARTESIAN_POINT('Ctrl Pts',(-38.0932639427213,-37.0420342125665,
6.48233210226156));
#22510=CARTESIAN_POINT('Ctrl Pts',(-37.1917925750707,-37.9890105144279,
6.53466547804564));
#22511=CARTESIAN_POINT('Ctrl Pts',(-36.0974795738098,-38.3477575516811,
6.58699885382972));
#22512=CARTESIAN_POINT('Ctrl Pts',(-35.0031665725488,-38.7065045889344,
6.63933222961381));
#22513=CARTESIAN_POINT('Ctrl Pts',(-33.7160119376775,-38.4770223615795,
6.69166560539789));
#22514=CARTESIAN_POINT('Ctrl Pts',(-32.8131208374828,-37.7621694030232,
6.74399898118198));
#22515=CARTESIAN_POINT('Ctrl Pts',(-31.9102297372881,-37.0473164444669,
6.79633235696606));
#22516=CARTESIAN_POINT('Ctrl Pts',(-31.3916021717699,-35.8470927547091,
6.84866573275014));
#22517=CARTESIAN_POINT('Ctrl Pts',(-31.4897608240433,-34.6996866784948,
6.90099910853423));
#22518=CARTESIAN_POINT('Ctrl Pts',(-31.5879194763167,-33.5522806022806,
6.95333248431831));
#22519=CARTESIAN_POINT('Ctrl Pts',(-32.3028643463816,-32.4576921396098,
7.0056658601024));
#22520=CARTESIAN_POINT('Ctrl Pts',(-33.3140595130386,-31.9065597820401,
7.05799923588649));
#22521=CARTESIAN_POINT('Ctrl Pts',(-34.3252546796956,-31.3554274244703,
7.11033261167057));
#22522=CARTESIAN_POINT('Ctrl Pts',(-35.6327001429448,-31.3477511720016,
7.16266598745465));
#22523=CARTESIAN_POINT('Ctrl Pts',(-36.6501701924127,-31.8872255334987,
7.21499936323874));
#22524=CARTESIAN_POINT('Ctrl Pts',(-37.6676402418807,-32.4266998949958,
7.26733273902282));
#22525=CARTESIAN_POINT('Ctrl Pts',(-38.3951348775673,-33.5133248704587,
7.3196661148069));
#22526=CARTESIAN_POINT('Ctrl Pts',(-38.5065312349523,-34.6593974459546,
7.37199949059099));
#22527=CARTESIAN_POINT('Ctrl Pts',(-38.5174702113759,-34.7719402721061,
7.37713855956333));
#22528=CARTESIAN_POINT('Ctrl Pts',(-38.5224681626868,-34.8850563504433,
7.38227762853568));
#22529=CARTESIAN_POINT('Ctrl Pts',(-38.5217392653161,-34.9982348400382,
7.38741669750802));
#22530=CARTESIAN_POINT('Ctrl Pts',(-36.0520713770612,-38.9352951690526,
8.));
#22531=CARTESIAN_POINT('Ctrl Pts',(-37.3460763064865,-38.5893527455387,
7.94766662421592));
#22532=CARTESIAN_POINT('Ctrl Pts',(-39.5450618542894,-36.527358944407,7.84299987264775));
#22533=CARTESIAN_POINT('Ctrl Pts',(-38.7813006061664,-32.0442159203332,
7.6859997452955));
#22534=CARTESIAN_POINT('Ctrl Pts',(-34.6204730922247,-30.2191423808613,
7.52899961794324));
#22535=CARTESIAN_POINT('Ctrl Pts',(-30.8030823517117,-32.6774434597138,
7.37199949059099));
#22536=CARTESIAN_POINT('Ctrl Pts',(-30.7475655592404,-37.2202136561835,
7.21499936323873));
#22537=CARTESIAN_POINT('Ctrl Pts',(-34.5060129709306,-39.7711989299046,
7.05799923588648));
#22538=CARTESIAN_POINT('Ctrl Pts',(-38.7070433506006,-38.044250072918,6.90099910853423));
#22539=CARTESIAN_POINT('Ctrl Pts',(-39.584120987438,-33.5872717262032,6.74399898118198));
#22540=CARTESIAN_POINT('Ctrl Pts',(-36.3504797430715,-30.3972101963624,
6.58699885382972));
#22541=CARTESIAN_POINT('Ctrl Pts',(-31.905896825022,-31.3344599279876,6.42999872647746));
#22542=CARTESIAN_POINT('Ctrl Pts',(-30.2358028418083,-35.5586616666892,
6.27299859912522));
#22543=CARTESIAN_POINT('Ctrl Pts',(-32.83782160528,-39.2818926978495,6.11599847177295));
#22544=CARTESIAN_POINT('Ctrl Pts',(-37.3786807951101,-39.1655161353224,
5.95899834442071));
#22545=CARTESIAN_POINT('Ctrl Pts',(-39.7865569169479,-35.3138779826965,
5.80199821706845));
#22546=CARTESIAN_POINT('Ctrl Pts',(-37.9022801309199,-31.1807840744948,
5.64499808971621));
#22547=CARTESIAN_POINT('Ctrl Pts',(-33.4155016033557,-30.4724169111822,
5.48799796236394));
#22548=CARTESIAN_POINT('Ctrl Pts',(-30.3495576440316,-33.8239773440302,
5.3309978350117));
#22549=CARTESIAN_POINT('Ctrl Pts',(-31.4537101308888,-38.230088373826,5.17399770765944));
#22550=CARTESIAN_POINT('Ctrl Pts',(-35.7378546799324,-39.7397482704758,
5.01699758030718));
#22551=CARTESIAN_POINT('Ctrl Pts',(-39.3603579010204,-36.9992303723996,
4.85999745295493));
#22552=CARTESIAN_POINT('Ctrl Pts',(-39.0728863399384,-32.4659834442205,
4.70299732560268));
#22553=CARTESIAN_POINT('Ctrl Pts',(-35.1332185347277,-30.2050134596587,
4.54599719825043));
#22554=CARTESIAN_POINT('Ctrl Pts',(-31.0740923862265,-32.2437539129077,
4.38899707089817));
#22555=CARTESIAN_POINT('Ctrl Pts',(-30.535365261007,-36.7540466716456,4.23199694354592));
#22556=CARTESIAN_POINT('Ctrl Pts',(-34.0001189367432,-39.6914689539076,
4.07499681619366));
#22557=CARTESIAN_POINT('Ctrl Pts',(-38.3614755549453,-38.4220060164266,
3.91799668884141));
#22558=CARTESIAN_POINT('Ctrl Pts',(-39.7085647942032,-34.0839974553828,
3.76099656148916));
#22559=CARTESIAN_POINT('Ctrl Pts',(-36.8334388106793,-30.5673771631648,
3.6039964341369));
#22560=CARTESIAN_POINT('Ctrl Pts',(-32.3142506564274,-31.0255322944533,
3.44699630678465));
#22561=CARTESIAN_POINT('Ctrl Pts',(-30.2033997043049,-35.0476307446275,
3.28999617943239));
#22562=CARTESIAN_POINT('Ctrl Pts',(-32.3937062542216,-39.0270182530956,
3.13299605208014));
#22563=CARTESIAN_POINT('Ctrl Pts',(-36.9211014088136,-39.3953398526252,
2.97599592472789));
#22564=CARTESIAN_POINT('Ctrl Pts',(-39.7258265015647,-35.8223180552711,
2.81899579737564));
#22565=CARTESIAN_POINT('Ctrl Pts',(-38.2928576294957,-31.5119157366759,
2.66199567002338));
#22566=CARTESIAN_POINT('Ctrl Pts',(-33.9071517375455,-30.3293121048675,
2.50499554267113));
#22567=CARTESIAN_POINT('Ctrl Pts',(-30.5014133532831,-33.3349589868354,
2.34799541531887));
#22568=CARTESIAN_POINT('Ctrl Pts',(-31.12960079995,-37.8336643815683,2.19099528796663));
#22569=CARTESIAN_POINT('Ctrl Pts',(-35.2284122851668,-39.7913952114128,
2.03399516061437));
#22570=CARTESIAN_POINT('Ctrl Pts',(-39.1224043939168,-37.4526370543192,
1.87699503326212));
#22571=CARTESIAN_POINT('Ctrl Pts',(-39.3197967106052,-32.9145735741338,
1.71999490590986));
#22572=CARTESIAN_POINT('Ctrl Pts',(-35.6435863248602,-30.2465363019221,
1.56299477855761));
#22573=CARTESIAN_POINT('Ctrl Pts',(-31.3902650003177,-31.8409668168855,
1.40599465120536));
#22574=CARTESIAN_POINT('Ctrl Pts',(-30.3738295074692,-36.2681502477922,
1.2489945238531));
#22575=CARTESIAN_POINT('Ctrl Pts',(-33.5057217955833,-39.5581358207848,
1.09199439650085));
#22576=CARTESIAN_POINT('Ctrl Pts',(-37.977555101084,-38.7608685197788,0.934994269148597));
#22577=CARTESIAN_POINT('Ctrl Pts',(-39.7793712418172,-34.5910508068424,
0.777994141796343));
#22578=CARTESIAN_POINT('Ctrl Pts',(-37.2955094371433,-30.7882309135474,
0.620994014444089));
#22579=CARTESIAN_POINT('Ctrl Pts',(-32.7531816644513,-30.7615622313046,
0.463993887091836));
#22580=CARTESIAN_POINT('Ctrl Pts',(-30.2257195673566,-34.5367150123096,
0.306993759739581));
#22581=CARTESIAN_POINT('Ctrl Pts',(-31.9791549439529,-38.7249342807031,
0.149993632387329));
#22582=CARTESIAN_POINT('Ctrl Pts',(-36.441898406148,-39.5777530280863,-0.00700649496492615));
#22583=CARTESIAN_POINT('Ctrl Pts',(-39.6107538265857,-36.3158122035465,
-0.164006622317178));
#22584=CARTESIAN_POINT('Ctrl Pts',(-38.9665644295237,-33.3709224100119,
-0.268673373885348));
#22585=CARTESIAN_POINT('Ctrl Pts',(-38.0961285948024,-32.3528524834368,
-0.321006749669432));
#22586=CARTESIAN_POINT('Ctrl Pts',(-36.0042049488753,-38.756249785149,8.10700224988981));
#22587=CARTESIAN_POINT('Ctrl Pts',(-37.2393361218454,-38.4260468148059,
8.05466887410573));
#22588=CARTESIAN_POINT('Ctrl Pts',(-39.3382737203354,-36.457868205641,7.95000212253756));
#22589=CARTESIAN_POINT('Ctrl Pts',(-38.6092615621806,-32.178696174684,7.7930019951853));
#22590=CARTESIAN_POINT('Ctrl Pts',(-34.6377405494255,-30.4366585902015,
7.63600186783305));
#22591=CARTESIAN_POINT('Ctrl Pts',(-30.9940308572923,-32.7831135580239,
7.4790017404808));
#22592=CARTESIAN_POINT('Ctrl Pts',(-30.9410399300978,-37.119199884829,7.32200161312854));
#22593=CARTESIAN_POINT('Ctrl Pts',(-34.528488056906,-39.5541221650401,7.16500148577629));
#22594=CARTESIAN_POINT('Ctrl Pts',(-38.5383828127393,-37.9057448529564,
7.00800135842404));
#22595=CARTESIAN_POINT('Ctrl Pts',(-39.3755557676012,-33.6515470766578,
6.85100123107178));
#22596=CARTESIAN_POINT('Ctrl Pts',(-36.2890365339436,-30.6066247973054,
6.69400110371953));
#22597=CARTESIAN_POINT('Ctrl Pts',(-32.046670227525,-31.5012321778987,6.53700097636728));
#22598=CARTESIAN_POINT('Ctrl Pts',(-30.4525610448241,-35.5332440580251,
6.38000084901503));
#22599=CARTESIAN_POINT('Ctrl Pts',(-32.936194927768,-39.0870780552405,6.22300072166276));
#22600=CARTESIAN_POINT('Ctrl Pts',(-37.2704571936142,-38.975996314428,6.06600059431052));
#22601=CARTESIAN_POINT('Ctrl Pts',(-39.5687814048312,-35.2995973756527,
5.90900046695826));
#22602=CARTESIAN_POINT('Ctrl Pts',(-37.7702341628505,-31.3545481639004,
5.75200033960601));
#22603=CARTESIAN_POINT('Ctrl Pts',(-33.4875920340692,-30.678409808149,5.59500021225376));
#22604=CARTESIAN_POINT('Ctrl Pts',(-30.5611403084004,-33.8774832232266,
5.4380000849015));
#22605=CARTESIAN_POINT('Ctrl Pts',(-31.6150568161493,-38.0831280092054,
5.28099995754926));
#22606=CARTESIAN_POINT('Ctrl Pts',(-35.7042842693892,-39.5241024263299,
5.12399983019699));
#22607=CARTESIAN_POINT('Ctrl Pts',(-39.1619733019478,-36.908270748239,4.96699970284474));
#22608=CARTESIAN_POINT('Ctrl Pts',(-38.8875809264933,-32.581274406539,4.80999957549249));
#22609=CARTESIAN_POINT('Ctrl Pts',(-35.127157448413,-30.4231724970492,4.65299944814023));
#22610=CARTESIAN_POINT('Ctrl Pts',(-31.2527106615227,-32.3691557233429,
4.49599932078798));
#22611=CARTESIAN_POINT('Ctrl Pts',(-30.7384941767535,-36.6742422487958,
4.33899919343573));
#22612=CARTESIAN_POINT('Ctrl Pts',(-34.045610845517,-39.4780196892807,4.18199906608348));
#22613=CARTESIAN_POINT('Ctrl Pts',(-38.2085374256912,-38.2663139133921,
4.02499893873122));
#22614=CARTESIAN_POINT('Ctrl Pts',(-39.4943377146584,-34.1256731163465,
3.86799881137897));
#22615=CARTESIAN_POINT('Ctrl Pts',(-36.7500222582684,-30.7690496231526,
3.71099868402672));
#22616=CARTESIAN_POINT('Ctrl Pts',(-32.4364450539584,-31.206359923788,3.55399855667446));
#22617=CARTESIAN_POINT('Ctrl Pts',(-30.4216321632391,-35.0454636733936,
3.39699842932221));
#22618=CARTESIAN_POINT('Ctrl Pts',(-32.5122856349878,-38.843799714679,3.23999830196996));
#22619=CARTESIAN_POINT('Ctrl Pts',(-36.8336964431165,-39.1953636685035,
3.0829981746177));
#22620=CARTESIAN_POINT('Ctrl Pts',(-39.510814060595,-35.7849047875054,2.92599804726545));
#22621=CARTESIAN_POINT('Ctrl Pts',(-38.1430414319588,-31.6706142228596,
2.76899791991319));
#22622=CARTESIAN_POINT('Ctrl Pts',(-33.9568734047379,-30.5418158870118,
2.61199779256094));
#22623=CARTESIAN_POINT('Ctrl Pts',(-30.7060869898426,-33.4107138907526,
2.45499766520869));
#22624=CARTESIAN_POINT('Ctrl Pts',(-31.3056935911801,-37.7047402462095,
2.29799753785644));
#22625=CARTESIAN_POINT('Ctrl Pts',(-35.2180201383191,-39.5733995698641,
2.14099741050418));
#22626=CARTESIAN_POINT('Ctrl Pts',(-38.9348460417202,-37.3410486412263,
1.98399728315193));
#22627=CARTESIAN_POINT('Ctrl Pts',(-39.1232575369955,-33.0094548877283,
1.82699715579967));
#22628=CARTESIAN_POINT('Ctrl Pts',(-35.614304871841,-30.4628061612676,1.66999702844742));
#22629=CARTESIAN_POINT('Ctrl Pts',(-31.5544982689911,-31.9846943607513,
1.51299690109517));
#22630=CARTESIAN_POINT('Ctrl Pts',(-30.5843078670984,-36.2104528100627,
1.35599677374291));
#22631=CARTESIAN_POINT('Ctrl Pts',(-33.5737074493336,-39.3507528563925,
1.19899664639066));
#22632=CARTESIAN_POINT('Ctrl Pts',(-37.8420843236033,-38.5897590809672,
1.04199651903841));
#22633=CARTESIAN_POINT('Ctrl Pts',(-39.5619226586618,-34.6096568991787,
0.884996391686153));
#22634=CARTESIAN_POINT('Ctrl Pts',(-37.191069909542,-30.9798551197638,0.7279962643339));
#22635=CARTESIAN_POINT('Ctrl Pts',(-32.8554058774184,-30.954399791093,0.570996136981647));
#22636=CARTESIAN_POINT('Ctrl Pts',(-30.4429365323376,-34.5577932376814,
0.413996009629392));
#22637=CARTESIAN_POINT('Ctrl Pts',(-32.1165952983707,-38.5554597534685,
0.25699588227714));
#22638=CARTESIAN_POINT('Ctrl Pts',(-36.3762958928451,-39.3694775333344,
0.0999957549248847));
#22639=CARTESIAN_POINT('Ctrl Pts',(-39.4009768839417,-36.2559462745606,
-0.0570043724273669));
#22640=CARTESIAN_POINT('Ctrl Pts',(-38.7860963780679,-33.4450410745538,
-0.161671123995537));
#22641=CARTESIAN_POINT('Ctrl Pts',(-37.9552630411254,-32.4732906012887,
-0.214004499779622));
#22642=CARTESIAN_POINT('Ctrl Pts',(-35.9563385206894,-38.5772044012455,
8.21400449977962));
#22643=CARTESIAN_POINT('Ctrl Pts',(-37.1325959372043,-38.2627408840732,
8.16167112399554));
#22644=CARTESIAN_POINT('Ctrl Pts',(-39.1314855863814,-36.388377466875,8.05700437242737));
#22645=CARTESIAN_POINT('Ctrl Pts',(-38.4372225181948,-32.3131764290349,
7.90000424507512));
#22646=CARTESIAN_POINT('Ctrl Pts',(-34.6550080066264,-30.6541747995416,
7.74300411772286));
#22647=CARTESIAN_POINT('Ctrl Pts',(-31.184979362873,-32.8887836563341,7.58600399037061));
#22648=CARTESIAN_POINT('Ctrl Pts',(-31.1345143009551,-37.0181861134745,
7.42900386301835));
#22649=CARTESIAN_POINT('Ctrl Pts',(-34.5509631428814,-39.3370454001755,
7.2720037356661));
#22650=CARTESIAN_POINT('Ctrl Pts',(-38.3697222748781,-37.7672396329946,
7.11500360831385));
#22651=CARTESIAN_POINT('Ctrl Pts',(-39.1669905477644,-33.7158224271125,
6.95800348096159));
#22652=CARTESIAN_POINT('Ctrl Pts',(-36.2275933248156,-30.8160393982482,
6.80100335360935));
#22653=CARTESIAN_POINT('Ctrl Pts',(-32.187443630028,-31.6680044278098,6.64400322625708));
#22654=CARTESIAN_POINT('Ctrl Pts',(-30.6693192478399,-35.5078264493611,
6.48700309890484));
#22655=CARTESIAN_POINT('Ctrl Pts',(-33.0345682502559,-38.8922634126314,
6.33000297155257));
#22656=CARTESIAN_POINT('Ctrl Pts',(-37.1622335921182,-38.7864764935337,
6.17300284420033));
#22657=CARTESIAN_POINT('Ctrl Pts',(-39.3510058927144,-35.2853167686088,
6.01600271684807));
#22658=CARTESIAN_POINT('Ctrl Pts',(-37.6381881947812,-31.5283122533059,
5.85900258949583));
#22659=CARTESIAN_POINT('Ctrl Pts',(-33.5596824647827,-30.8844027051158,
5.70200246214357));
#22660=CARTESIAN_POINT('Ctrl Pts',(-30.7727229727691,-33.9309891024229,
5.54500233479131));
#22661=CARTESIAN_POINT('Ctrl Pts',(-31.7764035014098,-37.9361676445846,
5.38800220743907));
#22662=CARTESIAN_POINT('Ctrl Pts',(-35.6707138588461,-39.3084565821841,
5.2310020800868));
#22663=CARTESIAN_POINT('Ctrl Pts',(-38.9635887028751,-36.8173111240784,
5.07400195273455));
#22664=CARTESIAN_POINT('Ctrl Pts',(-38.7022755130482,-32.6965653688576,
4.9170018253823));
#22665=CARTESIAN_POINT('Ctrl Pts',(-35.1210963620983,-30.6413315344396,
4.76000169803004));
#22666=CARTESIAN_POINT('Ctrl Pts',(-31.431328936819,-32.4945575337781,4.6030015706778));
#22667=CARTESIAN_POINT('Ctrl Pts',(-30.9416230925,-36.5944378259461,4.44600144332554));
#22668=CARTESIAN_POINT('Ctrl Pts',(-34.0911027542909,-39.2645704246538,
4.28900131597328));
#22669=CARTESIAN_POINT('Ctrl Pts',(-38.0555992964371,-38.1106218103576,
4.13200118862104));
#22670=CARTESIAN_POINT('Ctrl Pts',(-39.2801106351136,-34.1673487773102,
3.97500106126878));
#22671=CARTESIAN_POINT('Ctrl Pts',(-36.6666057058575,-30.9707220831404,
3.81800093391653));
#22672=CARTESIAN_POINT('Ctrl Pts',(-32.5586394514893,-31.3871875531226,
3.66100080656427));
#22673=CARTESIAN_POINT('Ctrl Pts',(-30.6398646221734,-35.0432966021599,
3.50400067921202));
#22674=CARTESIAN_POINT('Ctrl Pts',(-32.6308650157539,-38.6605811762622,
3.34700055185977));
#22675=CARTESIAN_POINT('Ctrl Pts',(-36.7462914774195,-38.9953874843817,
3.19000042450751));
#22676=CARTESIAN_POINT('Ctrl Pts',(-39.2958016196254,-35.7474915197397,
3.03300029715526));
#22677=CARTESIAN_POINT('Ctrl Pts',(-37.9932252344219,-31.8293127090433,
2.876000169803));
#22678=CARTESIAN_POINT('Ctrl Pts',(-34.0065950719303,-30.754319669156,2.71900004245075));
#22679=CARTESIAN_POINT('Ctrl Pts',(-30.910760626402,-33.4864687946697,2.5619999150985));
#22680=CARTESIAN_POINT('Ctrl Pts',(-31.4817863824102,-37.5758161108508,
2.40499978774625));
#22681=CARTESIAN_POINT('Ctrl Pts',(-35.2076279914714,-39.3554039283154,
2.24799966039399));
#22682=CARTESIAN_POINT('Ctrl Pts',(-38.7472876895237,-37.2294602281335,
2.09099953304174));
#22683=CARTESIAN_POINT('Ctrl Pts',(-38.9267183633859,-33.1043362013228,
1.93399940568948));
#22684=CARTESIAN_POINT('Ctrl Pts',(-35.5850234188216,-30.6790760206131,
1.77699927833723));
#22685=CARTESIAN_POINT('Ctrl Pts',(-31.7187315376645,-32.128421904617,1.61999915098498));
#22686=CARTESIAN_POINT('Ctrl Pts',(-30.7947862267274,-36.1527553723333,
1.46299902363272));
#22687=CARTESIAN_POINT('Ctrl Pts',(-33.6416931030839,-39.1433698920001,
1.30599889628047));
#22688=CARTESIAN_POINT('Ctrl Pts',(-37.7066135461226,-38.4186496421557,
1.14899876892822));
#22689=CARTESIAN_POINT('Ctrl Pts',(-39.3444740755065,-34.628262991515,0.991998641575964));
#22690=CARTESIAN_POINT('Ctrl Pts',(-37.0866303819407,-31.1714793259802,
0.83499851422371));
#22691=CARTESIAN_POINT('Ctrl Pts',(-32.9576300903856,-31.1472373508815,
0.677998386871457));
#22692=CARTESIAN_POINT('Ctrl Pts',(-30.6601534973185,-34.5788714630532,
0.520998259519203));
#22693=CARTESIAN_POINT('Ctrl Pts',(-32.2540356527884,-38.3859852262338,
0.363998132166951));
#22694=CARTESIAN_POINT('Ctrl Pts',(-36.3106933795422,-39.1612020385825,
0.206998004814695));
#22695=CARTESIAN_POINT('Ctrl Pts',(-39.1911999412976,-36.1960803455747,
0.049997877462444));
#22696=CARTESIAN_POINT('Ctrl Pts',(-38.6056283266121,-33.5191597390956,
-0.0546688741057268));
#22697=CARTESIAN_POINT('Ctrl Pts',(-37.8143974874483,-32.5937287191406,
-0.107002249889811));
#22698=CARTESIAN_POINT('Ctrl Pts',(-35.9084720925035,-38.3981590173419,
8.32100674966943));
#22699=CARTESIAN_POINT('Ctrl Pts',(-37.0258557525633,-38.0994349533404,
8.26867337388535));
#22700=CARTESIAN_POINT('Ctrl Pts',(-38.9246974524274,-36.318886728109,8.16400662231718));
#22701=CARTESIAN_POINT('Ctrl Pts',(-38.265183474209,-32.4476566833857,8.00700649496493));
#22702=CARTESIAN_POINT('Ctrl Pts',(-34.6722754638272,-30.8716910088818,
7.85000636761267));
#22703=CARTESIAN_POINT('Ctrl Pts',(-31.3759278684536,-32.9944537546442,
7.69300624026043));
#22704=CARTESIAN_POINT('Ctrl Pts',(-31.3279886718125,-36.9171723421199,
7.53600611290816));
#22705=CARTESIAN_POINT('Ctrl Pts',(-34.5734382288568,-39.119968635311,7.37900598555592));
#22706=CARTESIAN_POINT('Ctrl Pts',(-38.2010617370167,-37.6287344130329,
7.22200585820366));
#22707=CARTESIAN_POINT('Ctrl Pts',(-38.9584253279276,-33.7800977775671,
7.0650057308514));
#22708=CARTESIAN_POINT('Ctrl Pts',(-36.1661501156877,-31.0254539991911,
6.90800560349916));
#22709=CARTESIAN_POINT('Ctrl Pts',(-32.328217032531,-31.834776677721,6.75100547614689));
#22710=CARTESIAN_POINT('Ctrl Pts',(-30.8860774508557,-35.482408840697,6.59400534879465));
#22711=CARTESIAN_POINT('Ctrl Pts',(-33.1329415727439,-38.6974487700223,
6.43700522144238));
#22712=CARTESIAN_POINT('Ctrl Pts',(-37.0540099906223,-38.5969566726394,
6.28000509409015));
#22713=CARTESIAN_POINT('Ctrl Pts',(-39.1332303805976,-35.271036161565,6.12300496673788));
#22714=CARTESIAN_POINT('Ctrl Pts',(-37.5061422267118,-31.7020763427115,
5.96600483938563));
#22715=CARTESIAN_POINT('Ctrl Pts',(-33.6317728954962,-31.0903956020826,
5.80900471203338));
#22716=CARTESIAN_POINT('Ctrl Pts',(-30.9843056371378,-33.9844949816193,
5.65200458468112));
#22717=CARTESIAN_POINT('Ctrl Pts',(-31.9377501866703,-37.7892072799639,
5.49500445732888));
#22718=CARTESIAN_POINT('Ctrl Pts',(-35.6371434483029,-39.0928107380382,
5.33800432997661));
#22719=CARTESIAN_POINT('Ctrl Pts',(-38.7652041038025,-36.7263514999179,
5.18100420262437));
#22720=CARTESIAN_POINT('Ctrl Pts',(-38.5169700996031,-32.8118563311761,
5.02400407527211));
#22721=CARTESIAN_POINT('Ctrl Pts',(-35.1150352757837,-30.85949057183,4.86700394791986));
#22722=CARTESIAN_POINT('Ctrl Pts',(-31.6099472121153,-32.6199593442133,
4.7100038205676));
#22723=CARTESIAN_POINT('Ctrl Pts',(-31.1447520082465,-36.5146334030964,
4.55300369321535));
#22724=CARTESIAN_POINT('Ctrl Pts',(-34.1365946630648,-39.0511211600269,
4.3960035658631));
#22725=CARTESIAN_POINT('Ctrl Pts',(-37.902661167183,-37.9549297073231,4.23900343851084));
#22726=CARTESIAN_POINT('Ctrl Pts',(-39.0658835555688,-34.2090244382739,
4.08200331115859));
#22727=CARTESIAN_POINT('Ctrl Pts',(-36.5831891534466,-31.1723945431281,
3.92500318380633));
#22728=CARTESIAN_POINT('Ctrl Pts',(-32.6808338490201,-31.5680151824572,
3.76800305645409));
#22729=CARTESIAN_POINT('Ctrl Pts',(-30.8580970811077,-35.041129530926,3.61100292910183));
#22730=CARTESIAN_POINT('Ctrl Pts',(-32.74944439652,-38.4773626378456,3.45400280174958));
#22731=CARTESIAN_POINT('Ctrl Pts',(-36.6588865117225,-38.79541130026,3.29700267439732));
#22732=CARTESIAN_POINT('Ctrl Pts',(-39.0807891786557,-35.710078251974,3.14000254704507));
#22733=CARTESIAN_POINT('Ctrl Pts',(-37.8434090368849,-31.988011195227,2.98300241969281));
#22734=CARTESIAN_POINT('Ctrl Pts',(-34.0563167391228,-30.9668234513003,
2.82600229234056));
#22735=CARTESIAN_POINT('Ctrl Pts',(-31.1154342629614,-33.5622236985868,
2.66900216498831));
#22736=CARTESIAN_POINT('Ctrl Pts',(-31.6578791736403,-37.446891975492,2.51200203763606));
#22737=CARTESIAN_POINT('Ctrl Pts',(-35.1972358446236,-39.1374082867668,
2.3550019102838));
#22738=CARTESIAN_POINT('Ctrl Pts',(-38.5597293373271,-37.1178718150406,
2.19800178293155));
#22739=CARTESIAN_POINT('Ctrl Pts',(-38.7301791897763,-33.1992175149173,
2.04100165557929));
#22740=CARTESIAN_POINT('Ctrl Pts',(-35.5557419658023,-30.8953458799586,
1.88400152822704));
#22741=CARTESIAN_POINT('Ctrl Pts',(-31.8829648063379,-32.2721494484828,
1.72700140087479));
#22742=CARTESIAN_POINT('Ctrl Pts',(-31.0052645863564,-36.0950579346039,
1.57000127352254));
#22743=CARTESIAN_POINT('Ctrl Pts',(-33.7096787568343,-38.9359869276078,
1.41300114617028));
#22744=CARTESIAN_POINT('Ctrl Pts',(-37.5711427686419,-38.247540203344,1.25600101881803));
#22745=CARTESIAN_POINT('Ctrl Pts',(-39.1270254923511,-34.6468690838513,
1.09900089146578));
#22746=CARTESIAN_POINT('Ctrl Pts',(-36.9821908543394,-31.3631035321966,
0.94200076411352));
#22747=CARTESIAN_POINT('Ctrl Pts',(-33.0598543033527,-31.3400749106699,
0.785000636761268));
#22748=CARTESIAN_POINT('Ctrl Pts',(-30.8773704622995,-34.599949688425,0.628000509409013));
#22749=CARTESIAN_POINT('Ctrl Pts',(-32.3914760072062,-38.2165106989991,
0.471000382056762));
#22750=CARTESIAN_POINT('Ctrl Pts',(-36.2450908662393,-38.9529265438306,
0.314000254704506));
#22751=CARTESIAN_POINT('Ctrl Pts',(-38.9814229986536,-36.1362144165888,
0.157000127352255));
#22752=CARTESIAN_POINT('Ctrl Pts',(-38.4251602751564,-33.5932784036374,
0.0523333757840841));
#22753=CARTESIAN_POINT('Ctrl Pts',(-37.6735319337713,-32.7141668369925,
0.));
#22754=CARTESIAN_POINT('Ctrl Pts',(-37.6735319337713,-32.7141668369925,
0.));
#22755=CARTESIAN_POINT('Ctrl Pts',(-37.7506744675535,-32.7912795750214,
1.11409720010452E-16));
#22756=CARTESIAN_POINT('Ctrl Pts',(-37.8237046409441,-32.8720144826054,
2.54111086902063E-16));
#22757=CARTESIAN_POINT('Ctrl Pts',(-37.8926301480271,-32.9559530569886,
5.55111512312578E-17));
#22758=CARTESIAN_POINT('Ctrl Pts',(-37.9633155600031,-33.0420348714294,
-1.48159722809431E-16));
#22759=CARTESIAN_POINT('Ctrl Pts',(-38.0296843928246,-33.1314864952968,
-2.01877327443104E-15));
#22760=CARTESIAN_POINT('Ctrl Pts',(-38.0917150717573,-33.2239026806474,
-1.83186799063151E-15));
#22761=CARTESIAN_POINT('Ctrl Pts',(-38.155036796301,-33.318242325688,-1.64107264387499E-15));
#22762=CARTESIAN_POINT('Ctrl Pts',(-38.2138383235334,-33.4156718046105,
-8.85373385211783E-16));
#22763=CARTESIAN_POINT('Ctrl Pts',(-38.268059911681,-33.515799485594,-9.43689570931383E-16));
#22764=CARTESIAN_POINT('Ctrl Pts',(-38.319849146258,-33.6114354884346,-9.99389721462685E-16));
#22765=CARTESIAN_POINT('Ctrl Pts',(-38.3674601237765,-33.7095338759835,
-7.11957983305256E-16));
#22766=CARTESIAN_POINT('Ctrl Pts',(-38.4108052730721,-33.809777999414,-7.21644966006352E-16));
#22767=CARTESIAN_POINT('Ctrl Pts',(-38.4178427440334,-33.8260535254913,
-7.23217733907022E-16));
#22768=CARTESIAN_POINT('Ctrl Pts',(-38.4247676868796,-33.8423856539009,
2.30001299369943E-15));
#22769=CARTESIAN_POINT('Ctrl Pts',(-38.4315796332288,-33.8587730721181,
2.33146835171283E-15));
#22770=CARTESIAN_POINT('Ctrl Pts',(-38.4380896782009,-33.8744342097871,
2.3615296271221E-15));
#22771=CARTESIAN_POINT('Ctrl Pts',(-38.4444935030833,-33.8901386536763,
1.24943603957411E-15));
#22772=CARTESIAN_POINT('Ctrl Pts',(-38.4507888941826,-33.9058797515619,
1.16573417585641E-15));
#22773=CARTESIAN_POINT('Ctrl Pts',(-38.4941742238636,-34.0143611327099,
5.88894247237743E-16));
#22774=CARTESIAN_POINT('Ctrl Pts',(-38.5324456986686,-34.1246595013341,
-1.81750747552515E-15));
#22775=CARTESIAN_POINT('Ctrl Pts',(-38.5655747031801,-34.2363430523647,
-1.22124532708767E-15));
#22776=CARTESIAN_POINT('Ctrl Pts',(-38.5991382485882,-34.3494915152183,
-6.17162228628305E-16));
#22777=CARTESIAN_POINT('Ctrl Pts',(-38.6274239303319,-34.4640624881056,
-2.28097715513866E-15));
#22778=CARTESIAN_POINT('Ctrl Pts',(-38.6503593525615,-34.5796394751672,
-2.85882428840978E-15));
#22779=CARTESIAN_POINT('Ctrl Pts',(-38.6743343050071,-34.7004548994865,
-3.46286189462104E-15));
#22780=CARTESIAN_POINT('Ctrl Pts',(-38.6924637958468,-34.8223704157046,
7.50012201101083E-16));
#22781=CARTESIAN_POINT('Ctrl Pts',(-38.7046094044796,-34.9449336658503,
9.15933995315754E-16));
#22782=CARTESIAN_POINT('Ctrl Pts',(-38.7137186109542,-35.0368561034595,
1.04037534097676E-15));
#22783=CARTESIAN_POINT('Ctrl Pts',(-38.7194607604909,-35.1291434881023,
1.55226768069038E-15));
#22784=CARTESIAN_POINT('Ctrl Pts',(-38.7217543278029,-35.2216084347256,
1.52655665885959E-15));
#22785=CARTESIAN_POINT('Ctrl Pts',(-38.7223018974601,-35.2436836530358,
1.52041837142613E-15));
#22786=CARTESIAN_POINT('Ctrl Pts',(-38.7226527519925,-35.2657735186889,
2.89381252678048E-15));
#22787=CARTESIAN_POINT('Ctrl Pts',(-38.722805679631,-35.2878464184275,2.85882428840978E-15));
#22788=CARTESIAN_POINT('Ctrl Pts',(-38.7236405005601,-35.4083407832928,
2.66782602310891E-15));
#22789=CARTESIAN_POINT('Ctrl Pts',(-38.7185871650491,-35.5284803305467,
-1.0113839359997E-15));
#22790=CARTESIAN_POINT('Ctrl Pts',(-38.7075767134548,-35.6478390239293,
-6.10622663543836E-16));
#22791=CARTESIAN_POINT('Ctrl Pts',(-38.696636914708,-35.766431805807,-2.12433031749896E-16));
#22792=CARTESIAN_POINT('Ctrl Pts',(-38.6798164549903,-35.8842545994116,
4.47017550934916E-16));
#22793=CARTESIAN_POINT('Ctrl Pts',(-38.6569982586142,-36.0009023628565,
1.11022302462516E-15));
#22794=CARTESIAN_POINT('Ctrl Pts',(-38.6541246129484,-36.0155925835174,
1.19374485534308E-15));
#22795=CARTESIAN_POINT('Ctrl Pts',(-38.6511557754508,-36.0302641749016,
1.91345521755541E-15));
#22796=CARTESIAN_POINT('Ctrl Pts',(-38.6480914530901,-36.044916331709,1.97064586870965E-15));
#22797=CARTESIAN_POINT('Ctrl Pts',(-38.6241809707793,-36.1592450787926,
2.44399783547239E-15));
#22798=CARTESIAN_POINT('Ctrl Pts',(-38.594461283178,-36.2723911010901,-8.48644965904397E-16));
#22799=CARTESIAN_POINT('Ctrl Pts',(-38.5592385353076,-36.3840879064664,
-8.60422844084496E-16));
#22800=CARTESIAN_POINT('Ctrl Pts',(-38.5372732895732,-36.4537431130068,
-8.67767642662035E-16));
#22801=CARTESIAN_POINT('Ctrl Pts',(-38.5131668858195,-36.5228346461715,
9.22437028861002E-17));
#22802=CARTESIAN_POINT('Ctrl Pts',(-38.4869837165243,-36.5912956919754,
8.32667268468867E-17));
#22803=CARTESIAN_POINT('Ctrl Pts',(-38.4780341824549,-36.6146960089858,
8.01983529614736E-17));
#22804=CARTESIAN_POINT('Ctrl Pts',(-38.4688419572729,-36.6380226459113,
-1.61456985271483E-15));
#22805=CARTESIAN_POINT('Ctrl Pts',(-38.4594094252689,-36.6612728659742,
-1.77635683940025E-15));
#22806=CARTESIAN_POINT('Ctrl Pts',(-38.4526602969819,-36.6779087722017,
-1.89211802927477E-15));
#22807=CARTESIAN_POINT('Ctrl Pts',(-38.4457875924452,-36.6945066762169,
2.33562128204704E-15));
#22808=CARTESIAN_POINT('Ctrl Pts',(-38.4387992548886,-36.7110492733397,
2.24820162486594E-15));
#22809=CARTESIAN_POINT('Ctrl Pts',(-38.3928779298073,-36.8197529491441,
1.67375506108868E-15));
#22810=CARTESIAN_POINT('Ctrl Pts',(-38.341903576542,-36.9262302239648,1.3366443388947E-15));
#22811=CARTESIAN_POINT('Ctrl Pts',(-38.2862346344182,-37.0302267509451,
1.30451205393456E-15));
#22812=CARTESIAN_POINT('Ctrl Pts',(-38.2286504882323,-37.1378011179799,
1.2712743072873E-15));
#22813=CARTESIAN_POINT('Ctrl Pts',(-38.1660430056126,-37.2427217973211,
4.33181580130382E-15));
#22814=CARTESIAN_POINT('Ctrl Pts',(-38.098753525921,-37.3446999432836,3.3584246494911E-15));
#22815=CARTESIAN_POINT('Ctrl Pts',(-38.030830880622,-37.4476376605642,2.37587429771653E-15));
#22816=CARTESIAN_POINT('Ctrl Pts',(-37.9581372777995,-37.5475779522675,
-1.61807423508707E-16));
#22817=CARTESIAN_POINT('Ctrl Pts',(-37.8809732699071,-37.6442054678576,
-4.30211422042248E-16));
#22818=CARTESIAN_POINT('Ctrl Pts',(-37.826560213076,-37.7123434332233,-6.19479481397997E-16));
#22819=CARTESIAN_POINT('Ctrl Pts',(-37.769923167717,-37.7788337520814,-1.16007728999665E-15));
#22820=CARTESIAN_POINT('Ctrl Pts',(-37.7111544669349,-37.8435573649047,
-1.58206781009085E-15));
#22821=CARTESIAN_POINT('Ctrl Pts',(-37.6849217834628,-37.8724481524459,
-1.77043242585642E-15));
#22822=CARTESIAN_POINT('Ctrl Pts',(-37.6582642395734,-37.9009868195143,
-1.55320898075906E-15));
#22823=CARTESIAN_POINT('Ctrl Pts',(-37.6311894369306,-37.9291622039588,
-1.76247905159244E-15));
#22824=CARTESIAN_POINT('Ctrl Pts',(-37.6195672281553,-37.9412568516894,
-1.85231093276087E-15));
#22825=CARTESIAN_POINT('Ctrl Pts',(-37.6078695516101,-37.9532830190668,
-1.32384934798458E-15));
#22826=CARTESIAN_POINT('Ctrl Pts',(-37.5961035133295,-37.9652334405448,
-1.346145417358E-15));
#22827=CARTESIAN_POINT('Ctrl Pts',(-37.5076612499423,-38.0550616646887,
-1.51373919811968E-15));
#22828=CARTESIAN_POINT('Ctrl Pts',(-37.4152596553304,-38.1407172584711,
9.39449970766038E-16));
#22829=CARTESIAN_POINT('Ctrl Pts',(-37.3192274679083,-38.221882071393,-9.29811783123569E-16));
#22830=CARTESIAN_POINT('Ctrl Pts',(-37.2371876089162,-38.2912208002711,
-2.52671355975721E-15));
#22831=CARTESIAN_POINT('Ctrl Pts',(-37.1524970590086,-38.3572819982496,
-3.43309726072543E-16));
#22832=CARTESIAN_POINT('Ctrl Pts',(-37.0653365594432,-38.419849736978,-1.11022302462516E-16));
#22833=CARTESIAN_POINT('Ctrl Pts',(-37.0262256852631,-38.4479252869043,
-6.78971724635936E-18));
#22834=CARTESIAN_POINT('Ctrl Pts',(-36.9866172085179,-38.4752971710175,
-3.75915299087743E-16));
#22835=CARTESIAN_POINT('Ctrl Pts',(-36.9465262167991,-38.5019445229708,
-5.06539254985228E-16));
#22836=CARTESIAN_POINT('Ctrl Pts',(-36.9192926653871,-38.5200458968282,
-5.95271263500483E-16));
#22837=CARTESIAN_POINT('Ctrl Pts',(-36.8918308185162,-38.5378163160328,
-1.49578843933597E-15));
#22838=CARTESIAN_POINT('Ctrl Pts',(-36.8641753660581,-38.555230466303,-1.48492329543615E-15));
#22839=CARTESIAN_POINT('Ctrl Pts',(-36.7573710739483,-38.6224832438564,
-1.44296252821847E-15));
#22840=CARTESIAN_POINT('Ctrl Pts',(-36.6476200524945,-38.6844692154967,
-2.67652767243929E-15));
#22841=CARTESIAN_POINT('Ctrl Pts',(-36.5352242775472,-38.7408547238633,
-3.18495230189342E-15));
#22842=CARTESIAN_POINT('Ctrl Pts',(-36.4331305324386,-38.792072020258,-3.64677548475584E-15));
#22843=CARTESIAN_POINT('Ctrl Pts',(-36.3288538528326,-38.8386685011131,
8.48923205726707E-17));
#22844=CARTESIAN_POINT('Ctrl Pts',(-36.2225972039516,-38.8803649981066,
1.52308721190764E-15));
#22845=CARTESIAN_POINT('Ctrl Pts',(-36.1671666977136,-38.9021166528128,
2.30316661476457E-15));
#22846=CARTESIAN_POINT('Ctrl Pts',(-36.1111970366882,-38.922534339231,-1.9802954995054E-18));
#22847=CARTESIAN_POINT('Ctrl Pts',(-36.0547323436802,-38.9416301693299,
1.11022302462516E-16));
#22848=CARTESIAN_POINT('Ctrl Pts',(-38.5153122961063,-34.9971887940747,
7.11258330249198));
#22849=CARTESIAN_POINT('Ctrl Pts',(-38.5180434423612,-34.646197163443,7.09672411194512));
#22850=CARTESIAN_POINT('Ctrl Pts',(-38.4695960103246,-34.2959413770096,
7.08086492139826));
#22851=CARTESIAN_POINT('Ctrl Pts',(-38.3668188607358,-33.9624299204154,
7.0650057308514));
#22852=CARTESIAN_POINT('Ctrl Pts',(-38.0276669238477,-32.8618831847751,
7.01267235506732));
#22853=CARTESIAN_POINT('Ctrl Pts',(-37.0969085197677,-31.9436685919831,
6.96033897928324));
#22854=CARTESIAN_POINT('Ctrl Pts',(-35.9918738038683,-31.6194484086754,
6.90800560349915));
#22855=CARTESIAN_POINT('Ctrl Pts',(-34.8868390879688,-31.2952282253677,
6.85567222771507));
#22856=CARTESIAN_POINT('Ctrl Pts',(-33.6075280602499,-31.5650024515443,
6.80333885193098));
#22857=CARTESIAN_POINT('Ctrl Pts',(-32.7275159494446,-32.307828258462,6.75100547614689));
#22858=CARTESIAN_POINT('Ctrl Pts',(-31.8475038386392,-33.0506540653796,
6.69867210036281));
#22859=CARTESIAN_POINT('Ctrl Pts',(-31.3667906447475,-34.2665314530383,
6.64633872457873));
#22860=CARTESIAN_POINT('Ctrl Pts',(-31.5009114014496,-35.4103101350885,
6.59400534879465));
#22861=CARTESIAN_POINT('Ctrl Pts',(-31.6350321581518,-36.5540888171387,
6.54167197301056));
#22862=CARTESIAN_POINT('Ctrl Pts',(-32.3839868654478,-37.6257687935805,
6.48933859722647));
#22863=CARTESIAN_POINT('Ctrl Pts',(-33.4119756220756,-38.1448600989042,
6.43700522144239));
#22864=CARTESIAN_POINT('Ctrl Pts',(-34.4399643787034,-38.663951404228,6.3846718456583));
#22865=CARTESIAN_POINT('Ctrl Pts',(-35.7469871846628,-38.6304540384337,
6.33233846987422));
#22866=CARTESIAN_POINT('Ctrl Pts',(-36.7470353193051,-38.0593852703575,
6.28000509409014));
#22867=CARTESIAN_POINT('Ctrl Pts',(-37.7470834539474,-37.4883165022812,
6.22767171830606));
#22868=CARTESIAN_POINT('Ctrl Pts',(-38.4401569172725,-36.3796763319231,
6.17533834252197));
#22869=CARTESIAN_POINT('Ctrl Pts',(-38.5155122899541,-35.2305296102685,
6.12300496673788));
#22870=CARTESIAN_POINT('Ctrl Pts',(-38.5205143775731,-35.1542492816832,
6.11953107865591));
#22871=CARTESIAN_POINT('Ctrl Pts',(-38.5227946134492,-35.0777904690468,
6.11605719057395));
#22872=CARTESIAN_POINT('Ctrl Pts',(-38.522424122767,-35.0013091826171,6.11258330249198));
#22873=CARTESIAN_POINT('Origin',(35.,35.,10.2084234471775));
#22874=CARTESIAN_POINT('Ctrl Pts',(30.9215901961247,35.0020443570103,7.70842344717745));
#22875=CARTESIAN_POINT('Ctrl Pts',(30.9207461022984,35.1331126499304,7.70328437820511));
#22876=CARTESIAN_POINT('Ctrl Pts',(30.985475579174,36.5980980633283,7.64581193344868));
#22877=CARTESIAN_POINT('Ctrl Pts',(32.753181262015,39.238437809064,7.53600611290817));
#22878=CARTESIAN_POINT('Ctrl Pts',(37.2955097522044,39.2117697306779,7.37900598555592));
#22879=CARTESIAN_POINT('Ctrl Pts',(39.7793716811886,35.4089491092894,7.22200585820366));
#22880=CARTESIAN_POINT('Ctrl Pts',(37.9775554192851,31.2391311721338,7.06500573085141));
#22881=CARTESIAN_POINT('Ctrl Pts',(33.5057216363881,30.441863683446,6.90800560349916));
#22882=CARTESIAN_POINT('Ctrl Pts',(31.1346462527125,32.9326274967327,6.7891448422745));
#22883=CARTESIAN_POINT('Ctrl Pts',(30.9248234084473,34.6330160680086,6.72261745683393));
#22884=CARTESIAN_POINT('Ctrl Pts',(30.9278854598697,34.9965452008231,6.70842344717745));
#22885=CARTESIAN_POINT('Ctrl Pts',(30.9308749498806,34.995920959377,7.79157655282255));
#22886=CARTESIAN_POINT('Ctrl Pts',(30.9370382260235,35.8984227922016,7.75638428364686));
#22887=CARTESIAN_POINT('Ctrl Pts',(31.6729751170447,38.1550462153353,7.66885863868709));
#22888=CARTESIAN_POINT('Ctrl Pts',(35.3795268052061,39.7808547962683,7.52899961794324));
#22889=CARTESIAN_POINT('Ctrl Pts',(39.1969168896572,37.3225573472918,7.37199949059099));
#22890=CARTESIAN_POINT('Ctrl Pts',(39.2524338890068,32.7797860374403,7.21499936323873));
#22891=CARTESIAN_POINT('Ctrl Pts',(35.4939868648458,30.2288021766129,7.05799923588648));
#22892=CARTESIAN_POINT('Ctrl Pts',(31.7173195455156,31.7813045011721,6.91685829908108));
#22893=CARTESIAN_POINT('Ctrl Pts',(30.9363083182476,34.0684206807159,6.82805073805977));
#22894=CARTESIAN_POINT('Ctrl Pts',(30.9290341434093,35.0032555560525,6.79157655282255));
#22895=CARTESIAN_POINT('Ctrl Pts',(37.6735319337713,37.2858331630076,8.));
#22896=CARTESIAN_POINT('Ctrl Pts',(38.4251602751564,36.4067215963626,7.94766662421592));
#22897=CARTESIAN_POINT('Ctrl Pts',(38.981419710079,33.8637820915388,7.84299987264775));
#22898=CARTESIAN_POINT('Ctrl Pts',(36.2450923914777,31.0470745569746,7.68599974529549));
#22899=CARTESIAN_POINT('Ctrl Pts',(32.3914750767338,31.7834880469926,7.52899961794325));
#22900=CARTESIAN_POINT('Ctrl Pts',(30.877370367455,35.4000509161799,7.37199949059098));
#22901=CARTESIAN_POINT('Ctrl Pts',(33.0598539558457,38.6599251241887,7.21499936323874));
#22902=CARTESIAN_POINT('Ctrl Pts',(36.9821911263972,38.6368970240971,7.05799923588648));
#22903=CARTESIAN_POINT('Ctrl Pts',(39.1270258717517,35.3531308437279,6.90099910853422));
#22904=CARTESIAN_POINT('Ctrl Pts',(37.5711430434112,31.75245953062,6.74399898118198));
#22905=CARTESIAN_POINT('Ctrl Pts',(33.7096786193679,31.0640126442915,6.58699885382972));
#22906=CARTESIAN_POINT('Ctrl Pts',(31.0052641890983,33.9049419734146,6.42999872647747));
#22907=CARTESIAN_POINT('Ctrl Pts',(31.882964491631,37.7278508156672,6.27299859912521));
#22908=CARTESIAN_POINT('Ctrl Pts',(35.5557420224402,39.1046545373095,6.11599847177296));
#22909=CARTESIAN_POINT('Ctrl Pts',(38.7301795638466,36.8007826630852,5.9589983444207));
#22910=CARTESIAN_POINT('Ctrl Pts',(38.559729694875,32.8821279738221,5.80199821706846));
#22911=CARTESIAN_POINT('Ctrl Pts',(35.1972358643355,30.8625912971014,5.64499808971619));
#22912=CARTESIAN_POINT('Ctrl Pts',(31.6578788381682,32.5531077792767,5.48799796236396));
#22913=CARTESIAN_POINT('Ctrl Pts',(31.1154338729727,36.437776445535,5.33099783501168));
#22914=CARTESIAN_POINT('Ctrl Pts',(34.0563166443959,39.033176953701,5.17399770765944));
#22915=CARTESIAN_POINT('Ctrl Pts',(37.843409322329,38.0119891070858,5.01699758030718));
#22916=CARTESIAN_POINT('Ctrl Pts',(39.0807895883257,34.2899216767724,4.85999745295493));
#22917=CARTESIAN_POINT('Ctrl Pts',(36.6588866782563,31.2045883187048,4.70299732560268));
#22918=CARTESIAN_POINT('Ctrl Pts',(32.7494441705885,31.5226370130723,4.54599719825042));
#22919=CARTESIAN_POINT('Ctrl Pts',(30.8580966653042,34.9588704649406,4.38899707089817));
#22920=CARTESIAN_POINT('Ctrl Pts',(32.6808336162004,38.4319851620801,4.23199694354592));
#22921=CARTESIAN_POINT('Ctrl Pts',(36.5831893123819,38.8276058411217,4.07499681619366));
#22922=CARTESIAN_POINT('Ctrl Pts',(39.0658839637408,35.7909756411325,3.91799668884141));
#22923=CARTESIAN_POINT('Ctrl Pts',(37.9026614585792,32.0450699960324,3.76099656148916));
#22924=CARTESIAN_POINT('Ctrl Pts',(34.1365945763887,30.9488784332844,3.6039964341369));
#22925=CARTESIAN_POINT('Ctrl Pts',(31.1447516212191,33.4853664448484,3.44699630678465));
#22926=CARTESIAN_POINT('Ctrl Pts',(31.6099468717921,37.3800408947213,3.2899961794324));
#22927=CARTESIAN_POINT('Ctrl Pts',(35.1150352873275,39.1405098438263,3.13299605208014));
#22928=CARTESIAN_POINT('Ctrl Pts',(38.5169704526781,37.1881438885041,2.97599592472789));
#22929=CARTESIAN_POINT('Ctrl Pts',(38.7652044817734,33.2736483267483,2.81899579737564));
#22930=CARTESIAN_POINT('Ctrl Pts',(35.6371435122955,30.9071888511377,2.66199567002338));
#22931=CARTESIAN_POINT('Ctrl Pts',(31.9377498791963,32.2107924399309,2.50499554267113));
#22932=CARTESIAN_POINT('Ctrl Pts',(30.9843052341107,36.0155051205153,2.34799541531888));
#22933=CARTESIAN_POINT('Ctrl Pts',(33.6317727579422,38.9096047900383,2.19099528796662));
#22934=CARTESIAN_POINT('Ctrl Pts',(37.5061424786706,38.297923989058,2.03399516061437));
#22935=CARTESIAN_POINT('Ctrl Pts',(39.1332307948504,34.7289638099038,1.87699503326212));
#22936=CARTESIAN_POINT('Ctrl Pts',(37.0540101980664,31.4030429687795,1.71999490590986));
#22937=CARTESIAN_POINT('Ctrl Pts',(33.1329413830615,31.3025508540242,1.56299477855761));
#22938=CARTESIAN_POINT('Ctrl Pts',(30.8860770418796,34.5175911198794,1.40599465120536));
#22939=CARTESIAN_POINT('Ctrl Pts',(32.3282167572518,38.1652236231046,1.2489945238531));
#22940=CARTESIAN_POINT('Ctrl Pts',(36.1661502448953,38.9745464314742,1.09199439650085));
#22941=CARTESIAN_POINT('Ctrl Pts',(38.9584257050592,36.219902286033,0.934994269148596));
#22942=CARTESIAN_POINT('Ctrl Pts',(38.2010620907038,32.3712654317411,0.777994141796343));
#22943=CARTESIAN_POINT('Ctrl Pts',(34.5734381379524,30.8800307521414,0.620994014444089));
#22944=CARTESIAN_POINT('Ctrl Pts',(31.3279883656859,33.0828278259953,0.463993887091835));
#22945=CARTESIAN_POINT('Ctrl Pts',(31.3759274478189,37.0055458008236,0.306993759739581));
#22946=CARTESIAN_POINT('Ctrl Pts',(34.6722754073454,39.1283105516069,0.149993632387328));
#22947=CARTESIAN_POINT('Ctrl Pts',(38.2651841076192,37.5523415454803,-0.007006494964925));
#22948=CARTESIAN_POINT('Ctrl Pts',(38.9246967202481,33.681118012335,-0.164006622317179));
#22949=CARTESIAN_POINT('Ctrl Pts',(37.0258557525633,31.9005650466596,-0.268673373885348));
#22950=CARTESIAN_POINT('Ctrl Pts',(35.9084720925035,31.6018409826581,-0.321006749669432));
#22951=CARTESIAN_POINT('Ctrl Pts',(37.8143974874483,37.4062712808594,8.10700224988981));
#22952=CARTESIAN_POINT('Ctrl Pts',(38.6056283266121,36.4808402609044,8.05466887410573));
#22953=CARTESIAN_POINT('Ctrl Pts',(39.1911964794515,33.80391597857,7.95000212253756));
#22954=CARTESIAN_POINT('Ctrl Pts',(36.3106949851439,30.8387991202229,7.7930019951853));
#22955=CARTESIAN_POINT('Ctrl Pts',(32.2540346732905,31.6140134536857,7.63600186783305));
#22956=CARTESIAN_POINT('Ctrl Pts',(30.6601533974768,35.4211291734076,7.4790017404808));
#22957=CARTESIAN_POINT('Ctrl Pts',(32.9576297245688,38.8527626858139,7.32200161312855));
#22958=CARTESIAN_POINT('Ctrl Pts',(37.0866306683329,38.828521259624,7.16500148577629));
#22959=CARTESIAN_POINT('Ctrl Pts',(39.3444744748973,35.3717369322484,7.00800135842404));
#22960=CARTESIAN_POINT('Ctrl Pts',(37.7066138353691,31.5813500777913,6.85100123107178));
#22961=CARTESIAN_POINT('Ctrl Pts',(33.6416929583746,30.856629657343,6.69400110371953));
#22962=CARTESIAN_POINT('Ctrl Pts',(30.7947858085381,33.8472445308389,6.53700097636727));
#22963=CARTESIAN_POINT('Ctrl Pts',(31.7187312063761,37.8715783734507,6.38000084901503));
#22964=CARTESIAN_POINT('Ctrl Pts',(35.5850234784437,39.3209244186404,6.22300072166276));
#22965=CARTESIAN_POINT('Ctrl Pts',(38.9267187571656,36.8956639860585,6.06600059431053));
#22966=CARTESIAN_POINT('Ctrl Pts',(38.7472880659103,32.7705395496047,5.90900046695826));
#22967=CARTESIAN_POINT('Ctrl Pts',(35.2076280122218,30.6445956336272,5.75200033960601));
#22968=CARTESIAN_POINT('Ctrl Pts',(31.4817860292625,32.4241836309969,5.59500021225375));
#22969=CARTESIAN_POINT('Ctrl Pts',(30.9107602158652,36.5135313570458,5.4380000849015));
#22970=CARTESIAN_POINT('Ctrl Pts',(34.0065949722125,39.2456807571843,5.28099995754925));
#22971=CARTESIAN_POINT('Ctrl Pts',(37.9932255349056,38.1706876091981,5.12399983019699));
#22972=CARTESIAN_POINT('Ctrl Pts',(39.2958020508805,34.2525084052524,4.96699970284474));
#22973=CARTESIAN_POINT('Ctrl Pts',(36.7462916527279,31.0046121145067,4.80999957549249));
#22974=CARTESIAN_POINT('Ctrl Pts',(32.6308647779182,31.3394184562628,4.65299944814024));
#22975=CARTESIAN_POINT('Ctrl Pts',(30.6398641844617,34.956703393489,4.49599932078798));
#22976=CARTESIAN_POINT('Ctrl Pts',(32.5586392064025,38.612812809568,4.33899919343573));
#22977=CARTESIAN_POINT('Ctrl Pts',(36.6666058731669,39.0292783213552,4.18199906608348));
#22978=CARTESIAN_POINT('Ctrl Pts',(39.2801110647917,35.8326513062801,4.02499893873122));
#22979=CARTESIAN_POINT('Ctrl Pts',(38.0555996031866,31.889377877368,3.86799881137897));
#22980=CARTESIAN_POINT('Ctrl Pts',(34.0911026630479,30.7354291472295,3.71099868402672));
#22981=CARTESIAN_POINT('Ctrl Pts',(30.9416226850806,33.4055620139871,3.55399855667446));
#22982=CARTESIAN_POINT('Ctrl Pts',(31.4313285785645,37.5054427177457,3.39699842932221));
#22983=CARTESIAN_POINT('Ctrl Pts',(35.1210963742505,39.3586689031172,3.23999830196995));
#22984=CARTESIAN_POINT('Ctrl Pts',(38.7022758847263,37.3034348623974,3.0829981746177));
#22985=CARTESIAN_POINT('Ctrl Pts',(38.9635891007609,33.1826886934549,2.92599804726545));
#22986=CARTESIAN_POINT('Ctrl Pts',(35.6707139262103,30.691542985346,2.76899791991319));
#22987=CARTESIAN_POINT('Ctrl Pts',(31.7764031777353,32.0638320605518,2.61199779256094));
#22988=CARTESIAN_POINT('Ctrl Pts',(30.7727225485069,36.0690110050931,2.45499766520869));
#22989=CARTESIAN_POINT('Ctrl Pts',(33.5596823199811,39.1155977076656,2.29799753785643));
#22990=CARTESIAN_POINT('Ctrl Pts',(37.6381884600154,38.4716880959441,2.14099741050418));
#22991=CARTESIAN_POINT('Ctrl Pts',(39.3510063287937,34.7146832013567,1.98399728315193));
#22992=CARTESIAN_POINT('Ctrl Pts',(37.1622338104923,31.2135231289919,1.82699715579967));
#22993=CARTESIAN_POINT('Ctrl Pts',(33.0345680505794,31.1077361916065,1.66999702844742));
#22994=CARTESIAN_POINT('Ctrl Pts',(30.6693188173153,34.4921735091382,1.51299690109517));
#22995=CARTESIAN_POINT('Ctrl Pts',(32.1874433402447,38.3319958888659,1.35599677374292));
#22996=CARTESIAN_POINT('Ctrl Pts',(36.227593460831,39.1839610551084,1.19899664639066));
#22997=CARTESIAN_POINT('Ctrl Pts',(39.1669909447667,36.2841776398386,1.04199651903841));
#22998=CARTESIAN_POINT('Ctrl Pts',(38.3697226472005,32.2327602036007,0.884996391686153));
#22999=CARTESIAN_POINT('Ctrl Pts',(34.5509630471873,30.6629539550025,0.727996264333901));
#23000=CARTESIAN_POINT('Ctrl Pts',(31.1345139786991,32.9818140634986,0.570996136981646));
#23001=CARTESIAN_POINT('Ctrl Pts',(31.1849789200754,37.1112158757118,0.413996009629392));
#23002=CARTESIAN_POINT('Ctrl Pts',(34.6550079471686,39.3458268431676,0.256995882277139));
#23003=CARTESIAN_POINT('Ctrl Pts',(38.4372231849787,37.6868217065119,0.0999957549248859));
#23004=CARTESIAN_POINT('Ctrl Pts',(39.1314848156243,33.611627523338,-0.0570043724273679));
#23005=CARTESIAN_POINT('Ctrl Pts',(37.1325959372044,31.7372591159268,-0.161671123995537));
#23006=CARTESIAN_POINT('Ctrl Pts',(35.9563385206894,31.4227955987545,-0.214004499779622));
#23007=CARTESIAN_POINT('Ctrl Pts',(37.9552630411254,37.5267093987114,8.21400449977962));
#23008=CARTESIAN_POINT('Ctrl Pts',(38.7860963780679,36.5549589254462,8.16167112399554));
#23009=CARTESIAN_POINT('Ctrl Pts',(39.4009732488241,33.744049865601,8.05700437242737));
#23010=CARTESIAN_POINT('Ctrl Pts',(36.37629757881,30.6305236834712,7.90000424507512));
#23011=CARTESIAN_POINT('Ctrl Pts',(32.1165942698471,31.4445388603786,7.74300411772287));
#23012=CARTESIAN_POINT('Ctrl Pts',(30.4429364274986,35.4422074306354,7.58600399037061));
#23013=CARTESIAN_POINT('Ctrl Pts',(32.8554054932919,39.0456002474389,7.42900386301836));
#23014=CARTESIAN_POINT('Ctrl Pts',(37.1910702102687,39.020145495151,7.2720037356661));
#23015=CARTESIAN_POINT('Ctrl Pts',(39.561923078043,35.3903430207689,7.11500360831385));
#23016=CARTESIAN_POINT('Ctrl Pts',(37.8420846273271,31.4102406249626,6.95800348096159));
#23017=CARTESIAN_POINT('Ctrl Pts',(33.5737072973814,30.6492466703945,6.80100335360934));
#23018=CARTESIAN_POINT('Ctrl Pts',(30.5843074279779,33.789547088263,6.64400322625708));
#23019=CARTESIAN_POINT('Ctrl Pts',(31.5544979211211,38.0153059312343,6.48700309890484));
#23020=CARTESIAN_POINT('Ctrl Pts',(35.6143049344472,39.5371942999712,6.33000297155258));
#23021=CARTESIAN_POINT('Ctrl Pts',(39.1232579504846,36.9905453090318,6.17300284420033));
#23022=CARTESIAN_POINT('Ctrl Pts',(38.9348464369457,32.6589511253872,6.01600271684807));
#23023=CARTESIAN_POINT('Ctrl Pts',(35.2180201601081,30.4265999701529,5.85900258949582));
#23024=CARTESIAN_POINT('Ctrl Pts',(31.3056932203567,32.2952594827172,5.70200246214357));
#23025=CARTESIAN_POINT('Ctrl Pts',(30.7060865587576,36.5892862685565,5.54500233479131));
#23026=CARTESIAN_POINT('Ctrl Pts',(33.956873300029,39.4581845606676,5.38800220743906));
#23027=CARTESIAN_POINT('Ctrl Pts',(38.1430417474823,38.3293861113103,5.2310020800868));
#23028=CARTESIAN_POINT('Ctrl Pts',(39.5108145134353,34.2150951337324,5.07400195273456));
#23029=CARTESIAN_POINT('Ctrl Pts',(36.8336966271993,30.8046359103087,4.9170018253823));
#23030=CARTESIAN_POINT('Ctrl Pts',(32.512285385248,31.1561998994534,4.76000169803005));
#23031=CARTESIAN_POINT('Ctrl Pts',(30.4216317036192,34.9545363220374,4.60300157067779));
#23032=CARTESIAN_POINT('Ctrl Pts',(32.4364447966046,38.7936404570559,4.44600144332554));
#23033=CARTESIAN_POINT('Ctrl Pts',(36.750022433952,39.2309508015887,4.28900131597329));
#23034=CARTESIAN_POINT('Ctrl Pts',(39.4943381658426,35.8743269714277,4.13200118862103));
#23035=CARTESIAN_POINT('Ctrl Pts',(38.2085377477941,31.7336857587036,3.97500106126878));
#23036=CARTESIAN_POINT('Ctrl Pts',(34.0456107497072,30.5219798611747,3.81800093391652));
#23037=CARTESIAN_POINT('Ctrl Pts',(30.738493748942,33.3257575831257,3.66100080656427));
#23038=CARTESIAN_POINT('Ctrl Pts',(31.252710285337,37.6308445407701,3.50400067921202));
#23039=CARTESIAN_POINT('Ctrl Pts',(35.1271574611734,39.5768279624082,3.34700055185977));
#23040=CARTESIAN_POINT('Ctrl Pts',(38.8875813167745,37.4187258362905,3.19000042450751));
#23041=CARTESIAN_POINT('Ctrl Pts',(39.1619737197485,33.0917290601617,3.03300029715526));
#23042=CARTESIAN_POINT('Ctrl Pts',(35.7042843401251,30.4758971195542,2.876000169803));
#23043=CARTESIAN_POINT('Ctrl Pts',(31.6150564762743,31.9168716811727,2.71900004245075));
#23044=CARTESIAN_POINT('Ctrl Pts',(30.5611398629031,36.1225168896708,2.5619999150985));
#23045=CARTESIAN_POINT('Ctrl Pts',(33.48759188202,39.3215906252928,2.40499978774624));
#23046=CARTESIAN_POINT('Ctrl Pts',(37.7702344413602,38.6454522028303,2.24799966039399));
#23047=CARTESIAN_POINT('Ctrl Pts',(39.568781862737,34.7004025928096,2.09099953304174));
#23048=CARTESIAN_POINT('Ctrl Pts',(37.2704574229183,31.0240032892043,1.93399940568949));
#23049=CARTESIAN_POINT('Ctrl Pts',(32.9361947180972,30.9129215291889,1.77699927833723));
#23050=CARTESIAN_POINT('Ctrl Pts',(30.4525605927511,34.4667558983969,1.61999915098498));
#23051=CARTESIAN_POINT('Ctrl Pts',(32.0466699232375,38.4987681546272,1.46299902363272));
#23052=CARTESIAN_POINT('Ctrl Pts',(36.2890366767668,39.3933756787425,1.30599889628047));
#23053=CARTESIAN_POINT('Ctrl Pts',(39.3755561844741,36.3484529936443,1.14899876892822));
#23054=CARTESIAN_POINT('Ctrl Pts',(38.5383832036972,32.0942549754603,0.991998641575964));
#23055=CARTESIAN_POINT('Ctrl Pts',(34.5284879564222,30.4458771578634,0.834998514223711));
#23056=CARTESIAN_POINT('Ctrl Pts',(30.9410395917123,32.8808003010019,0.677998386871457));
#23057=CARTESIAN_POINT('Ctrl Pts',(30.9940303923319,37.2168859506,0.520998259519203));
#23058=CARTESIAN_POINT('Ctrl Pts',(34.6377404869918,39.5633431347282,0.36399813216695));
#23059=CARTESIAN_POINT('Ctrl Pts',(38.6092622623382,37.8213018675437,0.206998004814697));
#23060=CARTESIAN_POINT('Ctrl Pts',(39.3382729110006,33.5421370343408,0.0499978774624429));
#23061=CARTESIAN_POINT('Ctrl Pts',(37.2393361218455,31.5739531851941,-0.0546688741057264));
#23062=CARTESIAN_POINT('Ctrl Pts',(36.0042049488753,31.243750214851,-0.107002249889811));
#23063=CARTESIAN_POINT('Ctrl Pts',(38.0961285948024,37.6471475165633,8.32100674966943));
#23064=CARTESIAN_POINT('Ctrl Pts',(38.9665644295237,36.6290775899881,8.26867337388535));
#23065=CARTESIAN_POINT('Ctrl Pts',(39.6107500181967,33.6841837526321,8.16400662231718));
#23066=CARTESIAN_POINT('Ctrl Pts',(36.441900172476,30.4222482467195,8.00700649496493));
#23067=CARTESIAN_POINT('Ctrl Pts',(31.9791538664038,31.2750642670716,7.85000636761267));
#23068=CARTESIAN_POINT('Ctrl Pts',(30.2257194575204,35.4632856878632,7.69300624026042));
#23069=CARTESIAN_POINT('Ctrl Pts',(32.753181262015,39.238437809064,7.53600611290817));
#23070=CARTESIAN_POINT('Ctrl Pts',(37.2955097522044,39.2117697306779,7.37900598555592));
#23071=CARTESIAN_POINT('Ctrl Pts',(39.7793716811886,35.4089491092894,7.22200585820366));
#23072=CARTESIAN_POINT('Ctrl Pts',(37.9775554192851,31.2391311721338,7.06500573085141));
#23073=CARTESIAN_POINT('Ctrl Pts',(33.5057216363881,30.441863683446,6.90800560349916));
#23074=CARTESIAN_POINT('Ctrl Pts',(30.3738290474178,33.7318496456872,6.75100547614689));
#23075=CARTESIAN_POINT('Ctrl Pts',(31.3902646358661,38.1590334890178,6.59400534879465));
#23076=CARTESIAN_POINT('Ctrl Pts',(35.6435863904507,39.7534641813021,6.43700522144238));
#23077=CARTESIAN_POINT('Ctrl Pts',(39.3197971438036,37.085426632005,6.28000509409014));
#23078=CARTESIAN_POINT('Ctrl Pts',(39.122404807981,32.5473627011697,6.12300496673788));
#23079=CARTESIAN_POINT('Ctrl Pts',(35.2284123079944,30.2086043066787,5.96600483938564));
#23080=CARTESIAN_POINT('Ctrl Pts',(31.1296004114509,32.1663353344374,5.80900471203338));
#23081=CARTESIAN_POINT('Ctrl Pts',(30.5014129016501,36.6650411800673,5.65200458468112));
#23082=CARTESIAN_POINT('Ctrl Pts',(33.9071516278456,39.6706883641509,5.49500445732887));
#23083=CARTESIAN_POINT('Ctrl Pts',(38.2928579600589,38.4880846134226,5.33800432997661));
#23084=CARTESIAN_POINT('Ctrl Pts',(39.72582697599,34.1776818622125,5.18100420262437));
#23085=CARTESIAN_POINT('Ctrl Pts',(36.9211016016709,30.6046597061106,5.0240040752721));
#23086=CARTESIAN_POINT('Ctrl Pts',(32.3937059925777,30.9729813426439,4.86700394791986));
#23087=CARTESIAN_POINT('Ctrl Pts',(30.2033992227766,34.9523692505858,4.7100038205676));
#23088=CARTESIAN_POINT('Ctrl Pts',(32.3142503868067,38.9744681045439,4.55300369321535));
#23089=CARTESIAN_POINT('Ctrl Pts',(36.833438994737,39.4326232818222,4.39600356586309));
#23090=CARTESIAN_POINT('Ctrl Pts',(39.7085652668935,35.9160026365752,4.23900343851085));
#23091=CARTESIAN_POINT('Ctrl Pts',(38.3614758924016,31.5779936400392,4.08200331115859));
#23092=CARTESIAN_POINT('Ctrl Pts',(34.0001188363665,30.3085305751198,3.92500318380634));
#23093=CARTESIAN_POINT('Ctrl Pts',(30.5353648128034,33.2459531522644,3.76800305645408));
#23094=CARTESIAN_POINT('Ctrl Pts',(31.0740919921095,37.7562463637945,3.61100292910183));
#23095=CARTESIAN_POINT('Ctrl Pts',(35.1332185480963,39.7949870216991,3.45400280174957));
#23096=CARTESIAN_POINT('Ctrl Pts',(39.0728867488228,37.5340168101838,3.29700267439732));
#23097=CARTESIAN_POINT('Ctrl Pts',(39.360358338736,33.0007694268683,3.14000254704507));
#23098=CARTESIAN_POINT('Ctrl Pts',(35.7378547540399,30.2602512537625,2.98300241969282));
#23099=CARTESIAN_POINT('Ctrl Pts',(31.4537097748133,31.7699113017935,2.82600229234056));
#23100=CARTESIAN_POINT('Ctrl Pts',(30.3495571772993,36.1760227742485,2.66900216498831));
#23101=CARTESIAN_POINT('Ctrl Pts',(33.415501444059,39.52758354292,2.51200203763605));
#23102=CARTESIAN_POINT('Ctrl Pts',(37.902280422705,38.8192163097165,2.3550019102838));
#23103=CARTESIAN_POINT('Ctrl Pts',(39.7865573966804,34.6861219842625,2.19800178293155));
#23104=CARTESIAN_POINT('Ctrl Pts',(37.3786810353442,30.8344834494167,2.0410016555793));
#23105=CARTESIAN_POINT('Ctrl Pts',(32.8378213856151,30.7181068667712,1.88400152822704));
#23106=CARTESIAN_POINT('Ctrl Pts',(30.2358023681867,34.4413382876556,1.72700140087479));
#23107=CARTESIAN_POINT('Ctrl Pts',(31.9058965062304,38.6655404203885,1.57000127352254));
#23108=CARTESIAN_POINT('Ctrl Pts',(36.3504798927025,39.6027903023767,1.41300114617028));
#23109=CARTESIAN_POINT('Ctrl Pts',(39.5841214241815,36.41272834745,1.25600101881803));
#23110=CARTESIAN_POINT('Ctrl Pts',(38.7070437601939,31.9557497473198,1.09900089146578));
#23111=CARTESIAN_POINT('Ctrl Pts',(34.5060128656572,30.2288003607244,0.942000764113522));
#23112=CARTESIAN_POINT('Ctrl Pts',(30.7475652047255,32.7797865385051,0.785000636761267));
#23113=CARTESIAN_POINT('Ctrl Pts',(30.8030818645885,37.3225560254883,0.628000509409015));
#23114=CARTESIAN_POINT('Ctrl Pts',(34.620473026815,39.7808594262888,0.47100038205676));
#23115=CARTESIAN_POINT('Ctrl Pts',(38.7813013396977,37.9557820285754,0.314000254704507));
#23116=CARTESIAN_POINT('Ctrl Pts',(39.5450610063768,33.4726465453437,0.157000127352254));
#23117=CARTESIAN_POINT('Ctrl Pts',(37.3460763064866,31.4106472544613,0.0523333757840845));
#23118=CARTESIAN_POINT('Ctrl Pts',(36.0520713770613,31.0647048309474,0.));
#23119=CARTESIAN_POINT('Ctrl Pts',(36.0520713770613,31.0647048309474,0.));
#23120=CARTESIAN_POINT('Ctrl Pts',(36.1681792227746,31.1043194052127,-1.93406836379874E-16));
#23121=CARTESIAN_POINT('Ctrl Pts',(36.2820220087194,31.1494844117486,-1.00024874895392E-15));
#23122=CARTESIAN_POINT('Ctrl Pts',(36.3933738437048,31.1998422365254,-1.16573417585641E-15));
#23123=CARTESIAN_POINT('Ctrl Pts',(36.5072229375308,31.2513294232309,-1.33493090168249E-15));
#23124=CARTESIAN_POINT('Ctrl Pts',(36.6184687230184,31.3082454542348,-1.64395861563978E-15));
#23125=CARTESIAN_POINT('Ctrl Pts',(36.7268454950609,31.3702566870239,-9.99200722162641E-16));
#23126=CARTESIAN_POINT('Ctrl Pts',(36.8407839045068,31.435450188349,-3.21355391692774E-16));
#23127=CARTESIAN_POINT('Ctrl Pts',(36.9515522547681,31.5062756815887,8.02288849704332E-16));
#23128=CARTESIAN_POINT('Ctrl Pts',(37.058802639455,31.5823916741173,9.99200722162641E-16));
#23129=CARTESIAN_POINT('Ctrl Pts',(37.1526467260561,31.6489931675798,1.17149861056366E-15));
#23130=CARTESIAN_POINT('Ctrl Pts',(37.2437970657742,31.7196462572752,8.48680262035355E-16));
#23131=CARTESIAN_POINT('Ctrl Pts',(37.3319890907744,31.7941443117117,9.99200722162641E-16));
#23132=CARTESIAN_POINT('Ctrl Pts',(37.3493641971328,31.8088215075162,1.02885543304851E-15));
#23133=CARTESIAN_POINT('Ctrl Pts',(37.3666243754182,31.8236479962496,-1.0299785826125E-15));
#23134=CARTESIAN_POINT('Ctrl Pts',(37.3837674478979,31.8386222687341,-1.0547118733939E-15));
#23135=CARTESIAN_POINT('Ctrl Pts',(37.3963017832026,31.8495708634207,-1.07279587555905E-15));
#23136=CARTESIAN_POINT('Ctrl Pts',(37.4087723034701,31.8605974704649,-2.60456824673694E-15));
#23137=CARTESIAN_POINT('Ctrl Pts',(37.4211693573137,31.8716933759855,-2.4980018054066E-15));
#23138=CARTESIAN_POINT('Ctrl Pts',(37.5137485970205,31.954555845562,-1.70218045614906E-15));
#23139=CARTESIAN_POINT('Ctrl Pts',(37.6023719888639,32.0414000295362,-2.33877871405102E-15));
#23140=CARTESIAN_POINT('Ctrl Pts',(37.6867781087441,32.1319050017937,-1.99840144432528E-15));
#23141=CARTESIAN_POINT('Ctrl Pts',(37.7709925191637,32.2222044124232,-1.65879726478403E-15));
#23142=CARTESIAN_POINT('Ctrl Pts',(37.8510093104121,32.3161487056446,-9.47721428060247E-16));
#23143=CARTESIAN_POINT('Ctrl Pts',(37.9265284067741,32.4134511741487,-1.30451205393456E-15));
#23144=CARTESIAN_POINT('Ctrl Pts',(38.0010152019123,32.5094235756611,-1.65642556372184E-15));
#23145=CARTESIAN_POINT('Ctrl Pts',(38.0711268225993,32.6086636566059,-6.10757404334397E-16));
#23146=CARTESIAN_POINT('Ctrl Pts',(38.1365292929227,32.710917134839,-5.27355936696949E-16));
#23147=CARTESIAN_POINT('Ctrl Pts',(38.1898350382321,32.7942579909372,-4.59380256721482E-16));
#23148=CARTESIAN_POINT('Ctrl Pts',(38.2400117946351,32.8796011515617,-1.29327937900734E-15));
#23149=CARTESIAN_POINT('Ctrl Pts',(38.28685279593,32.9668147810226,-1.63757896132211E-15));
#23150=CARTESIAN_POINT('Ctrl Pts',(38.298752249944,32.9889704682297,-1.72504457763057E-15));
#23151=CARTESIAN_POINT('Ctrl Pts',(38.3104363019817,33.0112468837781,3.54805112116964E-15));
#23152=CARTESIAN_POINT('Ctrl Pts',(38.3219012991264,33.0336418915139,3.66373598126302E-15));
#23153=CARTESIAN_POINT('Ctrl Pts',(38.3300587509266,33.0495761472196,3.74604683213415E-15));
#23154=CARTESIAN_POINT('Ctrl Pts',(38.3381015974855,33.0655632618739,-7.08373702740619E-16));
#23155=CARTESIAN_POINT('Ctrl Pts',(38.3460261690062,33.0815968043693,-6.93889390390723E-16));
#23156=CARTESIAN_POINT('Ctrl Pts',(38.3989870883303,33.1887510080204,-5.97088888833881E-16));
#23157=CARTESIAN_POINT('Ctrl Pts',(38.4467091567301,33.2980550637735,1.26900815615077E-15));
#23158=CARTESIAN_POINT('Ctrl Pts',(38.4889135757351,33.409246351529,1.0547118733939E-15));
#23159=CARTESIAN_POINT('Ctrl Pts',(38.5302818373033,33.5182347083035,8.44661246299018E-16));
#23160=CARTESIAN_POINT('Ctrl Pts',(38.5663491876186,33.6290368908256,3.13106813660632E-16));
#23161=CARTESIAN_POINT('Ctrl Pts',(38.5968048600256,33.7414193655312,4.9960036108132E-16));
#23162=CARTESIAN_POINT('Ctrl Pts',(38.6012591757497,33.7578559431745,5.26876105632901E-16));
#23163=CARTESIAN_POINT('Ctrl Pts',(38.6055933637529,33.7743263394091,3.42924457172855E-16));
#23164=CARTESIAN_POINT('Ctrl Pts',(38.6098063577125,33.7908298367184,3.33066907387547E-16));
#23165=CARTESIAN_POINT('Ctrl Pts',(38.6394749188516,33.9070500410733,3.19833619294622E-16));
#23166=CARTESIAN_POINT('Ctrl Pts',(38.6631375043611,34.0249121336904,2.13657224701249E-16));
#23167=CARTESIAN_POINT('Ctrl Pts',(38.6808849682855,34.1439802784308,6.10622663543836E-16));
#23168=CARTESIAN_POINT('Ctrl Pts',(38.6908685193634,34.2109601528418,8.33929201973265E-16));
#23169=CARTESIAN_POINT('Ctrl Pts',(38.6989793099884,34.2783216258907,1.0776972087123E-15));
#23170=CARTESIAN_POINT('Ctrl Pts',(38.705226464765,34.3459856591442,1.13797860024079E-15));
#23171=CARTESIAN_POINT('Ctrl Pts',(38.7081089504882,34.3772063695005,1.1657929023787E-15));
#23172=CARTESIAN_POINT('Ctrl Pts',(38.7105946047039,34.4084914721069,9.83922849187538E-16));
#23173=CARTESIAN_POINT('Ctrl Pts',(38.7126839762627,34.4398330679179,1.02695629777827E-15));
#23174=CARTESIAN_POINT('Ctrl Pts',(38.7138850693151,34.4578500514573,1.05169444256127E-15));
#23175=CARTESIAN_POINT('Ctrl Pts',(38.7149546915907,34.4758786502346,-4.64302084245928E-16));
#23176=CARTESIAN_POINT('Ctrl Pts',(38.715892912359,34.4939090237972,-4.44089209850063E-16));
#23177=CARTESIAN_POINT('Ctrl Pts',(38.7222038666684,34.6151905681615,-3.08127044991787E-16));
#23178=CARTESIAN_POINT('Ctrl Pts',(38.7225822971166,34.7366693867671,-2.99144274726584E-15));
#23179=CARTESIAN_POINT('Ctrl Pts',(38.7171864105867,34.8578982328034,-2.05391259555654E-15));
#23180=CARTESIAN_POINT('Ctrl Pts',(38.71190245704,34.9766122916381,-1.13583069320137E-15));
#23181=CARTESIAN_POINT('Ctrl Pts',(38.7010807679502,35.0950875649844,1.78168855748587E-15));
#23182=CARTESIAN_POINT('Ctrl Pts',(38.6848165352731,35.2128980770419,1.76247905159244E-15));
#23183=CARTESIAN_POINT('Ctrl Pts',(38.6687112067838,35.3295575613132,1.74345722568323E-15));
#23184=CARTESIAN_POINT('Ctrl Pts',(38.6472688142291,35.4455660470931,1.26625388930718E-16));
#23185=CARTESIAN_POINT('Ctrl Pts',(38.62053500354,35.5604910223212,1.80411241501588E-16));
#23186=CARTESIAN_POINT('Ctrl Pts',(38.6031281268642,35.6353207910372,2.15432201045671E-16));
#23187=CARTESIAN_POINT('Ctrl Pts',(38.5834769893052,35.7096907862118,1.51379352364637E-15));
#23188=CARTESIAN_POINT('Ctrl Pts',(38.5615843902035,35.7834747121961,1.2490009027033E-15));
#23189=CARTESIAN_POINT('Ctrl Pts',(38.5541960332861,35.8083754550181,1.15963817406959E-15));
#23190=CARTESIAN_POINT('Ctrl Pts',(38.5465523248095,35.8332093935643,2.32778305945499E-15));
#23191=CARTESIAN_POINT('Ctrl Pts',(38.5386531847276,35.8579714965102,2.3037127760972E-15));
#23192=CARTESIAN_POINT('Ctrl Pts',(38.5335667575399,35.8739163502969,2.28821339990993E-15));
#23193=CARTESIAN_POINT('Ctrl Pts',(38.528375210839,35.8898288067619,1.8799349255917E-16));
#23194=CARTESIAN_POINT('Ctrl Pts',(38.5230814037796,35.9056994997334,2.77555756156289E-16));
#23195=CARTESIAN_POINT('Ctrl Pts',(38.4861837480683,36.016317691632,9.0180169672523E-16));
#23196=CARTESIAN_POINT('Ctrl Pts',(38.4442853792632,36.1250244064477,1.67610385059537E-15));
#23197=CARTESIAN_POINT('Ctrl Pts',(38.3974510894444,36.2314004501635,1.54737334057131E-15));
#23198=CARTESIAN_POINT('Ctrl Pts',(38.3593370450265,36.3179699544917,1.44261162867242E-15));
#23199=CARTESIAN_POINT('Ctrl Pts',(38.3179530965748,36.4029957144323,1.09861093914672E-15));
#23200=CARTESIAN_POINT('Ctrl Pts',(38.27331318169,36.4862361414904,1.49186218934005E-15));
#23201=CARTESIAN_POINT('Ctrl Pts',(38.2516982037212,36.526541773829,1.68227736219745E-15));
#23202=CARTESIAN_POINT('Ctrl Pts',(38.2293195714479,36.5664285801089,1.70359564472489E-15));
#23203=CARTESIAN_POINT('Ctrl Pts',(38.2061773939932,36.6058676078699,1.76247905159244E-15));
#23204=CARTESIAN_POINT('Ctrl Pts',(38.1925910511184,36.629021529097,1.79704840691352E-15));
#23205=CARTESIAN_POINT('Ctrl Pts',(38.1787394785284,36.652024183054,3.81993764399042E-15));
#23206=CARTESIAN_POINT('Ctrl Pts',(38.1646367510805,36.6748472188681,3.75394160201381E-15));
#23207=CARTESIAN_POINT('Ctrl Pts',(38.1062052960737,36.7694092952617,3.48050195910614E-15));
#23208=CARTESIAN_POINT('Ctrl Pts',(38.0434225704545,36.8609661715359,-8.52927663010733E-16));
#23209=CARTESIAN_POINT('Ctrl Pts',(37.9763226192313,36.9491271397218,-6.21031004399697E-16));
#23210=CARTESIAN_POINT('Ctrl Pts',(37.9162919198372,37.0279999925776,-4.13565598690696E-16));
#23211=CARTESIAN_POINT('Ctrl Pts',(37.8528051248739,37.1041547391556,2.13873726282784E-15));
#23212=CARTESIAN_POINT('Ctrl Pts',(37.7858631238401,37.1772850733286,2.38004060904018E-15));
#23213=CARTESIAN_POINT('Ctrl Pts',(37.7510082002317,37.215362097793,2.52360662668101E-15));
#23214=CARTESIAN_POINT('Ctrl Pts',(37.71521617243,37.2526187144799,1.78459625189646E-16));
#23215=CARTESIAN_POINT('Ctrl Pts',(37.6785244495408,37.2890395253442,2.4980018054066E-16));
#23216=CARTESIAN_POINT('Ctrl Pts',(31.4836963557363,34.997016753135,6.38741669750802));
#23217=CARTESIAN_POINT('Ctrl Pts',(31.4810522497149,34.6831064242593,6.4016107071645));
#23218=CARTESIAN_POINT('Ctrl Pts',(31.5197088623892,34.3698361384337,6.41580471682098));
#23219=CARTESIAN_POINT('Ctrl Pts',(31.602283311232,34.0686052256029,6.42999872647746));
#23220=CARTESIAN_POINT('Ctrl Pts',(31.9067356658548,32.9579655303736,6.48233210226155));
#23221=CARTESIAN_POINT('Ctrl Pts',(32.8082071426114,32.0109890873326,6.53466547804563));
#23222=CARTESIAN_POINT('Ctrl Pts',(33.9025202849968,31.6522420135335,6.58699885382972));
#23223=CARTESIAN_POINT('Ctrl Pts',(34.9968334273823,31.2934949397344,6.6393322296138));
#23224=CARTESIAN_POINT('Ctrl Pts',(36.2839882353967,31.5229772351772,6.69166560539789));
#23225=CARTESIAN_POINT('Ctrl Pts',(37.1868794441274,32.2378302684166,6.74399898118197));
#23226=CARTESIAN_POINT('Ctrl Pts',(38.089770652858,32.952683301656,6.79633235696606));
#23227=CARTESIAN_POINT('Ctrl Pts',(38.6083982623049,34.1529070726919,6.84866573275014));
#23228=CARTESIAN_POINT('Ctrl Pts',(38.5102396094692,35.3003133216048,6.90099910853422));
#23229=CARTESIAN_POINT('Ctrl Pts',(38.4120809566336,36.4477195705176,6.95333248431831));
#23230=CARTESIAN_POINT('Ctrl Pts',(37.6971360415154,37.5423082973073,7.00566586010239));
#23231=CARTESIAN_POINT('Ctrl Pts',(36.6859407221977,38.0934406773841,7.05799923588648));
#23232=CARTESIAN_POINT('Ctrl Pts',(35.67474540288,38.6445730574609,7.11033261167056));
#23233=CARTESIAN_POINT('Ctrl Pts',(34.3672996793629,38.6522490908248,7.16266598745465));
#23234=CARTESIAN_POINT('Ctrl Pts',(33.3498295528725,38.1127747395053,7.21499936323873));
#23235=CARTESIAN_POINT('Ctrl Pts',(32.3323594263822,37.5733003881858,7.26733273902282));
#23236=CARTESIAN_POINT('Ctrl Pts',(31.6048648969186,36.4866756521828,7.3196661148069));
#23237=CARTESIAN_POINT('Ctrl Pts',(31.4934684170666,35.3406028059835,7.37199949059098));
#23238=CARTESIAN_POINT('Ctrl Pts',(31.4825294286169,35.2280599532493,7.37713855956333));
#23239=CARTESIAN_POINT('Ctrl Pts',(31.4775314630746,35.1149438434099,7.38227762853567));
#23240=CARTESIAN_POINT('Ctrl Pts',(31.47826034488,35.0017653187145,7.38741669750802));
#23241=CARTESIAN_POINT('Ctrl Pts',(33.9479286229388,31.0647048309474,8.));
#23242=CARTESIAN_POINT('Ctrl Pts',(32.6539236935135,31.4106472544613,7.94766662421592));
#23243=CARTESIAN_POINT('Ctrl Pts',(30.454936822078,33.4726324908028,7.84299987264775));
#23244=CARTESIAN_POINT('Ctrl Pts',(31.2187005389846,37.9557872897229,7.6859997452955));
#23245=CARTESIAN_POINT('Ctrl Pts',(35.3795268052061,39.7808547962683,7.52899961794324));
#23246=CARTESIAN_POINT('Ctrl Pts',(39.1969168896572,37.3225573472918,7.37199949059099));
#23247=CARTESIAN_POINT('Ctrl Pts',(39.2524338890068,32.7797860374403,7.21499936323873));
#23248=CARTESIAN_POINT('Ctrl Pts',(35.4939868648458,30.2288021766129,7.05799923588648));
#23249=CARTESIAN_POINT('Ctrl Pts',(31.2929572874421,31.9557502059188,6.90099910853422));
#23250=CARTESIAN_POINT('Ctrl Pts',(30.4158796925061,36.4127281597254,6.74399898118197));
#23251=CARTESIAN_POINT('Ctrl Pts',(33.6495204900336,39.6027890266495,6.58699885382972));
#23252=CARTESIAN_POINT('Ctrl Pts',(38.0941026784935,38.6655395297167,6.42999872647747));
#23253=CARTESIAN_POINT('Ctrl Pts',(39.7641964207046,34.4413384042963,6.27299859912521));
#23254=CARTESIAN_POINT('Ctrl Pts',(37.1621780526355,30.7181079801836,6.11599847177296));
#23255=CARTESIAN_POINT('Ctrl Pts',(32.6213195789955,30.8344845112897,5.95899834442071));
#23256=CARTESIAN_POINT('Ctrl Pts',(30.2134438300848,34.686122068773,5.80199821706845));
#23257=CARTESIAN_POINT('Ctrl Pts',(32.0977203234525,38.8192153272012,5.6449980897162));
#23258=CARTESIAN_POINT('Ctrl Pts',(36.5844981485848,39.5275823816942,5.48799796236394));
#23259=CARTESIAN_POINT('Ctrl Pts',(39.6504416291735,36.1760224717832,5.33099783501169));
#23260=CARTESIAN_POINT('Ctrl Pts',(38.5462893146292,31.7699121313011,5.17399770765944));
#23261=CARTESIAN_POINT('Ctrl Pts',(34.2621454354683,30.2602524703801,5.01699758030718));
#23262=CARTESIAN_POINT('Ctrl Pts',(30.6396427805907,33.0007699401812,4.85999745295493));
#23263=CARTESIAN_POINT('Ctrl Pts',(30.927114296777,37.5340161596205,4.70299732560268));
#23264=CARTESIAN_POINT('Ctrl Pts',(34.86678148609,39.7949857907703,4.54599719825042));
#23265=CARTESIAN_POINT('Ctrl Pts',(38.9259070000539,37.7562456562111,4.38899707089817));
#23266=CARTESIAN_POINT('Ctrl Pts',(39.4646340410498,33.2459536025622,4.23199694354592));
#23267=CARTESIAN_POINT('Ctrl Pts',(35.9998809069499,30.3085317794917,4.07499681619366));
#23268=CARTESIAN_POINT('Ctrl Pts',(31.6385249705421,31.5779945185253,3.91799668884141));
#23269=CARTESIAN_POINT('Ctrl Pts',(30.291435941871,35.9160024014201,3.76099656148915));
#23270=CARTESIAN_POINT('Ctrl Pts',(33.1665614759356,39.4326221439007,3.60399643413691));
#23271=CARTESIAN_POINT('Ctrl Pts',(37.6857489237188,38.9744670842276,3.44699630678464));
#23272=CARTESIAN_POINT('Ctrl Pts',(39.7965995458586,34.9523692628263,3.2899961794324));
#23273=CARTESIAN_POINT('Ctrl Pts',(37.6062933383462,30.9729823764193,3.13299605208014));
#23274=CARTESIAN_POINT('Ctrl Pts',(33.078898891504,30.6046608345122,2.97599592472789));
#23275=CARTESIAN_POINT('Ctrl Pts',(30.2741742372111,34.1776820732232,2.81899579737563));
#23276=CARTESIAN_POINT('Ctrl Pts',(31.7071428852578,38.4880837181509,2.66199567002338));
#23277=CARTESIAN_POINT('Ctrl Pts',(36.0928480916297,39.6706871647746,2.50499554267113));
#23278=CARTESIAN_POINT('Ctrl Pts',(39.4985859434327,36.6650407532663,2.34799541531887));
#23279=CARTESIAN_POINT('Ctrl Pts',(38.8703985950797,32.1663360606625,2.19099528796662));
#23280=CARTESIAN_POINT('Ctrl Pts',(34.7715877503781,30.208605539026,2.03399516061437));
#23281=CARTESIAN_POINT('Ctrl Pts',(30.8775962508689,32.547363326415,1.87699503326212));
#23282=CARTESIAN_POINT('Ctrl Pts',(30.6802039639638,37.0854261049008,1.71999490590986));
#23283=CARTESIAN_POINT('Ctrl Pts',(34.3564137772933,39.7534629455386,1.56299477855761));
#23284=CARTESIAN_POINT('Ctrl Pts',(38.6097344321268,38.159032706872,1.40599465120535));
#23285=CARTESIAN_POINT('Ctrl Pts',(39.6261697761982,33.7318499178854,1.2489945238531));
#23286=CARTESIAN_POINT('Ctrl Pts',(36.4942779564007,30.441864951573,1.09199439650085));
#23287=CARTESIAN_POINT('Ctrl Pts',(32.0224453946446,31.2391319593762,0.934994269148593));
#23288=CARTESIAN_POINT('Ctrl Pts',(30.2206294419397,35.4089493247815,0.77799414179634));
#23289=CARTESIAN_POINT('Ctrl Pts',(32.7044910542971,39.2117680815463,0.620994014444087));
#23290=CARTESIAN_POINT('Ctrl Pts',(37.246817707304,39.2384377086451,0.463993887091833));
#23291=CARTESIAN_POINT('Ctrl Pts',(39.7742802645754,35.4632838929154,0.30699375973958));
#23292=CARTESIAN_POINT('Ctrl Pts',(38.0208433725288,31.2750679875305,0.149993632387326));
#23293=CARTESIAN_POINT('Ctrl Pts',(33.5581043558821,30.4222449751611,-0.00700649496492684));
#23294=CARTESIAN_POINT('Ctrl Pts',(30.3892402311535,33.6841941049532,-0.164006622317179));
#23295=CARTESIAN_POINT('Ctrl Pts',(31.0334355704763,36.629077589988,-0.26867337388535));
#23296=CARTESIAN_POINT('Ctrl Pts',(31.9038714051976,37.6471475165632,-0.321006749669435));
#23297=CARTESIAN_POINT('Ctrl Pts',(33.9957950511247,31.243750214851,8.10700224988981));
#23298=CARTESIAN_POINT('Ctrl Pts',(32.7606638781546,31.573953185194,8.05466887410573));
#23299=CARTESIAN_POINT('Ctrl Pts',(30.6617250162538,33.5421236192438,7.95000212253755));
#23300=CARTESIAN_POINT('Ctrl Pts',(31.3907395308691,37.8213068893232,7.79300199518531));
#23301=CARTESIAN_POINT('Ctrl Pts',(35.3622593526719,39.5633387153612,7.63600186783305));
#23302=CARTESIAN_POINT('Ctrl Pts',(39.0059684185923,37.2168872122651,7.4790017404808));
#23303=CARTESIAN_POINT('Ctrl Pts',(39.0589595432527,32.8807998227341,7.32200161312854));
#23304=CARTESIAN_POINT('Ctrl Pts',(35.4715117863422,30.4458788911338,7.16500148577629));
#23305=CARTESIAN_POINT('Ctrl Pts',(31.4616177962741,32.0942554131942,7.00800135842404));
#23306=CARTESIAN_POINT('Ctrl Pts',(30.6244448814073,36.3484528144607,6.85100123107178));
#23307=CARTESIAN_POINT('Ctrl Pts',(33.7109636885558,39.3933744610575,6.69400110371954));
#23308=CARTESIAN_POINT('Ctrl Pts',(37.9533292985792,38.4987673044786,6.53700097636727));
#23309=CARTESIAN_POINT('Ctrl Pts',(39.5474382512424,34.4667560097307,6.38000084901502));
#23310=CARTESIAN_POINT('Ctrl Pts',(37.0638047457115,30.9129225919439,6.22300072166277));
#23311=CARTESIAN_POINT('Ctrl Pts',(32.7295431634706,31.0240043027649,6.06600059431052));
#23312=CARTESIAN_POINT('Ctrl Pts',(30.4312193082136,34.7004026734751,5.90900046695826));
#23313=CARTESIAN_POINT('Ctrl Pts',(32.2297662708491,38.6454512650169,5.75200033960601));
#23314=CARTESIAN_POINT('Ctrl Pts',(36.5124077291574,39.3215895168996,5.59500021225375));
#23315=CARTESIAN_POINT('Ctrl Pts',(39.4388589978718,36.1225166009669,5.4380000849015));
#23316=CARTESIAN_POINT('Ctrl Pts',(38.3849426545962,31.9168724729398,5.28099995754925));
#23317=CARTESIAN_POINT('Ctrl Pts',(34.295715840761,30.4758982808191,5.12399983019699));
#23318=CARTESIAN_POINT('Ctrl Pts',(30.8380273486519,33.0917295501202,4.96699970284475));
#23319=CARTESIAN_POINT('Ctrl Pts',(31.1124196812533,37.4187252153261,4.80999957549248));
#23320=CARTESIAN_POINT('Ctrl Pts',(34.8728425714575,39.5768267874833,4.65299944814023));
#23321=CARTESIAN_POINT('Ctrl Pts',(38.7472887526802,37.6308438653799,4.49599932078798));
#23322=CARTESIAN_POINT('Ctrl Pts',(39.2615051570579,33.3257580129361,4.33899919343573));
#23323=CARTESIAN_POINT('Ctrl Pts',(35.9543890052876,30.5219810107509,4.18199906608348));
#23324=CARTESIAN_POINT('Ctrl Pts',(31.7914630758879,31.7336865972209,4.02499893873122));
#23325=CARTESIAN_POINT('Ctrl Pts',(30.5056629879263,35.8743267469715,3.86799881137897));
#23326=CARTESIAN_POINT('Ctrl Pts',(33.2499780153063,39.2309497154396,3.71099868402671));
#23327=CARTESIAN_POINT('Ctrl Pts',(37.5635545452901,38.7936394831613,3.55399855667446));
#23328=CARTESIAN_POINT('Ctrl Pts',(39.5783671210399,34.954536333721,3.39699842932221));
#23329=CARTESIAN_POINT('Ctrl Pts',(37.4877139761171,31.1562008861948,3.23999830196995));
#23330=CARTESIAN_POINT('Ctrl Pts',(33.1663038435374,30.804636987371,3.0829981746177));
#23331=CARTESIAN_POINT('Ctrl Pts',(30.4891866445685,34.2150953351428,2.92599804726545));
#23332=CARTESIAN_POINT('Ctrl Pts',(31.8569590593748,38.3293852567711,2.76899791991319));
#23333=CARTESIAN_POINT('Ctrl Pts',(36.0431264322094,39.4581834158598,2.61199779256094));
#23334=CARTESIAN_POINT('Ctrl Pts',(39.2939123388708,36.5892858611738,2.45499766520869));
#23335=CARTESIAN_POINT('Ctrl Pts',(38.6943058313741,32.295260175901,2.29799753785643));
#23336=CARTESIAN_POINT('Ctrl Pts',(34.7819798956087,30.4266011464317,2.14099741050418));
#23337=CARTESIAN_POINT('Ctrl Pts',(31.0651545737294,32.6589517221855,1.98399728315193));
#23338=CARTESIAN_POINT('Ctrl Pts',(30.8767431068824,36.9905448059094,1.82699715579967));
#23339=CARTESIAN_POINT('Ctrl Pts',(34.3856952256649,39.5371931204316,1.66999702844742));
#23340=CARTESIAN_POINT('Ctrl Pts',(38.4455011892756,38.015305184674,1.51299690109516));
#23341=CARTESIAN_POINT('Ctrl Pts',(39.4156914491603,33.789547348077,1.35599677374291));
#23342=CARTESIAN_POINT('Ctrl Pts',(36.4262923139345,30.6492478808251,1.19899664639066));
#23343=CARTESIAN_POINT('Ctrl Pts',(32.1579161495709,31.4102413763875,1.0419965190384));
#23344=CARTESIAN_POINT('Ctrl Pts',(30.438077993986,35.3903432264567,0.884996391686151));
#23345=CARTESIAN_POINT('Ctrl Pts',(32.8089305595391,39.0201439210504,0.727996264333897));
#23346=CARTESIAN_POINT('Ctrl Pts',(37.1445935229203,39.0456001515887,0.570996136981644));
#23347=CARTESIAN_POINT('Ctrl Pts',(39.5570633072411,35.4422057173529,0.413996009629391));
#23348=CARTESIAN_POINT('Ctrl Pts',(37.8834030947066,31.4445424115665,0.256995882277137));
#23349=CARTESIAN_POINT('Ctrl Pts',(33.6237067435201,30.63052056076,0.0999957549248841));
#23350=CARTESIAN_POINT('Ctrl Pts',(30.5990174441545,33.7440597469193,-0.0570043724273687));
#23351=CARTESIAN_POINT('Ctrl Pts',(31.2139036219321,36.5549589254462,-0.161671123995539));
#23352=CARTESIAN_POINT('Ctrl Pts',(32.0447369588746,37.5267093987113,-0.214004499779624));
#23353=CARTESIAN_POINT('Ctrl Pts',(34.0436614793107,31.4227955987545,8.21400449977962));
#23354=CARTESIAN_POINT('Ctrl Pts',(32.8674040627957,31.7372591159268,8.16167112399554));
#23355=CARTESIAN_POINT('Ctrl Pts',(30.8685132104295,33.6116147476849,8.05700437242736));
#23356=CARTESIAN_POINT('Ctrl Pts',(31.5627785227536,37.6868264889233,7.90000424507513));
#23357=CARTESIAN_POINT('Ctrl Pts',(35.3449919001376,39.3458226344541,7.74300411772285));
#23358=CARTESIAN_POINT('Ctrl Pts',(38.8150199475273,37.1112170772383,7.58600399037062));
#23359=CARTESIAN_POINT('Ctrl Pts',(38.8654851974986,32.9818136080279,7.42900386301834));
#23360=CARTESIAN_POINT('Ctrl Pts',(35.4490367078385,30.6629556056548,7.27200373566611));
#23361=CARTESIAN_POINT('Ctrl Pts',(31.6302783051062,32.2327606204696,7.11500360831384));
#23362=CARTESIAN_POINT('Ctrl Pts',(30.8330100703084,36.284177469196,6.9580034809616));
#23363=CARTESIAN_POINT('Ctrl Pts',(33.7724068870781,39.1839598954654,6.80100335360933));
#23364=CARTESIAN_POINT('Ctrl Pts',(37.812555918665,38.3319950792405,6.64400322625709));
#23365=CARTESIAN_POINT('Ctrl Pts',(39.3306800817804,34.4921736151651,6.48700309890483));
#23366=CARTESIAN_POINT('Ctrl Pts',(36.9654314387874,31.1077372037044,6.33000297155258));
#23367=CARTESIAN_POINT('Ctrl Pts',(32.8377667479458,31.2135240942401,6.17300284420033));
#23368=CARTESIAN_POINT('Ctrl Pts',(30.6489947863424,34.7146832781773,6.01600271684807));
#23369=CARTESIAN_POINT('Ctrl Pts',(32.3618122182458,38.4716872028325,5.85900258949582));
#23370=CARTESIAN_POINT('Ctrl Pts',(36.4403173097299,39.1155966521051,5.70200246214356));
#23371=CARTESIAN_POINT('Ctrl Pts',(39.2272763665704,36.0690107301504,5.54500233479131));
#23372=CARTESIAN_POINT('Ctrl Pts',(38.2235959945632,32.0638328145787,5.38800220743906));
#23373=CARTESIAN_POINT('Ctrl Pts',(34.3292862460537,30.6915440912579,5.2310020800868));
#23374=CARTESIAN_POINT('Ctrl Pts',(31.0364119167131,33.1826891600592,5.07400195273456));
#23375=CARTESIAN_POINT('Ctrl Pts',(31.2977250657295,37.3034342710318,4.9170018253823));
#23376=CARTESIAN_POINT('Ctrl Pts',(34.8789036568251,39.3586677841964,4.76000169803004));
#23377=CARTESIAN_POINT('Ctrl Pts',(38.5686705053066,37.5054420745486,4.60300157067779));
#23378=CARTESIAN_POINT('Ctrl Pts',(39.0583762730659,33.4055624233101,4.44600144332554));
#23379=CARTESIAN_POINT('Ctrl Pts',(35.9088971036253,30.7354302420101,4.28900131597329));
#23380=CARTESIAN_POINT('Ctrl Pts',(31.9444011812337,31.8893786759165,4.13200118862103));
#23381=CARTESIAN_POINT('Ctrl Pts',(30.7198900339817,35.8326510925229,3.97500106126878));
#23382=CARTESIAN_POINT('Ctrl Pts',(33.333394554677,39.0292772869785,3.81800093391652));
#23383=CARTESIAN_POINT('Ctrl Pts',(37.4413601668615,38.6128118820951,3.66100080656427));
#23384=CARTESIAN_POINT('Ctrl Pts',(39.3601346962212,34.9567034046157,3.50400067921202));
#23385=CARTESIAN_POINT('Ctrl Pts',(37.3691346138881,31.3394193959702,3.34700055185976));
#23386=CARTESIAN_POINT('Ctrl Pts',(33.2537087955707,31.0046131402298,3.19000042450751));
#23387=CARTESIAN_POINT('Ctrl Pts',(30.7041990519258,34.2525085970623,3.03300029715526));
#23388=CARTESIAN_POINT('Ctrl Pts',(32.0067752334918,38.1706867953913,2.876000169803));
#23389=CARTESIAN_POINT('Ctrl Pts',(35.9934047727891,39.2456796669448,2.71900004245075));
#23390=CARTESIAN_POINT('Ctrl Pts',(39.0892387343089,36.5135309690814,2.5619999150985));
#23391=CARTESIAN_POINT('Ctrl Pts',(38.5182130676685,32.4241842911394,2.40499978774624));
#23392=CARTESIAN_POINT('Ctrl Pts',(34.7923720408392,30.6445967538374,2.24799966039399));
#23393=CARTESIAN_POINT('Ctrl Pts',(31.25271289659,32.770540117956,2.09099953304174));
#23394=CARTESIAN_POINT('Ctrl Pts',(31.0732822498009,36.8956635069179,1.93399940568948));
#23395=CARTESIAN_POINT('Ctrl Pts',(34.4149766740365,39.3209232953247,1.77699927833723));
#23396=CARTESIAN_POINT('Ctrl Pts',(38.2812679464245,37.8715776624759,1.61999915098497));
#23397=CARTESIAN_POINT('Ctrl Pts',(39.2052131221224,33.8472447782685,1.46299902363272));
#23398=CARTESIAN_POINT('Ctrl Pts',(36.3583066714682,30.8566308100772,1.30599889628047));
#23399=CARTESIAN_POINT('Ctrl Pts',(32.2933869044973,31.5813507933988,1.14899876892822));
#23400=CARTESIAN_POINT('Ctrl Pts',(30.6555265460323,35.3717371281319,0.991998641575962));
#23401=CARTESIAN_POINT('Ctrl Pts',(32.9133700647812,38.8285197605545,0.834998514223708));
#23402=CARTESIAN_POINT('Ctrl Pts',(37.0423693385366,38.8527625945324,0.677998386871455));
#23403=CARTESIAN_POINT('Ctrl Pts',(39.3398463499068,35.4211275417905,0.520998259519202));
#23404=CARTESIAN_POINT('Ctrl Pts',(37.7459628168843,31.6140168356026,0.363998132166948));
#23405=CARTESIAN_POINT('Ctrl Pts',(33.6893091311581,30.8387961463588,0.206998004814695));
#23406=CARTESIAN_POINT('Ctrl Pts',(30.8087946571555,33.8039253888853,0.0499978774624422));
#23407=CARTESIAN_POINT('Ctrl Pts',(31.3943716733878,36.4808402609044,-0.0546688741057282));
#23408=CARTESIAN_POINT('Ctrl Pts',(32.1856025125517,37.4062712808594,-0.107002249889813));
#23409=CARTESIAN_POINT('Ctrl Pts',(34.0915279074966,31.601840982658,8.32100674966943));
#23410=CARTESIAN_POINT('Ctrl Pts',(32.9741442474368,31.9005650466595,8.26867337388535));
#23411=CARTESIAN_POINT('Ctrl Pts',(31.0753014046052,33.6811058761259,8.16400662231717));
#23412=CARTESIAN_POINT('Ctrl Pts',(31.7348175146381,37.5523460885235,8.00700649496493));
#23413=CARTESIAN_POINT('Ctrl Pts',(35.3277244476034,39.128306553547,7.85000636761267));
#23414=CARTESIAN_POINT('Ctrl Pts',(38.6240714764623,37.0055469422116,7.69300624026043));
#23415=CARTESIAN_POINT('Ctrl Pts',(38.6720108517446,33.0828273933217,7.53600611290816));
#23416=CARTESIAN_POINT('Ctrl Pts',(35.4265616293347,30.8800323201757,7.37900598555592));
#23417=CARTESIAN_POINT('Ctrl Pts',(31.7989388139383,32.371265827745,7.22200585820365));
#23418=CARTESIAN_POINT('Ctrl Pts',(31.0415752592096,36.2199021239313,7.06500573085141));
#23419=CARTESIAN_POINT('Ctrl Pts',(33.8338500856003,38.9745453298735,6.90800560349915));
#23420=CARTESIAN_POINT('Ctrl Pts',(37.6717825387507,38.1652228540024,6.75100547614691));
#23421=CARTESIAN_POINT('Ctrl Pts',(39.1139219123182,34.5175912205995,6.59400534879464));
#23422=CARTESIAN_POINT('Ctrl Pts',(36.8670581318634,31.3025518154648,6.4370052214424));
#23423=CARTESIAN_POINT('Ctrl Pts',(32.9459903324209,31.4030438857154,6.28000509409014));
#23424=CARTESIAN_POINT('Ctrl Pts',(30.8667702644712,34.7289638828794,6.12300496673789));
#23425=CARTESIAN_POINT('Ctrl Pts',(32.4938581656424,38.2979231406482,5.96600483938563));
#23426=CARTESIAN_POINT('Ctrl Pts',(36.3682268903025,38.9096037873106,5.80900471203337));
#23427=CARTESIAN_POINT('Ctrl Pts',(39.0156937352688,36.0155048593341,5.65200458468113));
#23428=CARTESIAN_POINT('Ctrl Pts',(38.0622493345301,32.2107931562174,5.49500445732887));
#23429=CARTESIAN_POINT('Ctrl Pts',(34.3628566513464,30.9071899016968,5.33800432997662));
#23430=CARTESIAN_POINT('Ctrl Pts',(31.2347964847743,33.2736487699982,5.18100420262436));
#23431=CARTESIAN_POINT('Ctrl Pts',(31.4830304502057,37.1881433267374,5.02400407527211));
#23432=CARTESIAN_POINT('Ctrl Pts',(34.8849647421926,39.1405087809095,4.86700394791985));
#23433=CARTESIAN_POINT('Ctrl Pts',(38.3900522579329,37.3800402837173,4.71000382056761));
#23434=CARTESIAN_POINT('Ctrl Pts',(38.855247389074,33.4853668336842,4.55300369321535));
#23435=CARTESIAN_POINT('Ctrl Pts',(35.863405201963,30.9488794732692,4.3960035658631));
#23436=CARTESIAN_POINT('Ctrl Pts',(32.0973392865795,32.0450707546122,4.23900343851084));
#23437=CARTESIAN_POINT('Ctrl Pts',(30.9341170800371,35.7909754380742,4.08200331115859));
#23438=CARTESIAN_POINT('Ctrl Pts',(33.4168110940477,38.8276048585174,3.92500318380633));
#23439=CARTESIAN_POINT('Ctrl Pts',(37.3191657884328,38.4319842810288,3.76800305645409));
#23440=CARTESIAN_POINT('Ctrl Pts',(39.1419022714024,34.9588704755104,3.61100292910183));
#23441=CARTESIAN_POINT('Ctrl Pts',(37.250555251659,31.5226379057457,3.45400280174958));
#23442=CARTESIAN_POINT('Ctrl Pts',(33.3411137476041,31.2045892930886,3.29700267439732));
#23443=CARTESIAN_POINT('Ctrl Pts',(30.9192114592832,34.2899218589819,3.14000254704507));
#23444=CARTESIAN_POINT('Ctrl Pts',(32.1565914076088,38.0119883340115,2.98300241969281));
#23445=CARTESIAN_POINT('Ctrl Pts',(35.9436831133688,39.0331759180299,2.82600229234056));
#23446=CARTESIAN_POINT('Ctrl Pts',(38.884565129747,36.4377760769889,2.66900216498831));
#23447=CARTESIAN_POINT('Ctrl Pts',(38.3421203039629,32.5531084063779,2.51200203763606));
#23448=CARTESIAN_POINT('Ctrl Pts',(34.8027641860698,30.8625923612432,2.3550019102838));
#23449=CARTESIAN_POINT('Ctrl Pts',(31.4402712194505,32.8821285137264,2.19800178293155));
#23450=CARTESIAN_POINT('Ctrl Pts',(31.2698213927195,36.8007822079265,2.04100165557929));
#23451=CARTESIAN_POINT('Ctrl Pts',(34.4442581224081,39.1046534702177,1.88400152822704));
#23452=CARTESIAN_POINT('Ctrl Pts',(38.1170347035733,37.7278501402779,1.72700140087479));
#23453=CARTESIAN_POINT('Ctrl Pts',(38.9947347950846,33.90494220846,1.57000127352253));
#23454=CARTESIAN_POINT('Ctrl Pts',(36.290321029002,31.0640137393293,1.41300114617028));
#23455=CARTESIAN_POINT('Ctrl Pts',(32.4288576594237,31.7524602104101,1.25600101881803));
#23456=CARTESIAN_POINT('Ctrl Pts',(30.8729750980786,35.353131029807,1.09900089146577));
#23457=CARTESIAN_POINT('Ctrl Pts',(33.0178095700233,38.6368956000587,0.94200076411352));
#23458=CARTESIAN_POINT('Ctrl Pts',(36.9401451541529,38.6599250374761,0.785000636761265));
#23459=CARTESIAN_POINT('Ctrl Pts',(39.1226293925725,35.400049366228,0.628000509409013));
#23460=CARTESIAN_POINT('Ctrl Pts',(37.6085225390622,31.7834912596387,0.471000382056759));
#23461=CARTESIAN_POINT('Ctrl Pts',(33.754911518796,31.0470717319576,0.314000254704506));
#23462=CARTESIAN_POINT('Ctrl Pts',(31.0185718701565,33.8637910308514,0.157000127352253));
#23463=CARTESIAN_POINT('Ctrl Pts',(31.5748397248436,36.4067215963626,0.0523333757840826));
#23464=CARTESIAN_POINT('Ctrl Pts',(32.3264680662287,37.2858331630075,-2.22044604925031E-15));
#23465=CARTESIAN_POINT('Ctrl Pts',(32.3264680662287,37.2858331630075,-2.16493489801906E-15));
#23466=CARTESIAN_POINT('Ctrl Pts',(32.2493253814486,37.208720274039,-2.02930540817935E-15));
#23467=CARTESIAN_POINT('Ctrl Pts',(32.1762950504991,37.1279852253981,-2.22088175559797E-15));
#23468=CARTESIAN_POINT('Ctrl Pts',(32.1073693836416,37.0440465177293,-2.44249065417534E-15));
#23469=CARTESIAN_POINT('Ctrl Pts',(32.0366838276613,36.957964590773,-2.66975792514024E-15));
#23470=CARTESIAN_POINT('Ctrl Pts',(31.9703148460741,36.8685128644539,-1.62037951577862E-15));
#23471=CARTESIAN_POINT('Ctrl Pts',(31.9082840182324,36.7760965840633,-1.60982338570648E-15));
#23472=CARTESIAN_POINT('Ctrl Pts',(31.8449621738338,36.681756889908,-1.59904755618531E-15));
#23473=CARTESIAN_POINT('Ctrl Pts',(31.7861605220008,36.5843273727301,-2.0500807145436E-15));
#23474=CARTESIAN_POINT('Ctrl Pts',(31.7319388093681,36.4841996609406,-1.27675647831893E-15));
#23475=CARTESIAN_POINT('Ctrl Pts',(31.6801495481474,36.3885637990409,-5.38124499843711E-16));
#23476=CARTESIAN_POINT('Ctrl Pts',(31.6325385292086,36.2904655679991,-4.81778164441647E-15));
#23477=CARTESIAN_POINT('Ctrl Pts',(31.5891933275412,36.1902216120283,-5.77315972805081E-15));
#23478=CARTESIAN_POINT('Ctrl Pts',(31.5821551531175,36.1739445059149,-5.92828918493564E-15));
#23479=CARTESIAN_POINT('Ctrl Pts',(31.5752295287451,36.1576107865788,-2.14687895786075E-15));
#23480=CARTESIAN_POINT('Ctrl Pts',(31.5684169229622,36.1412217669136,-2.1094237467878E-15));
#23481=CARTESIAN_POINT('Ctrl Pts',(31.5619076362096,36.1255624388982,-2.07363616168158E-15));
#23482=CARTESIAN_POINT('Ctrl Pts',(31.5555045468442,36.1098598194457,-5.01667023260332E-15));
#23483=CARTESIAN_POINT('Ctrl Pts',(31.5492098653947,36.0941205526839,-4.94049245958195E-15));
#23484=CARTESIAN_POINT('Ctrl Pts',(31.5058243818098,35.9856391775398,-4.41544452070402E-15));
#23485=CARTESIAN_POINT('Ctrl Pts',(31.4675527596774,35.875340817696,2.70422581427715E-15));
#23486=CARTESIAN_POINT('Ctrl Pts',(31.4344236193294,35.7636572747171,2.16493489801906E-15));
#23487=CARTESIAN_POINT('Ctrl Pts',(31.4008599589415,35.6505088963383,1.61857067083336E-15));
#23488=CARTESIAN_POINT('Ctrl Pts',(31.3725741668882,35.5359380090966,1.5704555898309E-16));
#23489=CARTESIAN_POINT('Ctrl Pts',(31.3496386440377,35.4203611044154,3.88578058618805E-16));
#23490=CARTESIAN_POINT('Ctrl Pts',(31.3256636190246,35.2995459305591,6.30604259909078E-16));
#23491=CARTESIAN_POINT('Ctrl Pts',(31.3075340503036,35.1776306642325,-4.77206768499493E-16));
#23492=CARTESIAN_POINT('Ctrl Pts',(31.2953883637021,35.0550676565495,-7.49400541621981E-16));
#23493=CARTESIAN_POINT('Ctrl Pts',(31.2862790987509,34.9631454007872,-9.53545871463847E-16));
#23494=CARTESIAN_POINT('Ctrl Pts',(31.2805368906832,34.8708581938176,-1.66063273915206E-15));
#23495=CARTESIAN_POINT('Ctrl Pts',(31.2782432669551,34.7783934177904,-1.83186799063151E-15));
#23496=CARTESIAN_POINT('Ctrl Pts',(31.2776956893352,34.7563184621811,-1.87274853712248E-15));
#23497=CARTESIAN_POINT('Ctrl Pts',(31.2773448230031,34.7342288592592,-1.15850189636716E-15));
#23498=CARTESIAN_POINT('Ctrl Pts',(31.2771918797387,34.7121562214804,-1.19348975147204E-15));
#23499=CARTESIAN_POINT('Ctrl Pts',(31.2763569642807,34.5916619548496,-1.38448803559665E-15));
#23500=CARTESIAN_POINT('Ctrl Pts',(31.2814102215213,34.471522491006,-2.99090776565717E-15));
#23501=CARTESIAN_POINT('Ctrl Pts',(31.2924206159431,34.3521638613563,-2.66453525910038E-15));
#23502=CARTESIAN_POINT('Ctrl Pts',(31.3033603504718,34.2335712231593,-2.34025726846702E-15));
#23503=CARTESIAN_POINT('Ctrl Pts',(31.3201807588279,34.1157485527733,3.70943136885229E-16));
#23504=CARTESIAN_POINT('Ctrl Pts',(31.342998921253,33.9991008864625,6.93889390390723E-16));
#23505=CARTESIAN_POINT('Ctrl Pts',(31.3458725738232,33.9844106208813,7.34560296054722E-16));
#23506=CARTESIAN_POINT('Ctrl Pts',(31.348841419242,33.9697389843081,-2.36384243829245E-16));
#23507=CARTESIAN_POINT('Ctrl Pts',(31.3519057505532,33.9550867820407,-2.22044604925031E-16));
#23508=CARTESIAN_POINT('Ctrl Pts',(31.3758162053254,33.8407581458576,-1.09500521307372E-16));
#23509=CARTESIAN_POINT('Ctrl Pts',(31.405535880703,33.7276122083523,-1.31284998081472E-15));
#23510=CARTESIAN_POINT('Ctrl Pts',(31.4407586285186,33.6159154648327,-2.41473507855972E-15));
#23511=CARTESIAN_POINT('Ctrl Pts',(31.4627238926124,33.5462602385377,-3.10188184234126E-15));
#23512=CARTESIAN_POINT('Ctrl Pts',(31.4868303230444,33.4771686776378,-2.63257088976062E-16));
#23513=CARTESIAN_POINT('Ctrl Pts',(31.5130135264214,33.4087075970126,-2.22044604925031E-16));
#23514=CARTESIAN_POINT('Ctrl Pts',(31.5219635139129,33.385306112999,-2.0795728293307E-16));
#23515=CARTESIAN_POINT('Ctrl Pts',(31.5311562173418,33.361978315516,-2.32755725796262E-15));
#23516=CARTESIAN_POINT('Ctrl Pts',(31.5405892520308,33.3387269417829,-2.58126853225349E-15));
#23517=CARTESIAN_POINT('Ctrl Pts',(31.5473379087033,33.3220922591317,-2.76278066918334E-15));
#23518=CARTESIAN_POINT('Ctrl Pts',(31.5542101234624,33.3054955734371,-8.17270399285879E-16));
#23519=CARTESIAN_POINT('Ctrl Pts',(31.5611979545174,33.288954186216,-7.7715611723761E-16));
#23520=CARTESIAN_POINT('Ctrl Pts',(31.6071192859873,33.1802505670847,-5.13540522049862E-16));
#23521=CARTESIAN_POINT('Ctrl Pts',(31.6580936513602,33.0737733268919,-1.22043518676627E-15));
#23522=CARTESIAN_POINT('Ctrl Pts',(31.713762608453,32.9697768155529,-8.60422844084496E-16));
#23523=CARTESIAN_POINT('Ctrl Pts',(31.7713468082815,32.8622023934125,-4.88024585443386E-16));
#23524=CARTESIAN_POINT('Ctrl Pts',(31.8339543542604,32.7572816421653,-1.6844387016455E-15));
#23525=CARTESIAN_POINT('Ctrl Pts',(31.9012439032021,32.6553034111749,-1.60982338570648E-15));
#23526=CARTESIAN_POINT('Ctrl Pts',(31.9691666425039,32.5523655715406,-1.53450594440749E-15));
#23527=CARTESIAN_POINT('Ctrl Pts',(32.0418603487199,32.4524251462352,-2.14412608245669E-16));
#23528=CARTESIAN_POINT('Ctrl Pts',(32.119024465224,32.3557974897081,-1.11022302462516E-16));
#23529=CARTESIAN_POINT('Ctrl Pts',(32.1734376325243,32.2876593825328,-3.81154351168831E-17));
#23530=CARTESIAN_POINT('Ctrl Pts',(32.2300747937192,32.2211689202647,2.3957932567246E-15));
#23531=CARTESIAN_POINT('Ctrl Pts',(32.2888436140898,32.1564451639975,2.85882428840978E-15));
#23532=CARTESIAN_POINT('Ctrl Pts',(32.3150756619651,32.1275550712175,3.06550279776831E-15));
#23533=CARTESIAN_POINT('Ctrl Pts',(32.3417325486905,32.0990170804093,1.33832078810492E-15));
#23534=CARTESIAN_POINT('Ctrl Pts',(32.3688066730543,32.0708423529797,1.58206781009085E-15));
#23535=CARTESIAN_POINT('Ctrl Pts',(32.3804284156068,32.0587481694606,1.68669779181855E-15));
#23536=CARTESIAN_POINT('Ctrl Pts',(32.3921256212299,32.0467224591722,5.62787663488911E-16));
#23537=CARTESIAN_POINT('Ctrl Pts',(32.4038911827787,32.0347724888588,5.27355936696949E-16));
#23538=CARTESIAN_POINT('Ctrl Pts',(32.4923334498706,31.9449440126051,2.61014017404201E-16));
#23539=CARTESIAN_POINT('Ctrl Pts',(32.584735051869,31.8592881592603,-7.81291389151021E-17));
#23540=CARTESIAN_POINT('Ctrl Pts',(32.6807672456031,31.778123082898,1.11022302462516E-16));
#23541=CARTESIAN_POINT('Ctrl Pts',(32.7628075187761,31.7087837834614,2.72614319871455E-16));
#23542=CARTESIAN_POINT('Ctrl Pts',(32.8474985084852,31.6427220447333,9.36044375735486E-16));
#23543=CARTESIAN_POINT('Ctrl Pts',(32.9346594679295,31.5801538004245,1.38777878078145E-16));
#23544=CARTESIAN_POINT('Ctrl Pts',(32.9737706916096,31.5520779208788,-2.18974819016821E-16));
#23545=CARTESIAN_POINT('Ctrl Pts',(33.0133795255453,31.5247057193814,-1.25086984652678E-15));
#23546=CARTESIAN_POINT('Ctrl Pts',(33.0534708815057,31.4980580630162,-1.7277845820729E-15));
#23547=CARTESIAN_POINT('Ctrl Pts',(33.0807055590029,31.479955898353,-2.0517601300469E-15));
#23548=CARTESIAN_POINT('Ctrl Pts',(33.1081685502538,31.462184715489,8.66601268491E-16));
#23549=CARTESIAN_POINT('Ctrl Pts',(33.1358251623594,31.4447698310871,9.5062846483529E-16));
#23550=CARTESIAN_POINT('Ctrl Pts',(33.2426295858021,31.377516955689,1.27512505265964E-15));
#23551=CARTESIAN_POINT('Ctrl Pts',(33.3523807267505,31.315530896685,3.7726686237795E-15));
#23552=CARTESIAN_POINT('Ctrl Pts',(33.4647766052556,31.2591453155976,2.97331603782425E-15));
#23553=CARTESIAN_POINT('Ctrl Pts',(33.5668702670808,31.2079280421183,2.24723218426034E-15));
#23554=CARTESIAN_POINT('Ctrl Pts',(33.6711468426795,31.1613315802118,-1.73124610826904E-15));
#23555=CARTESIAN_POINT('Ctrl Pts',(33.7774033647392,31.1196350998879,-2.12763834328555E-15));
#23556=CARTESIAN_POINT('Ctrl Pts',(33.8328339031569,31.0978834152884,-2.36077539403599E-15));
#23557=CARTESIAN_POINT('Ctrl Pts',(33.8888035920626,31.0774657030867,3.31895026664625E-16));
#23558=CARTESIAN_POINT('Ctrl Pts',(33.9452683089267,31.0583698510224,1.66533453693773E-16));
#23559=CARTESIAN_POINT('Ctrl Pts',(31.4846882532079,35.0028111988253,7.11258330249198));
#23560=CARTESIAN_POINT('Ctrl Pts',(31.4819571032991,35.3538027877235,7.09672411194513));
#23561=CARTESIAN_POINT('Ctrl Pts',(31.5304045241347,35.7040585316776,7.08086492139827));
#23562=CARTESIAN_POINT('Ctrl Pts',(31.6331816560628,36.037569942224,7.06500573085141));
#23563=CARTESIAN_POINT('Ctrl Pts',(31.9723335346732,37.138116525912,7.01267235506733));
#23564=CARTESIAN_POINT('Ctrl Pts',(32.9030918101368,38.0563309278927,6.96033897928324));
#23565=CARTESIAN_POINT('Ctrl Pts',(34.008126356727,38.3805510495713,6.90800560349915));
#23566=CARTESIAN_POINT('Ctrl Pts',(35.1131609033171,38.7047711712498,6.85567222771507));
#23567=CARTESIAN_POINT('Ctrl Pts',(36.3924717210339,38.4349970126261,6.80333885193099));
#23568=CARTESIAN_POINT('Ctrl Pts',(37.2724836921536,37.6921713277471,6.75100547614691));
#23569=CARTESIAN_POINT('Ctrl Pts',(38.1524956632732,36.9493456428681,6.69867210036282));
#23570=CARTESIAN_POINT('Ctrl Pts',(38.6332087877957,35.7334684317338,6.64633872457873));
#23571=CARTESIAN_POINT('Ctrl Pts',(38.4990880533145,34.5896899253109,6.59400534879465));
#23572=CARTESIAN_POINT('Ctrl Pts',(38.3649673188333,33.4459114188879,6.54167197301056));
#23573=CARTESIAN_POINT('Ctrl Pts',(37.6160127253483,32.3742316171763,6.48933859722648));
#23574=CARTESIAN_POINT('Ctrl Pts',(36.5880241286988,31.8551403946957,6.4370052214424));
#23575=CARTESIAN_POINT('Ctrl Pts',(35.5600355320492,31.336049172215,6.38467184565831));
#23576=CARTESIAN_POINT('Ctrl Pts',(34.2530129322351,31.3695465289652,6.33233846987422));
#23577=CARTESIAN_POINT('Ctrl Pts',(33.2529649543364,31.9406152068676,6.28000509409014));
#23578=CARTESIAN_POINT('Ctrl Pts',(32.2529169764377,32.51168388477,6.22767171830605));
#23579=CARTESIAN_POINT('Ctrl Pts',(31.5598436204544,33.6203238838247,6.17533834252197));
#23580=CARTESIAN_POINT('Ctrl Pts',(31.4844882593247,34.7694704263135,6.12300496673789));
#23581=CARTESIAN_POINT('Ctrl Pts',(31.4794861724725,34.8457507430058,6.11953107865592));
#23582=CARTESIAN_POINT('Ctrl Pts',(31.4772059369411,34.9222095437145,6.11605719057395));
#23583=CARTESIAN_POINT('Ctrl Pts',(31.4775764275568,34.998690818207,6.11258330249198));
#23584=CARTESIAN_POINT('Origin',(-35.,35.,10.2084234471775));
#23585=CARTESIAN_POINT('Ctrl Pts',(-39.0784090602678,35.0020440536088,7.70842344717747));
#23586=CARTESIAN_POINT('Ctrl Pts',(-39.0792531838394,35.133112279499,7.70328437820512));
#23587=CARTESIAN_POINT('Ctrl Pts',(-39.0145240110799,36.5980970201662,7.64581193344869));
#23588=CARTESIAN_POINT('Ctrl Pts',(-37.2468179015868,39.238437726829,7.53600611290815));
#23589=CARTESIAN_POINT('Ctrl Pts',(-32.7044909023729,39.2117683922069,7.37900598555592));
#23590=CARTESIAN_POINT('Ctrl Pts',(-30.2206292307696,35.4089492839864,7.22200585820365));
#23591=CARTESIAN_POINT('Ctrl Pts',(-32.0224452414743,31.2391318114334,7.0650057308514));
#23592=CARTESIAN_POINT('Ctrl Pts',(-36.4942780330333,30.4418647129305,6.90800560349915));
#23593=CARTESIAN_POINT('Ctrl Pts',(-38.8653529438983,32.9326279141667,6.7891448422745));
#23594=CARTESIAN_POINT('Ctrl Pts',(-39.0751757451768,34.6330161300415,6.72261745683394));
#23595=CARTESIAN_POINT('Ctrl Pts',(-39.0721136942453,34.9965451882256,6.70842344717746));
#23596=CARTESIAN_POINT('Ctrl Pts',(-39.0691248821302,34.9959228837483,7.79157655282255));
#23597=CARTESIAN_POINT('Ctrl Pts',(-39.0629617588157,35.8984240805364,7.75638428364687));
#23598=CARTESIAN_POINT('Ctrl Pts',(-38.3270254278953,38.1550448362135,7.6688586386871));
#23599=CARTESIAN_POINT('Ctrl Pts',(-34.6204731393245,39.7808563212243,7.52899961794324));
#23600=CARTESIAN_POINT('Ctrl Pts',(-30.8030827008644,37.3225569109026,7.37199949059099));
#23601=CARTESIAN_POINT('Ctrl Pts',(-30.7475658132336,32.7797862032913,7.21499936323873));
#23602=CARTESIAN_POINT('Ctrl Pts',(-34.5060130464714,30.2288015790917,7.05799923588648));
#23603=CARTESIAN_POINT('Ctrl Pts',(-38.2826807551488,31.7813043056651,6.91685829908108));
#23604=CARTESIAN_POINT('Ctrl Pts',(-39.0636920303636,34.0684206251935,6.82805073805977));
#23605=CARTESIAN_POINT('Ctrl Pts',(-39.070966199943,35.0032555604945,6.79157655282255));
#23606=CARTESIAN_POINT('Ctrl Pts',(-32.3264680662287,37.2858331630075,8.));
#23607=CARTESIAN_POINT('Ctrl Pts',(-31.5748397248436,36.4067215963625,7.94766662421592));
#23608=CARTESIAN_POINT('Ctrl Pts',(-31.0185734566188,33.863789346735,7.84299987264775));
#23609=CARTESIAN_POINT('Ctrl Pts',(-33.7549107807148,31.0470722659105,7.68599974529549));
#23610=CARTESIAN_POINT('Ctrl Pts',(-37.6085229887763,31.7834906538058,7.52899961794324));
#23611=CARTESIAN_POINT('Ctrl Pts',(-39.122629437071,35.4000496587684,7.37199949059099));
#23612=CARTESIAN_POINT('Ctrl Pts',(-36.9401453219176,38.6599250531781,7.21499936323873));
#23613=CARTESIAN_POINT('Ctrl Pts',(-33.0178094388356,38.6368958683166,7.05799923588648));
#23614=CARTESIAN_POINT('Ctrl Pts',(-30.8729749157314,35.3531309945801,6.90099910853423));
#23615=CARTESIAN_POINT('Ctrl Pts',(-32.4288575271599,31.7524600826604,6.74399898118197));
#23616=CARTESIAN_POINT('Ctrl Pts',(-36.2903210951748,31.0640135332596,6.58699885382972));
#23617=CARTESIAN_POINT('Ctrl Pts',(-38.9947349861635,33.9049421642868,6.42999872647747));
#23618=CARTESIAN_POINT('Ctrl Pts',(-38.1170348549754,37.7278502673058,6.27299859912521));
#23619=CARTESIAN_POINT('Ctrl Pts',(-34.4442580951562,39.1046536709688,6.11599847177296));
#23620=CARTESIAN_POINT('Ctrl Pts',(-31.2698212127753,36.8007822935419,5.95899834442071));
#23621=CARTESIAN_POINT('Ctrl Pts',(-31.4402710474498,32.8821284121656,5.80199821706844));
#23622=CARTESIAN_POINT('Ctrl Pts',(-34.8027641765881,30.8625921610582,5.6449980897162));
#23623=CARTESIAN_POINT('Ctrl Pts',(-38.3421204653421,32.553108288411,5.48799796236394));
#23624=CARTESIAN_POINT('Ctrl Pts',(-38.884565317352,36.4377761463179,5.33099783501169));
#23625=CARTESIAN_POINT('Ctrl Pts',(-35.9436831589371,39.0331761128571,5.17399770765944));
#23626=CARTESIAN_POINT('Ctrl Pts',(-32.1565912702954,38.0119884794394,5.01699758030718));
#23627=CARTESIAN_POINT('Ctrl Pts',(-30.9192112622106,34.2899218247053,4.85999745295493));
#23628=CARTESIAN_POINT('Ctrl Pts',(-33.3411136674927,31.2045891097909,4.70299732560268));
#23629=CARTESIAN_POINT('Ctrl Pts',(-37.2505553603438,31.522637737819,4.54599719825043));
#23630=CARTESIAN_POINT('Ctrl Pts',(-39.1419024714255,34.9588704735221,4.38899707089817));
#23631=CARTESIAN_POINT('Ctrl Pts',(-37.3191659004311,38.4319844467691,4.23199694354592));
#23632=CARTESIAN_POINT('Ctrl Pts',(-33.4168110175916,38.8276050433616,4.07499681619367));
#23633=CARTESIAN_POINT('Ctrl Pts',(-30.9341168836852,35.7909754762728,3.91799668884141));
#23634=CARTESIAN_POINT('Ctrl Pts',(-32.0973391464029,32.0450706119108,3.76099656148916));
#23635=CARTESIAN_POINT('Ctrl Pts',(-35.8634052436587,30.9488792776308,3.6039964341369));
#23636=CARTESIAN_POINT('Ctrl Pts',(-38.8552475752543,33.4853667605377,3.44699630678465));
#23637=CARTESIAN_POINT('Ctrl Pts',(-38.390052421646,37.3800403986573,3.2899961794324));
#23638=CARTESIAN_POINT('Ctrl Pts',(-34.8849647366394,39.1405089808617,3.13299605208014));
#23639=CARTESIAN_POINT('Ctrl Pts',(-31.4830302803583,37.1881434324151,2.97599592472789));
#23640=CARTESIAN_POINT('Ctrl Pts',(-31.2347963029507,33.2736486866154,2.81899579737564));
#23641=CARTESIAN_POINT('Ctrl Pts',(-34.3628566205626,30.9071897040694,2.66199567002338));
#23642=CARTESIAN_POINT('Ctrl Pts',(-38.0622494824414,32.2107930214718,2.50499554267113));
#23643=CARTESIAN_POINT('Ctrl Pts',(-39.0156939291453,36.0155049084671,2.34799541531888));
#23644=CARTESIAN_POINT('Ctrl Pts',(-36.368226956474,38.9096039759392,2.19099528796663));
#23645=CARTESIAN_POINT('Ctrl Pts',(-32.4938580444355,38.2979233002502,2.03399516061437));
#23646=CARTESIAN_POINT('Ctrl Pts',(-30.8667700651969,34.7289638691476,1.87699503326212));
#23647=CARTESIAN_POINT('Ctrl Pts',(-32.9459902326247,31.4030437132317,1.71999490590986));
#23648=CARTESIAN_POINT('Ctrl Pts',(-36.8670582231188,31.3025516345889,1.56299477855761));
#23649=CARTESIAN_POINT('Ctrl Pts',(-39.1139221090429,34.517591201676,1.40599465120536));
#23650=CARTESIAN_POINT('Ctrl Pts',(-37.6717826711976,38.1652229986406,1.2489945238531));
#23651=CARTESIAN_POINT('Ctrl Pts',(-33.8338500234071,38.9745455371789,1.09199439650085));
#23652=CARTESIAN_POINT('Ctrl Pts',(-31.041575077848,36.2199021542904,0.934994269148598));
#23653=CARTESIAN_POINT('Ctrl Pts',(-31.7989386437116,32.3712657534865,0.777994141796342));
#23654=CARTESIAN_POINT('Ctrl Pts',(-35.4265616731752,30.8800320247936,0.620994014444089));
#23655=CARTESIAN_POINT('Ctrl Pts',(-38.6720109988941,33.0828274754107,0.463993887091835));
#23656=CARTESIAN_POINT('Ctrl Pts',(-38.6240716788406,37.0055467263343,0.306993759739582));
#23657=CARTESIAN_POINT('Ctrl Pts',(-35.3277244750448,39.1283073075518,0.149993632387328));
#23658=CARTESIAN_POINT('Ctrl Pts',(-31.734817208837,37.552345230412,-0.00700649496492534));
#23659=CARTESIAN_POINT('Ctrl Pts',(-31.0753017580586,33.6811081626476,-0.164006622317179));
#23660=CARTESIAN_POINT('Ctrl Pts',(-32.9741442474368,31.9005650466595,-0.268673373885348));
#23661=CARTESIAN_POINT('Ctrl Pts',(-34.0915279074966,31.601840982658,-0.321006749669432));
#23662=CARTESIAN_POINT('Ctrl Pts',(-32.1856025125516,37.4062712808594,8.10700224988981));
#23663=CARTESIAN_POINT('Ctrl Pts',(-31.3943716733878,36.4808402609044,8.05466887410573));
#23664=CARTESIAN_POINT('Ctrl Pts',(-30.8087963272068,33.8039236160346,7.95000212253756));
#23665=CARTESIAN_POINT('Ctrl Pts',(-33.6893083541881,30.8387967084451,7.79300199518531));
#23666=CARTESIAN_POINT('Ctrl Pts',(-37.7459632902934,31.614016197849,7.63600186783304));
#23667=CARTESIAN_POINT('Ctrl Pts',(-39.3398463967498,35.4211278497445,7.47900174048081));
#23668=CARTESIAN_POINT('Ctrl Pts',(-37.0423695151407,38.8527626110617,7.32200161312853));
#23669=CARTESIAN_POINT('Ctrl Pts',(-32.9133699266814,38.8285200429468,7.1650014857763));
#23670=CARTESIAN_POINT('Ctrl Pts',(-30.6555263540774,35.3717370910488,7.00800135842403));
#23671=CARTESIAN_POINT('Ctrl Pts',(-32.2933867652647,31.5813506589181,6.85100123107178));
#23672=CARTESIAN_POINT('Ctrl Pts',(-36.3583067411276,30.8566305931499,6.69400110371953));
#23673=CARTESIAN_POINT('Ctrl Pts',(-39.2052133232691,33.8472447317679,6.53700097636727));
#23674=CARTESIAN_POINT('Ctrl Pts',(-38.2812681058037,37.8715777961968,6.38000084901503));
#23675=CARTESIAN_POINT('Ctrl Pts',(-34.4149766453488,39.3209235066531,6.22300072166276));
#23676=CARTESIAN_POINT('Ctrl Pts',(-31.0732820603757,36.8956635970443,6.06600059431052));
#23677=CARTESIAN_POINT('Ctrl Pts',(-31.2527127155268,32.770540011044,5.90900046695826));
#23678=CARTESIAN_POINT('Ctrl Pts',(-34.7923720308581,30.644596543105,5.75200033960601));
#23679=CARTESIAN_POINT('Ctrl Pts',(-38.5182132375505,32.424184166957,5.59500021225375));
#23680=CARTESIAN_POINT('Ctrl Pts',(-39.0892389317987,36.5135310420632,5.43800008490151));
#23681=CARTESIAN_POINT('Ctrl Pts',(-35.9934048207584,39.2456798720372,5.28099995754924));
#23682=CARTESIAN_POINT('Ctrl Pts',(-32.0067750889435,38.1706869484817,5.12399983019699));
#23683=CARTESIAN_POINT('Ctrl Pts',(-30.7041988444697,34.2525085609798,4.96699970284475));
#23684=CARTESIAN_POINT('Ctrl Pts',(-33.2537087112384,31.0046129472743,4.80999957549248));
#23685=CARTESIAN_POINT('Ctrl Pts',(-37.3691347282993,31.3394192191957,4.65299944814024));
#23686=CARTESIAN_POINT('Ctrl Pts',(-39.3601349067833,34.9567034025226,4.49599932078798));
#23687=CARTESIAN_POINT('Ctrl Pts',(-37.4413602847608,38.6128120565681,4.33899919343573));
#23688=CARTESIAN_POINT('Ctrl Pts',(-33.3333944741925,39.0292774815619,4.18199906608348));
#23689=CARTESIAN_POINT('Ctrl Pts',(-30.7198898272843,35.8326511327341,4.02499893873122));
#23690=CARTESIAN_POINT('Ctrl Pts',(-31.9444010336713,31.8893785256963,3.86799881137897));
#23691=CARTESIAN_POINT('Ctrl Pts',(-35.9088971475179,30.7354300360637,3.71099868402671));
#23692=CARTESIAN_POINT('Ctrl Pts',(-39.0583764690558,33.4055623463097,3.55399855667446));
#23693=CARTESIAN_POINT('Ctrl Pts',(-38.5686706776456,37.5054421955447,3.39699842932221));
#23694=CARTESIAN_POINT('Ctrl Pts',(-34.8789036509792,39.3586679946839,3.23999830196995));
#23695=CARTESIAN_POINT('Ctrl Pts',(-31.297724886933,37.3034343822775,3.0829981746177));
#23696=CARTESIAN_POINT('Ctrl Pts',(-31.0364117253094,33.1826890722831,2.92599804726545));
#23697=CARTESIAN_POINT('Ctrl Pts',(-34.3292862136479,30.6915438832177,2.76899791991319));
#23698=CARTESIAN_POINT('Ctrl Pts',(-38.2235961502677,32.0638326727334,2.61199779256094));
#23699=CARTESIAN_POINT('Ctrl Pts',(-39.2272765706619,36.0690107818723,2.45499766520869));
#23700=CARTESIAN_POINT('Ctrl Pts',(-36.440317379388,39.1155968506723,2.29799753785644));
#23701=CARTESIAN_POINT('Ctrl Pts',(-32.3618120906526,38.4716873708438,2.14099741050418));
#23702=CARTESIAN_POINT('Ctrl Pts',(-30.6489945765686,34.714683263722,1.98399728315193));
#23703=CARTESIAN_POINT('Ctrl Pts',(-32.8377666428914,31.2135239126685,1.82699715579967));
#23704=CARTESIAN_POINT('Ctrl Pts',(-36.965431534851,31.1077370132983,1.66999702844742));
#23705=CARTESIAN_POINT('Ctrl Pts',(-39.3306802888702,34.4921735952445,1.51299690109517));
#23706=CARTESIAN_POINT('Ctrl Pts',(-37.8125560580904,38.3319952314996,1.35599677374291));
#23707=CARTESIAN_POINT('Ctrl Pts',(-33.7724068216079,39.1839601136936,1.19899664639066));
#23708=CARTESIAN_POINT('Ctrl Pts',(-30.8330098793911,36.2841775011547,1.04199651903841));
#23709=CARTESIAN_POINT('Ctrl Pts',(-31.6302781259105,32.2327605422985,0.884996391686154));
#23710=CARTESIAN_POINT('Ctrl Pts',(-35.4490367539887,30.6629552947093,0.7279962643339));
#23711=CARTESIAN_POINT('Ctrl Pts',(-38.8654853524014,32.981813694442,0.570996136981647));
#23712=CARTESIAN_POINT('Ctrl Pts',(-38.8150201605686,37.1112168499867,0.413996009629392));
#23713=CARTESIAN_POINT('Ctrl Pts',(-35.3449919290248,39.3458234281866,0.256995882277139));
#23714=CARTESIAN_POINT('Ctrl Pts',(-31.5627782008402,37.6868255855989,0.0999957549248854));
#23715=CARTESIAN_POINT('Ctrl Pts',(-30.8685135825059,33.611617154681,-0.0570043724273683));
#23716=CARTESIAN_POINT('Ctrl Pts',(-32.8674040627957,31.7372591159268,-0.161671123995537));
#23717=CARTESIAN_POINT('Ctrl Pts',(-34.0436614793107,31.4227955987545,-0.214004499779622));
#23718=CARTESIAN_POINT('Ctrl Pts',(-32.0447369588746,37.5267093987113,8.21400449977962));
#23719=CARTESIAN_POINT('Ctrl Pts',(-31.2139036219321,36.5549589254462,8.16167112399554));
#23720=CARTESIAN_POINT('Ctrl Pts',(-30.5990191977949,33.7440578853343,8.05700437242737));
#23721=CARTESIAN_POINT('Ctrl Pts',(-33.6237059276614,30.6305211509797,7.90000424507511));
#23722=CARTESIAN_POINT('Ctrl Pts',(-37.8834035918105,31.4445417418923,7.74300411772286));
#23723=CARTESIAN_POINT('Ctrl Pts',(-39.5570633564287,35.4422060407206,7.58600399037061));
#23724=CARTESIAN_POINT('Ctrl Pts',(-37.1445937083637,39.0456001689453,7.42900386301835));
#23725=CARTESIAN_POINT('Ctrl Pts',(-32.8089304145272,39.0201442175769,7.27200373566611));
#23726=CARTESIAN_POINT('Ctrl Pts',(-30.4380777924235,35.3903431875176,7.11500360831384));
#23727=CARTESIAN_POINT('Ctrl Pts',(-32.1579160033695,31.4102412351758,6.9580034809616));
#23728=CARTESIAN_POINT('Ctrl Pts',(-36.4262923870805,30.6492476530402,6.80100335360934));
#23729=CARTESIAN_POINT('Ctrl Pts',(-39.4156916603747,33.7895472992489,6.64400322625709));
#23730=CARTESIAN_POINT('Ctrl Pts',(-38.4455013566321,38.0153053250877,6.48700309890483));
#23731=CARTESIAN_POINT('Ctrl Pts',(-34.3856951955414,39.5371933423375,6.33000297155258));
#23732=CARTESIAN_POINT('Ctrl Pts',(-30.876742907976,36.9905449005467,6.17300284420033));
#23733=CARTESIAN_POINT('Ctrl Pts',(-31.0651543836038,32.6589516099224,6.01600271684807));
#23734=CARTESIAN_POINT('Ctrl Pts',(-34.781979885128,30.4266009251517,5.85900258949583));
#23735=CARTESIAN_POINT('Ctrl Pts',(-38.694306009759,32.295260045503,5.70200246214356));
#23736=CARTESIAN_POINT('Ctrl Pts',(-39.2939125462453,36.5892859378086,5.54500233479132));
#23737=CARTESIAN_POINT('Ctrl Pts',(-36.0431264825797,39.4581836312174,5.38800220743905));
#23738=CARTESIAN_POINT('Ctrl Pts',(-31.8569589075916,38.3293854175239,5.23100208008681));
#23739=CARTESIAN_POINT('Ctrl Pts',(-30.4891864267288,34.2150952972543,5.07400195273455));
#23740=CARTESIAN_POINT('Ctrl Pts',(-33.166303754984,30.8046367847576,4.9170018253823));
#23741=CARTESIAN_POINT('Ctrl Pts',(-37.487714096255,31.1562007005724,4.76000169803004));
#23742=CARTESIAN_POINT('Ctrl Pts',(-39.578367342141,34.9545363315231,4.60300157067779));
#23743=CARTESIAN_POINT('Ctrl Pts',(-37.5635546690906,38.7936396663671,4.44600144332554));
#23744=CARTESIAN_POINT('Ctrl Pts',(-33.2499779307934,39.2309499197622,4.28900131597329));
#23745=CARTESIAN_POINT('Ctrl Pts',(-30.5056627708833,35.8743267891954,4.13200118862103));
#23746=CARTESIAN_POINT('Ctrl Pts',(-31.7914629209398,31.7336864394819,3.97500106126878));
#23747=CARTESIAN_POINT('Ctrl Pts',(-35.9543890513771,30.5219807944966,3.81800093391652));
#23748=CARTESIAN_POINT('Ctrl Pts',(-39.2615053628575,33.3257579320817,3.66100080656427));
#23749=CARTESIAN_POINT('Ctrl Pts',(-38.747288933645,37.630843992432,3.50400067921202));
#23750=CARTESIAN_POINT('Ctrl Pts',(-34.8728425653191,39.5768270085061,3.34700055185976));
#23751=CARTESIAN_POINT('Ctrl Pts',(-31.1124194935077,37.4187253321399,3.19000042450751));
#23752=CARTESIAN_POINT('Ctrl Pts',(-30.8380271476682,33.0917294579507,3.03300029715526));
#23753=CARTESIAN_POINT('Ctrl Pts',(-34.2957158067332,30.4758980623661,2.87600016980301));
#23754=CARTESIAN_POINT('Ctrl Pts',(-38.3849428180941,31.916872323995,2.71900004245075));
#23755=CARTESIAN_POINT('Ctrl Pts',(-39.4388592121786,36.1225166552775,2.5619999150985));
#23756=CARTESIAN_POINT('Ctrl Pts',(-36.5124078023019,39.3215897254055,2.40499978774625));
#23757=CARTESIAN_POINT('Ctrl Pts',(-32.2297661368697,38.6454514414374,2.24799966039399));
#23758=CARTESIAN_POINT('Ctrl Pts',(-30.4312190879402,34.7004026582963,2.09099953304174));
#23759=CARTESIAN_POINT('Ctrl Pts',(-32.7295430531581,31.0240041121053,1.93399940568948));
#23760=CARTESIAN_POINT('Ctrl Pts',(-37.0638048465832,30.9129223920078,1.77699927833723));
#23761=CARTESIAN_POINT('Ctrl Pts',(-39.5474384686975,34.466755988813,1.61999915098498));
#23762=CARTESIAN_POINT('Ctrl Pts',(-37.9533294449832,38.4987674643586,1.46299902363273));
#23763=CARTESIAN_POINT('Ctrl Pts',(-33.7109636198088,39.3933746902084,1.30599889628047));
#23764=CARTESIAN_POINT('Ctrl Pts',(-30.6244446809342,36.348452848019,1.14899876892822));
#23765=CARTESIAN_POINT('Ctrl Pts',(-31.4616176081094,32.0942553311105,0.991998641575964));
#23766=CARTESIAN_POINT('Ctrl Pts',(-35.4715118348024,30.445878564625,0.834998514223711));
#23767=CARTESIAN_POINT('Ctrl Pts',(-39.0589597059086,32.8807999134734,0.677998386871457));
#23768=CARTESIAN_POINT('Ctrl Pts',(-39.0059686422967,37.2168869736391,0.520998259519203));
#23769=CARTESIAN_POINT('Ctrl Pts',(-35.3622593830049,39.5633395488214,0.36399813216695));
#23770=CARTESIAN_POINT('Ctrl Pts',(-31.3907391928433,37.8213059407857,0.206998004814696));
#23771=CARTESIAN_POINT('Ctrl Pts',(-30.6617254069532,33.5421261467143,0.0499978774624425));
#23772=CARTESIAN_POINT('Ctrl Pts',(-32.7606638781546,31.573953185194,-0.0546688741057264));
#23773=CARTESIAN_POINT('Ctrl Pts',(-33.9957950511247,31.243750214851,-0.107002249889811));
#23774=CARTESIAN_POINT('Ctrl Pts',(-31.9038714051976,37.6471475165632,8.32100674966943));
#23775=CARTESIAN_POINT('Ctrl Pts',(-31.0334355704763,36.629077589988,8.26867337388535));
#23776=CARTESIAN_POINT('Ctrl Pts',(-30.3892420683829,33.6841921546339,8.16400662231718));
#23777=CARTESIAN_POINT('Ctrl Pts',(-33.5581035011348,30.4222455935143,8.00700649496493));
#23778=CARTESIAN_POINT('Ctrl Pts',(-38.0208438933277,31.2750672859355,7.85000636761266));
#23779=CARTESIAN_POINT('Ctrl Pts',(-39.7742803161076,35.4632842316967,7.69300624026044));
#23780=CARTESIAN_POINT('Ctrl Pts',(-37.2468179015868,39.238437726829,7.53600611290815));
#23781=CARTESIAN_POINT('Ctrl Pts',(-32.7044909023729,39.2117683922069,7.37900598555592));
#23782=CARTESIAN_POINT('Ctrl Pts',(-30.2206292307696,35.4089492839864,7.22200585820365));
#23783=CARTESIAN_POINT('Ctrl Pts',(-32.0224452414743,31.2391318114334,7.0650057308514));
#23784=CARTESIAN_POINT('Ctrl Pts',(-36.4942780330333,30.4418647129305,6.90800560349915));
#23785=CARTESIAN_POINT('Ctrl Pts',(-39.6261699974803,33.7318498667299,6.7510054761469));
#23786=CARTESIAN_POINT('Ctrl Pts',(-38.6097346074605,38.1590328539788,6.59400534879465));
#23787=CARTESIAN_POINT('Ctrl Pts',(-34.3564137457339,39.7534631780217,6.4370052214424));
#23788=CARTESIAN_POINT('Ctrl Pts',(-30.6802037555765,37.0854262040492,6.28000509409013));
#23789=CARTESIAN_POINT('Ctrl Pts',(-30.8775960516807,32.5473632088007,6.12300496673789));
#23790=CARTESIAN_POINT('Ctrl Pts',(-34.7715877393978,30.2086053071985,5.96600483938563));
#23791=CARTESIAN_POINT('Ctrl Pts',(-38.8703987819675,32.166335924049,5.80900471203337));
#23792=CARTESIAN_POINT('Ctrl Pts',(-39.4985861606919,36.6650408335539,5.65200458468113));
#23793=CARTESIAN_POINT('Ctrl Pts',(-36.092848144401,39.6706873903976,5.49500445732886));
#23794=CARTESIAN_POINT('Ctrl Pts',(-31.7071427262397,38.4880838865661,5.33800432997662));
#23795=CARTESIAN_POINT('Ctrl Pts',(-30.2741740089879,34.1776820335287,5.18100420262436));
#23796=CARTESIAN_POINT('Ctrl Pts',(-33.0788987987297,30.6046606222411,5.02400407527212));
#23797=CARTESIAN_POINT('Ctrl Pts',(-37.6062934642105,30.9729821819491,4.86700394791985));
#23798=CARTESIAN_POINT('Ctrl Pts',(-39.7965997774987,34.9523692605237,4.7100038205676));
#23799=CARTESIAN_POINT('Ctrl Pts',(-37.6857490534203,38.974467276166,4.55300369321535));
#23800=CARTESIAN_POINT('Ctrl Pts',(-33.1665613873943,39.4326223579625,4.3960035658631));
#23801=CARTESIAN_POINT('Ctrl Pts',(-30.2914357144823,35.9160024456566,4.23900343851084));
#23802=CARTESIAN_POINT('Ctrl Pts',(-31.6385248082081,31.5779943532675,4.08200331115859));
#23803=CARTESIAN_POINT('Ctrl Pts',(-35.9998809552364,30.3085315529294,3.92500318380634));
#23804=CARTESIAN_POINT('Ctrl Pts',(-39.464634256659,33.2459535178537,3.76800305645409));
#23805=CARTESIAN_POINT('Ctrl Pts',(-38.9259071896446,37.7562457893193,3.61100292910183));
#23806=CARTESIAN_POINT('Ctrl Pts',(-34.866781479659,39.7949860223284,3.45400280174958));
#23807=CARTESIAN_POINT('Ctrl Pts',(-30.9271141000824,37.5340162820022,3.29700267439732));
#23808=CARTESIAN_POINT('Ctrl Pts',(-30.6396425700269,33.0007698436185,3.14000254704507));
#23809=CARTESIAN_POINT('Ctrl Pts',(-34.2621453998186,30.2602522415144,2.98300241969281));
#23810=CARTESIAN_POINT('Ctrl Pts',(-38.5462894859204,31.7699119752566,2.82600229234057));
#23811=CARTESIAN_POINT('Ctrl Pts',(-39.6504418536953,36.1760225286826,2.66900216498831));
#23812=CARTESIAN_POINT('Ctrl Pts',(-36.5844982252159,39.5275826001387,2.51200203763606));
#23813=CARTESIAN_POINT('Ctrl Pts',(-32.0977201830868,38.819215512031,2.3550019102838));
#23814=CARTESIAN_POINT('Ctrl Pts',(-30.2134435993119,34.6861220528707,2.19800178293155));
#23815=CARTESIAN_POINT('Ctrl Pts',(-32.6213194634248,30.8344843115421,2.04100165557929));
#23816=CARTESIAN_POINT('Ctrl Pts',(-37.1621781583154,30.7181077707172,1.88400152822704));
#23817=CARTESIAN_POINT('Ctrl Pts',(-39.7641966485248,34.4413383823816,1.72700140087479));
#23818=CARTESIAN_POINT('Ctrl Pts',(-38.0941028318759,38.6655396972175,1.57000127352254));
#23819=CARTESIAN_POINT('Ctrl Pts',(-33.6495204180096,39.602789266723,1.41300114617028));
#23820=CARTESIAN_POINT('Ctrl Pts',(-30.4158794824773,36.4127281948833,1.25600101881803));
#23821=CARTESIAN_POINT('Ctrl Pts',(-31.2929570903083,31.9557501199225,1.09900089146578));
#23822=CARTESIAN_POINT('Ctrl Pts',(-35.4939869156159,30.2288018345407,0.942000764113521));
#23823=CARTESIAN_POINT('Ctrl Pts',(-39.2524340594159,32.7797861325047,0.785000636761268));
#23824=CARTESIAN_POINT('Ctrl Pts',(-39.1969171240247,37.3225570972915,0.628000509409013));
#23825=CARTESIAN_POINT('Ctrl Pts',(-35.379526836985,39.7808556694562,0.471000382056761));
#23826=CARTESIAN_POINT('Ctrl Pts',(-31.2187001848465,37.9557862959725,0.314000254704507));
#23827=CARTESIAN_POINT('Ctrl Pts',(-30.4549372314006,33.4726351387477,0.157000127352253));
#23828=CARTESIAN_POINT('Ctrl Pts',(-32.6539236935135,31.4106472544613,0.0523333757840845));
#23829=CARTESIAN_POINT('Ctrl Pts',(-33.9479286229388,31.0647048309474,0.));
#23830=CARTESIAN_POINT('Ctrl Pts',(-33.9479286229388,31.0647048309474,0.));
#23831=CARTESIAN_POINT('Ctrl Pts',(-33.8318205444026,31.104319484649,-6.12910217551102E-18));
#23832=CARTESIAN_POINT('Ctrl Pts',(-33.7179775273608,31.1494845452793,-1.6976040424202E-15));
#23833=CARTESIAN_POINT('Ctrl Pts',(-33.6066254658749,31.1998424056554,-1.16573417585641E-15));
#23834=CARTESIAN_POINT('Ctrl Pts',(-33.4927762352539,31.2513295858929,-6.21936653918048E-16));
#23835=CARTESIAN_POINT('Ctrl Pts',(-33.3815303134372,31.3082455820535,1.45039252013455E-15));
#23836=CARTESIAN_POINT('Ctrl Pts',(-33.2731534080755,31.3702567597409,9.99200722162641E-16));
#23837=CARTESIAN_POINT('Ctrl Pts',(-33.1592150345376,31.4354501023936,5.24855570462807E-16));
#23838=CARTESIAN_POINT('Ctrl Pts',(-33.0484467137175,31.5062753971616,-4.62145718692395E-16));
#23839=CARTESIAN_POINT('Ctrl Pts',(-32.9411963534997,31.5823911623814,-5.55111512312578E-16));
#23840=CARTESIAN_POINT('Ctrl Pts',(-32.8473522883091,31.6489924569487,-6.36456581730239E-16));
#23841=CARTESIAN_POINT('Ctrl Pts',(-32.7562019661932,31.7196453256574,-1.95036301750383E-15));
#23842=CARTESIAN_POINT('Ctrl Pts',(-32.6680099559688,31.7941431443398,-1.99840144432528E-15));
#23843=CARTESIAN_POINT('Ctrl Pts',(-32.6506336549248,31.8088213053349,-2.00786636256454E-15));
#23844=CARTESIAN_POINT('Ctrl Pts',(-32.6333722976869,31.8236487792666,-7.57847684029515E-16));
#23845=CARTESIAN_POINT('Ctrl Pts',(-32.6162280624477,31.8386240567023,-7.7715611723761E-16));
#23846=CARTESIAN_POINT('Ctrl Pts',(-32.6036937742642,31.8495726024021,-7.91272667951259E-16));
#23847=CARTESIAN_POINT('Ctrl Pts',(-32.5912233028683,31.8605991578939,4.81364284937086E-16));
#23848=CARTESIAN_POINT('Ctrl Pts',(-32.5788262971356,31.8716950114967,4.44089209850063E-16));
#23849=CARTESIAN_POINT('Ctrl Pts',(-32.4862471134748,31.9545573647705,1.6572392577578E-16));
#23850=CARTESIAN_POINT('Ctrl Pts',(-32.3976237822216,32.0414014202655,8.13390076176465E-16));
#23851=CARTESIAN_POINT('Ctrl Pts',(-32.3132177297223,32.1319062612438,6.38378239159465E-16));
#23852=CARTESIAN_POINT('Ctrl Pts',(-32.2290034543674,32.222205468154,4.63764042706654E-16));
#23853=CARTESIAN_POINT('Ctrl Pts',(-32.1489867981842,32.3161495489862,3.17588722629917E-16));
#23854=CARTESIAN_POINT('Ctrl Pts',(-32.0734678385385,32.4134518063003,8.88178419700125E-16));
#23855=CARTESIAN_POINT('Ctrl Pts',(-31.9989812077255,32.5094239615292,1.4509682715575E-15));
#23856=CARTESIAN_POINT('Ctrl Pts',(-31.9288697495096,32.6086637947563,-1.05272258015246E-15));
#23857=CARTESIAN_POINT('Ctrl Pts',(-31.8634674410238,32.710917033623,-1.02695629777827E-15));
#23858=CARTESIAN_POINT('Ctrl Pts',(-31.8101619976839,32.7942574287394,-1.00595576833249E-15));
#23859=CARTESIAN_POINT('Ctrl Pts',(-31.7599855228772,32.8796001211512,6.44886685271164E-16));
#23860=CARTESIAN_POINT('Ctrl Pts',(-31.7131447814318,32.9668132818295,6.10622663543836E-16));
#23861=CARTESIAN_POINT('Ctrl Pts',(-31.7012439418187,32.9889715527142,6.01917194448022E-16));
#23862=CARTESIAN_POINT('Ctrl Pts',(-31.6895585553312,33.0112505813609,1.19774783640231E-15));
#23863=CARTESIAN_POINT('Ctrl Pts',(-31.6780922762038,33.0336482309453,1.16573417585641E-15));
#23864=CARTESIAN_POINT('Ctrl Pts',(-31.6699364387253,33.0495794312833,1.14296321331454E-15));
#23865=CARTESIAN_POINT('Ctrl Pts',(-31.661895167037,33.0655634624947,-2.51368181031482E-15));
#23866=CARTESIAN_POINT('Ctrl Pts',(-31.6539721233883,33.0815939077556,-2.4980018054066E-15));
#23867=CARTESIAN_POINT('Ctrl Pts',(-31.6010112907938,33.1887478962384,-2.3931903021702E-15));
#23868=CARTESIAN_POINT('Ctrl Pts',(-31.5532893085976,33.2980517601776,-1.33576692347369E-15));
#23869=CARTESIAN_POINT('Ctrl Pts',(-31.5110849763849,33.409242888583,-1.0547118733939E-15));
#23870=CARTESIAN_POINT('Ctrl Pts',(-31.469716801377,33.5182310852453,-7.79225119096594E-16));
#23871=CARTESIAN_POINT('Ctrl Pts',(-31.4336495378063,33.6290331387016,-1.04560375035282E-15));
#23872=CARTESIAN_POINT('Ctrl Pts',(-31.4031939533011,33.7414155242157,-1.19348975147204E-15));
#23873=CARTESIAN_POINT('Ctrl Pts',(-31.3987398005021,33.7578515350533,-1.2151181935629E-15));
#23874=CARTESIAN_POINT('Ctrl Pts',(-31.3944057673546,33.7743213630571,-1.05328088726205E-15));
#23875=CARTESIAN_POINT('Ctrl Pts',(-31.390192920076,33.7908242908111,-1.11022302462516E-15));
#23876=CARTESIAN_POINT('Ctrl Pts',(-31.3605243708329,33.9070444840312,-1.45504712955035E-15));
#23877=CARTESIAN_POINT('Ctrl Pts',(-31.336861805495,34.0249066128039,2.32711961845814E-15));
#23878=CARTESIAN_POINT('Ctrl Pts',(-31.3191143685546,34.1439748333396,2.41473507855972E-15));
#23879=CARTESIAN_POINT('Ctrl Pts',(-31.3091308324304,34.2109547519018,2.46402175098999E-15));
#23880=CARTESIAN_POINT('Ctrl Pts',(-31.3010200590003,34.2783162816674,1.31577829093223E-15));
#23881=CARTESIAN_POINT('Ctrl Pts',(-31.2947729234008,34.3459803828548,1.66533453693773E-15));
#23882=CARTESIAN_POINT('Ctrl Pts',(-31.2918904510582,34.3772010754682,1.82662224956662E-15));
#23883=CARTESIAN_POINT('Ctrl Pts',(-31.2894048093972,34.4084861625173,5.36743605776751E-16));
#23884=CARTESIAN_POINT('Ctrl Pts',(-31.2873154495445,34.4398277448617,5.55111512312578E-16));
#23885=CARTESIAN_POINT('Ctrl Pts',(-31.2861143588149,34.4578447867584,5.6567049870877E-16));
#23886=CARTESIAN_POINT('Ctrl Pts',(-31.2850447395365,34.4758734447918,-4.83710549279582E-16));
#23887=CARTESIAN_POINT('Ctrl Pts',(-31.2841065224407,34.4939038782769,-4.44089209850063E-16));
#23888=CARTESIAN_POINT('Ctrl Pts',(-31.2777956059898,34.6151855728967,-1.77576305814986E-16));
#23889=CARTESIAN_POINT('Ctrl Pts',(-31.2774172190669,34.7366645735772,1.74591754833025E-15));
#23890=CARTESIAN_POINT('Ctrl Pts',(-31.2828131531898,34.8578936251582,1.77635683940025E-15));
#23891=CARTESIAN_POINT('Ctrl Pts',(-31.2880971535264,34.9766078894115,1.80616469483294E-15));
#23892=CARTESIAN_POINT('Ctrl Pts',(-31.2989188936952,35.0950833906807,2.23513941723243E-15));
#23893=CARTESIAN_POINT('Ctrl Pts',(-31.3151831802674,35.2128941454877,2.73392419813945E-15));
#23894=CARTESIAN_POINT('Ctrl Pts',(-31.3312885576294,35.3295538375714,3.22783563306706E-15));
#23895=CARTESIAN_POINT('Ctrl Pts',(-31.3527309988427,35.445562546077,2.65572620552751E-15));
#23896=CARTESIAN_POINT('Ctrl Pts',(-31.3794648565834,35.5604877518601,3.06699110552699E-15));
#23897=CARTESIAN_POINT('Ctrl Pts',(-31.3968717688464,35.6353176919788,3.33477333511016E-15));
#23898=CARTESIAN_POINT('Ctrl Pts',(-31.4165229425865,35.7096878616141,5.4636862845821E-16));
#23899=CARTESIAN_POINT('Ctrl Pts',(-31.4384155780607,35.7834719630247,4.85722573273506E-16));
#23900=CARTESIAN_POINT('Ctrl Pts',(-31.4458039236167,35.8083726853891,4.65255690113341E-16));
#23901=CARTESIAN_POINT('Ctrl Pts',(-31.45344761912,35.8332066040146,2.20922363074103E-15));
#23902=CARTESIAN_POINT('Ctrl Pts',(-31.4613467446,35.8579686875435,2.27595720048157E-15));
#23903=CARTESIAN_POINT('Ctrl Pts',(-31.4664331437066,35.8739134702743,2.31892823194254E-15));
#23904=CARTESIAN_POINT('Ctrl Pts',(-31.4716246609433,35.8898258563265,-1.15821499265833E-16));
#23905=CARTESIAN_POINT('Ctrl Pts',(-31.4769184371132,35.9056964793841,2.77555756156289E-17));
#23906=CARTESIAN_POINT('Ctrl Pts',(-31.5138161242914,36.0163149237837,1.02848961215397E-15));
#23907=CARTESIAN_POINT('Ctrl Pts',(-31.5557145226016,36.1250218909898,1.27042107846669E-15));
#23908=CARTESIAN_POINT('Ctrl Pts',(-31.6025488384922,36.2313981798515,1.95676808090184E-15));
#23909=CARTESIAN_POINT('Ctrl Pts',(-31.6406629331589,36.3179679496208,2.51532208404033E-15));
#23910=CARTESIAN_POINT('Ctrl Pts',(-31.6820469345646,36.4029939678578,-2.48735046316874E-16));
#23911=CARTESIAN_POINT('Ctrl Pts',(-31.7266869042645,36.4862346415976,-4.02455846426619E-16));
#23912=CARTESIAN_POINT('Ctrl Pts',(-31.748301897583,36.5265403725114,-4.76888559747074E-16));
#23913=CARTESIAN_POINT('Ctrl Pts',(-31.7706805448521,36.566427275075,1.22980137611631E-15));
#23914=CARTESIAN_POINT('Ctrl Pts',(-31.7938227368542,36.6058663963511,1.14491749414469E-15));
#23915=CARTESIAN_POINT('Ctrl Pts',(-31.8074091619825,36.6290204981016,1.09508347207335E-15));
#23916=CARTESIAN_POINT('Ctrl Pts',(-31.8212608195948,36.6520233300662,-7.62339319688486E-16));
#23917=CARTESIAN_POINT('Ctrl Pts',(-31.8353636346369,36.6748465408533,-5.68989300120393E-16));
#23918=CARTESIAN_POINT('Ctrl Pts',(-31.8937950765752,36.7694087337193,2.32107531151829E-16));
#23919=CARTESIAN_POINT('Ctrl Pts',(-31.9565777772527,36.8609657133175,3.78686475409805E-16));
#23920=CARTESIAN_POINT('Ctrl Pts',(-32.0236776904421,36.9491267660533,4.5102810375397E-17));
#23921=CARTESIAN_POINT('Ctrl Pts',(-32.0837084847486,37.0279998639616,-2.53337104489111E-16));
#23922=CARTESIAN_POINT('Ctrl Pts',(-32.1471953789829,37.1041548289018,-7.94184032652028E-16));
#23923=CARTESIAN_POINT('Ctrl Pts',(-32.2141374826654,37.1772853486058,-1.07986536379556E-15));
#23924=CARTESIAN_POINT('Ctrl Pts',(-32.2489924160368,37.2153624219495,-1.21791469682805E-15));
#23925=CARTESIAN_POINT('Ctrl Pts',(-32.2847844521695,37.2526190806637,6.40917790468134E-17));
#23926=CARTESIAN_POINT('Ctrl Pts',(-32.3214761820288,37.2890399271606,-2.77555756156289E-17));
#23927=CARTESIAN_POINT('Ctrl Pts',(-38.5163029138352,34.997016742257,6.38741669750802));
#23928=CARTESIAN_POINT('Ctrl Pts',(-38.5189470194328,34.6831064778252,6.4016107071645));
#23929=CARTESIAN_POINT('Ctrl Pts',(-38.4802904146781,34.3698362574768,6.41580471682098));
#23930=CARTESIAN_POINT('Ctrl Pts',(-38.3977159824674,34.0686054096188,6.42999872647747));
#23931=CARTESIAN_POINT('Ctrl Pts',(-38.0932636891673,32.9579659539444,6.48233210226155));
#23932=CARTESIAN_POINT('Ctrl Pts',(-37.1917923921711,32.010989743602,6.53466547804563));
#23933=CARTESIAN_POINT('Ctrl Pts',(-36.0974794823371,31.6522427299976,6.58699885382972));
#23934=CARTESIAN_POINT('Ctrl Pts',(-35.0031665725032,31.2934957163932,6.6393322296138));
#23935=CARTESIAN_POINT('Ctrl Pts',(-33.7160120498315,31.5229778995268,6.69166560539789));
#23936=CARTESIAN_POINT('Ctrl Pts',(-32.8131210199243,32.2378308097469,6.74399898118197));
#23937=CARTESIAN_POINT('Ctrl Pts',(-31.9102299900171,32.952683719967,6.79633235696605));
#23938=CARTESIAN_POINT('Ctrl Pts',(-31.3916024528742,34.1529073572735,6.84866573275014));
#23939=CARTESIAN_POINT('Ctrl Pts',(-31.4897611048202,35.3003133215496,6.90099910853422));
#23940=CARTESIAN_POINT('Ctrl Pts',(-31.5879197567661,36.4477192858256,6.95333248431831));
#23941=CARTESIAN_POINT('Ctrl Pts',(-32.3028645978009,37.5423075770711,7.00566586010239));
#23942=CARTESIAN_POINT('Ctrl Pts',(-33.3140596654986,38.0934399201708,7.05799923588648));
#23943=CARTESIAN_POINT('Ctrl Pts',(-34.3252547331963,38.6445722632704,7.11033261167056));
#23944=CARTESIAN_POINT('Ctrl Pts',(-35.6327000275569,38.6522486582243,7.16266598745464));
#23945=CARTESIAN_POINT('Ctrl Pts',(-36.6501700272628,38.1127742899662,7.21499936323873));
#23946=CARTESIAN_POINT('Ctrl Pts',(-37.6676400269687,37.5732999217082,7.26733273902281));
#23947=CARTESIAN_POINT('Ctrl Pts',(-38.3951347320199,36.4866747902383,7.3196661148069));
#23948=CARTESIAN_POINT('Ctrl Pts',(-38.5065310098296,35.3406023903429,7.37199949059099));
#23949=CARTESIAN_POINT('Ctrl Pts',(-38.5174699784391,35.2280595814352,7.37713855956333));
#23950=CARTESIAN_POINT('Ctrl Pts',(-38.5224679204996,35.1149435235394,7.38227762853568));
#23951=CARTESIAN_POINT('Ctrl Pts',(-38.521739013009,35.0017650567249,7.38741669750802));
#23952=CARTESIAN_POINT('Ctrl Pts',(-36.0520713770612,31.0647048309474,8.));
#23953=CARTESIAN_POINT('Ctrl Pts',(-37.3460763064866,31.4106472544613,7.94766662421592));
#23954=CARTESIAN_POINT('Ctrl Pts',(-39.5450624630061,33.4726371160361,7.84299987264775));
#23955=CARTESIAN_POINT('Ctrl Pts',(-38.7813000795415,37.9557855546777,7.6859997452955));
#23956=CARTESIAN_POINT('Ctrl Pts',(-34.6204731393245,39.7808563212243,7.52899961794324));
#23957=CARTESIAN_POINT('Ctrl Pts',(-30.8030827008644,37.3225569109026,7.37199949059099));
#23958=CARTESIAN_POINT('Ctrl Pts',(-30.7475658132336,32.7797862032913,7.21499936323873));
#23959=CARTESIAN_POINT('Ctrl Pts',(-34.5060130464714,30.2288015790917,7.05799923588648));
#23960=CARTESIAN_POINT('Ctrl Pts',(-38.707043056971,31.9557500555838,6.90099910853422));
#23961=CARTESIAN_POINT('Ctrl Pts',(-39.5841206744658,36.4127282212004,6.74399898118198));
#23962=CARTESIAN_POINT('Ctrl Pts',(-36.3504796357983,39.6027894460767,6.58699885382972));
#23963=CARTESIAN_POINT('Ctrl Pts',(-31.905897053523,38.6655398223873,6.42999872647746));
#23964=CARTESIAN_POINT('Ctrl Pts',(-30.2358031812474,34.4413383659989,6.27299859912522));
#23965=CARTESIAN_POINT('Ctrl Pts',(-32.8378217627235,30.7181076142107,6.11599847177296));
#23966=CARTESIAN_POINT('Ctrl Pts',(-37.3786806229274,30.8344841622903,5.95899834442071));
#23967=CARTESIAN_POINT('Ctrl Pts',(-39.7865565731199,34.68612204099,5.80199821706845));
#23968=CARTESIAN_POINT('Ctrl Pts',(-37.9022799217924,38.8192156501332,5.6449980897162));
#23969=CARTESIAN_POINT('Ctrl Pts',(-33.4155017175264,39.5275827633586,5.48799796236395));
#23970=CARTESIAN_POINT('Ctrl Pts',(-30.3495579785441,36.176022571197,5.33099783501169));
#23971=CARTESIAN_POINT('Ctrl Pts',(-31.4537103860929,31.7699118586619,5.17399770765944));
#23972=CARTESIAN_POINT('Ctrl Pts',(-35.7378546268185,30.2602520705083,5.01699758030719));
#23973=CARTESIAN_POINT('Ctrl Pts',(-39.3603575873042,33.0007697714678,4.85999745295493));
#23974=CARTESIAN_POINT('Ctrl Pts',(-39.0728860468858,37.5340163734447,4.70299732560268));
#23975=CARTESIAN_POINT('Ctrl Pts',(-35.1332185251462,39.7949861953461,4.54599719825043));
#23976=CARTESIAN_POINT('Ctrl Pts',(-31.0740926686951,37.7562458887763,4.38899707089817));
#23977=CARTESIAN_POINT('Ctrl Pts',(-30.5353655822401,33.2459534545604,4.23199694354592));
#23978=CARTESIAN_POINT('Ctrl Pts',(-34.0001190086845,30.3085313836444,4.07499681619366));
#23979=CARTESIAN_POINT('Ctrl Pts',(-38.3614753130862,31.5779942297887,3.91799668884141));
#23980=CARTESIAN_POINT('Ctrl Pts',(-39.70856445542,35.9160024787098,3.76099656148916));
#23981=CARTESIAN_POINT('Ctrl Pts',(-36.8334386787628,39.4326225179073,3.6039964341369));
#23982=CARTESIAN_POINT('Ctrl Pts',(-32.314250849668,38.9744674195804,3.44699630678465));
#23983=CARTESIAN_POINT('Ctrl Pts',(-30.2034000494222,34.9523692588031,3.2899961794324));
#23984=CARTESIAN_POINT('Ctrl Pts',(-32.3937064417451,30.9729820366429,3.13299605208014));
#23985=CARTESIAN_POINT('Ctrl Pts',(-36.9211012705904,30.6046604636344,2.97599592472789));
#23986=CARTESIAN_POINT('Ctrl Pts',(-39.7258261615381,34.1776820038694,2.81899579737564));
#23987=CARTESIAN_POINT('Ctrl Pts',(-38.2928573925768,38.4880840124043,2.66199567002338));
#23988=CARTESIAN_POINT('Ctrl Pts',(-33.9071518161688,39.6706875589806,2.50499554267113));
#23989=CARTESIAN_POINT('Ctrl Pts',(-30.5014136769744,36.6650408935442,2.34799541531887));
#23990=CARTESIAN_POINT('Ctrl Pts',(-31.1296010783918,32.1663358219723,2.19099528796663));
#23991=CARTESIAN_POINT('Ctrl Pts',(-35.2284122688067,30.2086051339802,2.03399516061437));
#23992=CARTESIAN_POINT('Ctrl Pts',(-39.1224040971504,32.5473631209192,1.87699503326212));
#23993=CARTESIAN_POINT('Ctrl Pts',(-39.319796400129,37.0854262781345,1.71999490590986));
#23994=CARTESIAN_POINT('Ctrl Pts',(-35.6435862778458,39.7534633517259,1.56299477855761));
#23995=CARTESIAN_POINT('Ctrl Pts',(-31.3902652615342,38.1590329639038,1.40599465120536));
#23996=CARTESIAN_POINT('Ctrl Pts',(-30.3738298371754,33.7318498284919,1.2489945238531));
#23997=CARTESIAN_POINT('Ctrl Pts',(-33.5057219097166,30.4418645346457,1.09199439650085));
#23998=CARTESIAN_POINT('Ctrl Pts',(-37.9775548729557,31.2391317008465,0.934994269148598));
#23999=CARTESIAN_POINT('Ctrl Pts',(-39.7793709270477,35.4089492535829,0.777994141796342));
#24000=CARTESIAN_POINT('Ctrl Pts',(-37.2955092110801,39.2117686241983,0.620994014444089));
#24001=CARTESIAN_POINT('Ctrl Pts',(-32.7531819533668,39.2384377406302,0.463993887091835));
#24002=CARTESIAN_POINT('Ctrl Pts',(-30.2257196451616,35.46328448449,0.306993759739582));
#24003=CARTESIAN_POINT('Ctrl Pts',(-31.9791557179606,31.2750667622313,0.149993632387329));
#24004=CARTESIAN_POINT('Ctrl Pts',(-36.4418971366481,30.4222460546565,-0.00700649496492604));
#24005=CARTESIAN_POINT('Ctrl Pts',(-39.6107565597589,33.6841906982476,-0.164006622317178));
#24006=CARTESIAN_POINT('Ctrl Pts',(-38.9665644295237,36.6290775899881,-0.268673373885348));
#24007=CARTESIAN_POINT('Ctrl Pts',(-38.0961285948024,37.6471475165632,-0.321006749669432));
#24008=CARTESIAN_POINT('Ctrl Pts',(-36.0042049488753,31.243750214851,8.10700224988981));
#24009=CARTESIAN_POINT('Ctrl Pts',(-37.2393361218455,31.5739531851941,8.05466887410573));
#24010=CARTESIAN_POINT('Ctrl Pts',(-39.3382743013571,33.5421280340415,7.95000212253756));
#24011=CARTESIAN_POINT('Ctrl Pts',(-38.6092610595157,37.8213052332178,7.79300199518531));
#24012=CARTESIAN_POINT('Ctrl Pts',(-34.6377405943825,39.5633401709358,7.63600186783305));
#24013=CARTESIAN_POINT('Ctrl Pts',(-30.9940311905596,37.2168867957304,7.4790017404808));
#24014=CARTESIAN_POINT('Ctrl Pts',(-30.941040172535,32.8807999810394,7.32200161312854));
#24015=CARTESIAN_POINT('Ctrl Pts',(-34.5284881290099,30.4458783207982,7.16500148577629));
#24016=CARTESIAN_POINT('Ctrl Pts',(-38.5383825324691,32.0942552696991,7.00800135842404));
#24017=CARTESIAN_POINT('Ctrl Pts',(-39.3755554688683,36.3484528731387,6.85100123107178));
#24018=CARTESIAN_POINT('Ctrl Pts',(-36.2890364315511,39.3933748614019,6.69400110371953));
#24019=CARTESIAN_POINT('Ctrl Pts',(-32.0466704456298,38.4987675838335,6.53700097636727));
#24020=CARTESIAN_POINT('Ctrl Pts',(-30.4525613688197,34.4667559731757,6.38000084901503));
#24021=CARTESIAN_POINT('Ctrl Pts',(-32.9361950780481,30.9129222426219,6.22300072166277));
#24022=CARTESIAN_POINT('Ctrl Pts',(-37.2704570292653,31.024003969644,6.06600059431052));
#24023=CARTESIAN_POINT('Ctrl Pts',(-39.5687810766463,34.7004026469562,5.90900046695827));
#24024=CARTESIAN_POINT('Ctrl Pts',(-37.7702339632379,38.6454515732563,5.752000339606));
#24025=CARTESIAN_POINT('Ctrl Pts',(-33.4875921430454,39.3215898811993,5.59500021225376));
#24026=CARTESIAN_POINT('Ctrl Pts',(-30.5611406276935,36.1225166958576,5.4380000849015));
#24027=CARTESIAN_POINT('Ctrl Pts',(-31.6150570597422,31.916872212705,5.28099995754925));
#24028=CARTESIAN_POINT('Ctrl Pts',(-35.7042842186919,30.4758978991403,5.123999830197));
#24029=CARTESIAN_POINT('Ctrl Pts',(-39.1619730025048,33.0917293890828,4.96699970284474));
#24030=CARTESIAN_POINT('Ctrl Pts',(-38.8875806467738,37.4187254194219,4.80999957549249));
#24031=CARTESIAN_POINT('Ctrl Pts',(-35.1271574392675,39.576827173652,4.65299944814024));
#24032=CARTESIAN_POINT('Ctrl Pts',(-31.2527109311398,37.6308440873639,4.49599932078798));
#24033=CARTESIAN_POINT('Ctrl Pts',(-30.7384944833714,33.3257578716681,4.33899919343573));
#24034=CARTESIAN_POINT('Ctrl Pts',(-34.0456109141852,30.5219806329136,4.18199906608347));
#24035=CARTESIAN_POINT('Ctrl Pts',(-38.208537194836,31.7336863216211,4.02499893873123));
#24036=CARTESIAN_POINT('Ctrl Pts',(-39.4943373912889,35.8743268207447,3.86799881137897));
#24037=CARTESIAN_POINT('Ctrl Pts',(-36.7500221323538,39.23095007243,3.71099868402672));
#24038=CARTESIAN_POINT('Ctrl Pts',(-32.4364452384069,38.7936398032564,3.55399855667446));
#24039=CARTESIAN_POINT('Ctrl Pts',(-30.4216324926546,34.9545363298808,3.39699842932221));
#24040=CARTESIAN_POINT('Ctrl Pts',(-32.5122858139794,31.1562005618773,3.23999830196995));
#24041=CARTESIAN_POINT('Ctrl Pts',(-36.8336963111821,30.8046366333671,3.0829981746177));
#24042=CARTESIAN_POINT('Ctrl Pts',(-39.5108137360388,34.2150952689444,2.92599804726545));
#24043=CARTESIAN_POINT('Ctrl Pts',(-38.1430412058191,38.3293855376367,2.7689979199132));
#24044=CARTESIAN_POINT('Ctrl Pts',(-33.9568734797841,39.4581837921304,2.61199779256094));
#24045=CARTESIAN_POINT('Ctrl Pts',(-30.7060872988067,36.5892859950694,2.45499766520869));
#24046=CARTESIAN_POINT('Ctrl Pts',(-31.3056938569536,32.2952599480705,2.29799753785643));
#24047=CARTESIAN_POINT('Ctrl Pts',(-35.2180201227033,30.4266007598144,2.14099741050418));
#24048=CARTESIAN_POINT('Ctrl Pts',(-38.9348457584559,32.6589515260392,1.98399728315193));
#24049=CARTESIAN_POINT('Ctrl Pts',(-39.1232572406452,36.9905449712614,1.82699715579967));
#24050=CARTESIAN_POINT('Ctrl Pts',(-35.6143048269655,39.5371935081385,1.66999702844742));
#24051=CARTESIAN_POINT('Ctrl Pts',(-31.554498518323,38.0153054300115,1.51299690109517));
#24052=CARTESIAN_POINT('Ctrl Pts',(-30.5843081818037,33.7895472627506,1.35599677374291));
#24053=CARTESIAN_POINT('Ctrl Pts',(-33.5737075582741,30.6492474828669,1.19899664639066));
#24054=CARTESIAN_POINT('Ctrl Pts',(-37.8420841058543,31.4102411296202,1.04199651903841));
#24055=CARTESIAN_POINT('Ctrl Pts',(-39.5619223582134,35.3903431584975,0.884996391686153));
#24056=CARTESIAN_POINT('Ctrl Pts',(-37.1910696937641,39.0201444390132,0.7279962643339));
#24057=CARTESIAN_POINT('Ctrl Pts',(-32.8554061531891,39.0456001821187,0.570996136981647));
#24058=CARTESIAN_POINT('Ctrl Pts',(-30.4429366066027,35.4422062820125,0.413996009629392));
#24059=CARTESIAN_POINT('Ctrl Pts',(-32.116596037163,31.4445412420153,0.25699588227714));
#24060=CARTESIAN_POINT('Ctrl Pts',(-36.3762946811041,30.6305215911411,0.0999957549248848));
#24061=CARTESIAN_POINT('Ctrl Pts',(-39.4009794927627,33.7440564952096,-0.057004372427367));
#24062=CARTESIAN_POINT('Ctrl Pts',(-38.7860963780679,36.5549589254462,-0.161671123995537));
#24063=CARTESIAN_POINT('Ctrl Pts',(-37.9552630411254,37.5267093987113,-0.214004499779622));
#24064=CARTESIAN_POINT('Ctrl Pts',(-35.9563385206894,31.4227955987545,8.21400449977962));
#24065=CARTESIAN_POINT('Ctrl Pts',(-37.1325959372044,31.7372591159268,8.16167112399554));
#24066=CARTESIAN_POINT('Ctrl Pts',(-39.1314861397082,33.6116189520467,8.05700437242738));
#24067=CARTESIAN_POINT('Ctrl Pts',(-38.4372220394899,37.6868249117579,7.90000424507511));
#24068=CARTESIAN_POINT('Ctrl Pts',(-34.6550080494404,39.3458240206473,7.74300411772287));
#24069=CARTESIAN_POINT('Ctrl Pts',(-31.1849796802547,37.1112166805582,7.5860039903706));
#24070=CARTESIAN_POINT('Ctrl Pts',(-31.1345145318363,32.9818137587874,7.42900386301836));
#24071=CARTESIAN_POINT('Ctrl Pts',(-34.5509632115484,30.6629550625048,7.2720037356661));
#24072=CARTESIAN_POINT('Ctrl Pts',(-38.3697220079671,32.2327604838143,7.11500360831385));
#24073=CARTESIAN_POINT('Ctrl Pts',(-39.166990263271,36.2841775250771,6.95800348096159));
#24074=CARTESIAN_POINT('Ctrl Pts',(-36.2275932273038,39.1839602767271,6.80100335360935));
#24075=CARTESIAN_POINT('Ctrl Pts',(-32.1874438377366,38.3319953452796,6.64400322625709));
#24076=CARTESIAN_POINT('Ctrl Pts',(-30.6693195563919,34.4921735803525,6.48700309890483));
#24077=CARTESIAN_POINT('Ctrl Pts',(-33.0345683933729,31.1077368710331,6.33000297155259));
#24078=CARTESIAN_POINT('Ctrl Pts',(-37.1622334356032,31.2135237769978,6.17300284420032));
#24079=CARTESIAN_POINT('Ctrl Pts',(-39.3510055801728,34.7146832529224,6.01600271684808));
#24080=CARTESIAN_POINT('Ctrl Pts',(-37.6381880046832,38.4716874963794,5.85900258949581));
#24081=CARTESIAN_POINT('Ctrl Pts',(-33.5596825685645,39.11559699904,5.70200246214357));
#24082=CARTESIAN_POINT('Ctrl Pts',(-30.7727232768428,36.0690108205182,5.54500233479131));
#24083=CARTESIAN_POINT('Ctrl Pts',(-31.7764037333916,32.0638325667482,5.38800220743906));
#24084=CARTESIAN_POINT('Ctrl Pts',(-35.6707138105653,30.6915437277723,5.23100208008681));
#24085=CARTESIAN_POINT('Ctrl Pts',(-38.9635884177054,33.1826890066978,5.07400195273455));
#24086=CARTESIAN_POINT('Ctrl Pts',(-38.7022752466618,37.3034344653991,4.9170018253823));
#24087=CARTESIAN_POINT('Ctrl Pts',(-35.1210963533887,39.3586681519579,4.76000169803004));
#24088=CARTESIAN_POINT('Ctrl Pts',(-31.4313291935845,37.5054422859516,4.6030015706778));
#24089=CARTESIAN_POINT('Ctrl Pts',(-30.9416233845026,33.4055622887757,4.44600144332554));
#24090=CARTESIAN_POINT('Ctrl Pts',(-34.091102819686,30.7354298821828,4.28900131597329));
#24091=CARTESIAN_POINT('Ctrl Pts',(-38.0555990765859,31.8893784134534,4.13200118862103));
#24092=CARTESIAN_POINT('Ctrl Pts',(-39.2801103271579,35.8326511627796,3.97500106126878));
#24093=CARTESIAN_POINT('Ctrl Pts',(-36.6666055859447,39.0292776269525,3.81800093391652));
#24094=CARTESIAN_POINT('Ctrl Pts',(-32.5586396271459,38.6128121869325,3.66100080656428));
#24095=CARTESIAN_POINT('Ctrl Pts',(-30.639864935887,34.9567034009586,3.50400067921202));
#24096=CARTESIAN_POINT('Ctrl Pts',(-32.6308651862137,31.3394190871117,3.34700055185977));
#24097=CARTESIAN_POINT('Ctrl Pts',(-36.7462913517739,31.0046128030999,3.19000042450751));
#24098=CARTESIAN_POINT('Ctrl Pts',(-39.2958013105393,34.2525085340193,3.03300029715526));
#24099=CARTESIAN_POINT('Ctrl Pts',(-37.9932250190614,38.1706870628692,2.876000169803));
#24100=CARTESIAN_POINT('Ctrl Pts',(-34.0065951433993,39.2456800252801,2.71900004245075));
#24101=CARTESIAN_POINT('Ctrl Pts',(-30.9107609206391,36.5135310965947,2.5619999150985));
#24102=CARTESIAN_POINT('Ctrl Pts',(-31.4817866355154,32.4241840741688,2.40499978774625));
#24103=CARTESIAN_POINT('Ctrl Pts',(-35.2076279765999,30.6445963856486,2.24799966039399));
#24104=CARTESIAN_POINT('Ctrl Pts',(-38.7472874197615,32.7705399311592,2.09099953304174));
#24105=CARTESIAN_POINT('Ctrl Pts',(-38.9267180811614,36.8956636643883,1.93399940568948));
#24106=CARTESIAN_POINT('Ctrl Pts',(-35.5850233760853,39.3209236645512,1.77699927833723));
#24107=CARTESIAN_POINT('Ctrl Pts',(-31.7187317751118,37.8715778961193,1.61999915098498));
#24108=CARTESIAN_POINT('Ctrl Pts',(-30.7947865264321,33.8472446970093,1.46299902363273));
#24109=CARTESIAN_POINT('Ctrl Pts',(-33.6416932068317,30.8566304310881,1.30599889628047));
#24110=CARTESIAN_POINT('Ctrl Pts',(-37.7066133387528,31.581350558394,1.14899876892822));
#24111=CARTESIAN_POINT('Ctrl Pts',(-39.3444737893792,35.371737063412,0.991998641575963));
#24112=CARTESIAN_POINT('Ctrl Pts',(-37.086630176448,38.8285202538281,0.834998514223711));
#24113=CARTESIAN_POINT('Ctrl Pts',(-32.9576303530114,38.8527626236071,0.677998386871457));
#24114=CARTESIAN_POINT('Ctrl Pts',(-30.6601535680437,35.421128079535,0.520998259519203));
#24115=CARTESIAN_POINT('Ctrl Pts',(-32.2540363563655,31.6140157217992,0.36399813216695));
#24116=CARTESIAN_POINT('Ctrl Pts',(-36.31069222556,30.8387971276259,0.206998004814696));
#24117=CARTESIAN_POINT('Ctrl Pts',(-39.1912024257666,33.8039222921716,0.0499978774624438));
#24118=CARTESIAN_POINT('Ctrl Pts',(-38.6056283266121,36.4808402609044,-0.0546688741057268));
#24119=CARTESIAN_POINT('Ctrl Pts',(-37.8143974874483,37.4062712808594,-0.107002249889811));
#24120=CARTESIAN_POINT('Ctrl Pts',(-35.9084720925035,31.6018409826581,8.32100674966943));
#24121=CARTESIAN_POINT('Ctrl Pts',(-37.0258557525633,31.9005650466595,8.26867337388535));
#24122=CARTESIAN_POINT('Ctrl Pts',(-38.9246979780591,33.681109870052,8.16400662231719));
#24123=CARTESIAN_POINT('Ctrl Pts',(-38.2651830194642,37.552344590298,8.00700649496492));
#24124=CARTESIAN_POINT('Ctrl Pts',(-34.6722755044984,39.1283078703588,7.85000636761267));
#24125=CARTESIAN_POINT('Ctrl Pts',(-31.3759281699498,37.005546565386,7.69300624026042));
#24126=CARTESIAN_POINT('Ctrl Pts',(-31.3279888911377,33.0828275365354,7.53600611290817));
#24127=CARTESIAN_POINT('Ctrl Pts',(-34.5734382940869,30.8800318042114,7.37900598555591));
#24128=CARTESIAN_POINT('Ctrl Pts',(-38.2010614834652,32.3712656979296,7.22200585820366));
#24129=CARTESIAN_POINT('Ctrl Pts',(-38.9584250576736,36.2199021770154,7.06500573085141));
#24130=CARTESIAN_POINT('Ctrl Pts',(-36.1661500230565,38.9745456920523,6.90800560349915));
#24131=CARTESIAN_POINT('Ctrl Pts',(-32.3282172298434,38.1652231067258,6.7510054761469));
#24132=CARTESIAN_POINT('Ctrl Pts',(-30.8860777439641,34.5175911875294,6.59400534879464));
#24133=CARTESIAN_POINT('Ctrl Pts',(-33.1329417086976,31.3025514994443,6.43700522144239));
#24134=CARTESIAN_POINT('Ctrl Pts',(-37.0540098419411,31.4030435843515,6.28000509409013));
#24135=CARTESIAN_POINT('Ctrl Pts',(-39.1332300836993,34.7289638588885,6.12300496673789));
#24136=CARTESIAN_POINT('Ctrl Pts',(-37.5061420461286,38.2979234195025,5.96600483938563));
#24137=CARTESIAN_POINT('Ctrl Pts',(-33.6317729940835,38.9096041168808,5.80900471203338));
#24138=CARTESIAN_POINT('Ctrl Pts',(-30.9843059259921,36.0155049451787,5.65200458468113));
#24139=CARTESIAN_POINT('Ctrl Pts',(-31.937750407041,32.2107929207913,5.49500445732887));
#24140=CARTESIAN_POINT('Ctrl Pts',(-35.6371434024388,30.9071895564043,5.33800432997662));
#24141=CARTESIAN_POINT('Ctrl Pts',(-38.765203832906,33.2736486243128,5.18100420262436));
#24142=CARTESIAN_POINT('Ctrl Pts',(-38.5169698465499,37.1881435113763,5.02400407527211));
#24143=CARTESIAN_POINT('Ctrl Pts',(-35.1150352675099,39.1405091302639,4.86700394791986));
#24144=CARTESIAN_POINT('Ctrl Pts',(-31.6099474560293,37.3800404845393,4.7100038205676));
#24145=CARTESIAN_POINT('Ctrl Pts',(-31.1447522856339,33.4853667058834,4.55300369321536));
#24146=CARTESIAN_POINT('Ctrl Pts',(-34.1365947251866,30.9488791314519,4.39600356586309));
#24147=CARTESIAN_POINT('Ctrl Pts',(-37.9026609583357,32.0450705052858,4.23900343851085));
#24148=CARTESIAN_POINT('Ctrl Pts',(-39.0658832630269,35.7909755048144,4.08200331115859));
#24149=CARTESIAN_POINT('Ctrl Pts',(-36.5831890395356,38.8276051814752,3.92500318380634));
#24150=CARTESIAN_POINT('Ctrl Pts',(-32.6808340158849,38.4319845706085,3.76800305645408));
#24151=CARTESIAN_POINT('Ctrl Pts',(-30.8580973791193,34.9588704720363,3.61100292910183));
#24152=CARTESIAN_POINT('Ctrl Pts',(-32.7494445584481,31.522637612346,3.45400280174958));
#24153=CARTESIAN_POINT('Ctrl Pts',(-36.6588863923657,31.2045889728327,3.29700267439732));
#24154=CARTESIAN_POINT('Ctrl Pts',(-39.0807888850399,34.2899217990943,3.14000254704507));
#24155=CARTESIAN_POINT('Ctrl Pts',(-37.8434088323037,38.0119885881016,2.98300241969281));
#24156=CARTESIAN_POINT('Ctrl Pts',(-34.0563168070145,39.0331762584299,2.82600229234057));
#24157=CARTESIAN_POINT('Ctrl Pts',(-31.1154345424715,36.4377761981199,2.66900216498831));
#24158=CARTESIAN_POINT('Ctrl Pts',(-31.6578794140771,32.553108200267,2.51200203763606));
#24159=CARTESIAN_POINT('Ctrl Pts',(-35.1972358304966,30.8625920114828,2.3550019102838));
#24160=CARTESIAN_POINT('Ctrl Pts',(-38.559729081067,32.8821283362792,2.19800178293155));
#24161=CARTESIAN_POINT('Ctrl Pts',(-38.7301789216776,36.8007823575152,2.04100165557929));
#24162=CARTESIAN_POINT('Ctrl Pts',(-35.555741925205,39.1046538209638,1.88400152822704));
#24163=CARTESIAN_POINT('Ctrl Pts',(-31.8829650319005,37.727850362227,1.72700140087479));
#24164=CARTESIAN_POINT('Ctrl Pts',(-31.0052648710604,33.904942131268,1.57000127352254));
#24165=CARTESIAN_POINT('Ctrl Pts',(-33.7096788553892,31.0640133793093,1.41300114617028));
#24166=CARTESIAN_POINT('Ctrl Pts',(-37.5711425716514,31.7524599871677,1.25600101881803));
#24167=CARTESIAN_POINT('Ctrl Pts',(-39.127025220545,35.3531309683265,1.09900089146578));
#24168=CARTESIAN_POINT('Ctrl Pts',(-36.982190659132,38.6368960686431,0.942000764113521));
#24169=CARTESIAN_POINT('Ctrl Pts',(-33.0598545528336,38.6599250650956,0.785000636761268));
#24170=CARTESIAN_POINT('Ctrl Pts',(-30.8773705294847,35.4000498770575,0.628000509409013));
#24171=CARTESIAN_POINT('Ctrl Pts',(-32.391476675568,31.7834902015831,0.471000382056762));
#24172=CARTESIAN_POINT('Ctrl Pts',(-36.2450897700159,31.0470726641105,0.314000254704506));
#24173=CARTESIAN_POINT('Ctrl Pts',(-38.9814253587705,33.8637880891336,0.157000127352255));
#24174=CARTESIAN_POINT('Ctrl Pts',(-38.4251602751564,36.4067215963626,0.0523333757840841));
#24175=CARTESIAN_POINT('Ctrl Pts',(-37.6735319337713,37.2858331630075,0.));
#24176=CARTESIAN_POINT('Ctrl Pts',(-37.6735319337713,37.2858331630075,0.));
#24177=CARTESIAN_POINT('Ctrl Pts',(-37.7506745369995,37.2087203555594,1.28363488612132E-16));
#24178=CARTESIAN_POINT('Ctrl Pts',(-37.8237047828546,37.1279853831031,-1.45961390077584E-15));
#24179=CARTESIAN_POINT('Ctrl Pts',(-37.8926303634218,37.044046747423,-1.27675647831893E-15));
#24180=CARTESIAN_POINT('Ctrl Pts',(-37.9633158416367,36.9579648812288,-1.08923010211539E-15));
#24181=CARTESIAN_POINT('Ctrl Pts',(-38.0296847428869,36.8685132102372,2.69373606469353E-15));
#24182=CARTESIAN_POINT('Ctrl Pts',(-38.0917154903142,36.776096981172,2.1094237467878E-15));
#24183=CARTESIAN_POINT('Ctrl Pts',(-38.1550372699928,36.6817573135345,1.51295026561079E-15));
#24184=CARTESIAN_POINT('Ctrl Pts',(-38.2138388545422,36.5843278170101,-6.22870230136456E-16));
#24185=CARTESIAN_POINT('Ctrl Pts',(-38.2680604999532,36.4842001218513,-1.22124532708767E-15));
#24186=CARTESIAN_POINT('Ctrl Pts',(-38.3198497467852,36.3885641838418,-1.7927771454093E-15));
#24187=CARTESIAN_POINT('Ctrl Pts',(-38.3674607433557,36.2904658682844,-1.21061342909026E-15));
#24188=CARTESIAN_POINT('Ctrl Pts',(-38.4108059167409,36.1902218218841,-1.49880108324396E-15));
#24189=CARTESIAN_POINT('Ctrl Pts',(-38.4178437109143,36.1739455698685,-1.54559303803029E-15));
#24190=CARTESIAN_POINT('Ctrl Pts',(-38.4247689668943,36.1576127105175,5.76904931418396E-16));
#24191=CARTESIAN_POINT('Ctrl Pts',(-38.4315812162273,36.1412245565248,6.10622663543836E-16));
#24192=CARTESIAN_POINT('Ctrl Pts',(-38.4380909127403,36.1255642505548,6.42842888099819E-16));
#24193=CARTESIAN_POINT('Ctrl Pts',(-38.4444943995979,36.1098606451587,1.94214412995646E-15));
#24194=CARTESIAN_POINT('Ctrl Pts',(-38.4507894645608,36.0941203888398,1.88737914186277E-15));
#24195=CARTESIAN_POINT('Ctrl Pts',(-38.4941748650482,35.9856390104596,1.50994047282167E-15));
#24196=CARTESIAN_POINT('Ctrl Pts',(-38.5324464076346,35.8753406458803,4.14672721999528E-16));
#24197=CARTESIAN_POINT('Ctrl Pts',(-38.5655754746426,35.7636570985597,-1.11022302462516E-16));
#24198=CARTESIAN_POINT('Ctrl Pts',(-38.599139072954,35.6505086745683,-6.43612508853869E-16));
#24199=CARTESIAN_POINT('Ctrl Pts',(-38.6274248054533,35.535937741082,5.81275891054099E-16));
#24200=CARTESIAN_POINT('Ctrl Pts',(-38.6503602739825,35.4203607919199,1.85962356624714E-15));
#24201=CARTESIAN_POINT('Ctrl Pts',(-38.6743352598313,35.2995454827809,3.19591052212541E-15));
#24202=CARTESIAN_POINT('Ctrl Pts',(-38.692464786516,35.1776300814803,-8.4407659709162E-16));
#24203=CARTESIAN_POINT('Ctrl Pts',(-38.7046104310317,35.0550669428354,-1.38777878078145E-15));
#24204=CARTESIAN_POINT('Ctrl Pts',(-38.7137196644185,34.9631445888517,-1.79555541854881E-15));
#24205=CARTESIAN_POINT('Ctrl Pts',(-38.7194618408911,34.8708572859148,2.82896256593911E-15));
#24206=CARTESIAN_POINT('Ctrl Pts',(-38.721755434165,34.7783924177428,2.94209101525666E-15));
#24207=CARTESIAN_POINT('Ctrl Pts',(-38.7223030074901,34.7563173201712,2.96909934400004E-15));
#24208=CARTESIAN_POINT('Ctrl Pts',(-38.7226538674535,34.7342275752707,-2.60000342473094E-16));
#24209=CARTESIAN_POINT('Ctrl Pts',(-38.7228068022813,34.7121547959299,-2.77555756156289E-16));
#24210=CARTESIAN_POINT('Ctrl Pts',(-38.7236416666969,34.5916604762348,-3.73389977849103E-16));
#24211=CARTESIAN_POINT('Ctrl Pts',(-38.7185883671926,34.4715209673338,1.72146304164403E-15));
#24212=CARTESIAN_POINT('Ctrl Pts',(-38.7075779418993,34.3521623032552,1.58206781009085E-15));
#24213=CARTESIAN_POINT('Ctrl Pts',(-38.6966381726954,34.2335695874665,1.44356710546673E-15));
#24214=CARTESIAN_POINT('Ctrl Pts',(-38.6798177366068,34.1157468505408,1.14312909921041E-17));
#24215=CARTESIAN_POINT('Ctrl Pts',(-38.6569995558515,33.9990991317786,-2.77555756156289E-16));
#24216=CARTESIAN_POINT('Ctrl Pts',(-38.654125907022,33.9844088905153,-3.13949862184534E-16));
#24217=CARTESIAN_POINT('Ctrl Pts',(-38.6511570658937,33.9697372784049,2.13659354022824E-15));
#24218=CARTESIAN_POINT('Ctrl Pts',(-38.6480927394297,33.9550851007466,2.1094237467878E-15));
#24219=CARTESIAN_POINT('Ctrl Pts',(-38.6241822697972,33.8407564046822,1.89676768741005E-15));
#24220=CARTESIAN_POINT('Ctrl Pts',(-38.5944625878303,33.7276104213963,7.3858195394121E-16));
#24221=CARTESIAN_POINT('Ctrl Pts',(-38.5592398399973,33.6159136444833,2.4980018054066E-16));
#24222=CARTESIAN_POINT('Ctrl Pts',(-38.5372745858279,33.5462584288701,-5.50089711192647E-17));
#24223=CARTESIAN_POINT('Ctrl Pts',(-38.5131681698132,33.4771668829623,6.13912691963219E-16));
#24224=CARTESIAN_POINT('Ctrl Pts',(-38.4869849848521,33.408705821156,6.93889390390723E-16));
#24225=CARTESIAN_POINT('Ctrl Pts',(-38.478035242453,33.3853049679579,7.21226433226402E-16));
#24226=CARTESIAN_POINT('Ctrl Pts',(-38.4688427975352,33.3619777978058,1.17968218996551E-15));
#24227=CARTESIAN_POINT('Ctrl Pts',(-38.4594100345669,33.3387270476804,1.30451205393456E-15));
#24228=CARTESIAN_POINT('Ctrl Pts',(-38.4526611227965,33.3220917032197,1.39382477610025E-15));
#24229=CARTESIAN_POINT('Ctrl Pts',(-38.4457886431155,33.3054943585584,8.23245697379087E-16));
#24230=CARTESIAN_POINT('Ctrl Pts',(-38.4388005380928,33.2889523169239,7.49400541621981E-16));
#24231=CARTESIAN_POINT('Ctrl Pts',(-38.3928792100309,33.1802486671866,2.64137711097381E-16));
#24232=CARTESIAN_POINT('Ctrl Pts',(-38.3419048511529,33.0737714082961,1.17255001397609E-15));
#24233=CARTESIAN_POINT('Ctrl Pts',(-38.2862359020984,32.9697748885158,9.43689570931383E-16));
#24234=CARTESIAN_POINT('Ctrl Pts',(-38.2286517312081,32.8622004961707,7.06955465363536E-16));
#24235=CARTESIAN_POINT('Ctrl Pts',(-38.1660442194156,32.7572797837933,2.65690729149937E-16));
#24236=CARTESIAN_POINT('Ctrl Pts',(-38.0987547078419,32.6553015987604,4.44089209850063E-16));
#24237=CARTESIAN_POINT('Ctrl Pts',(-38.0308320192805,32.5523638252493,6.24166374344619E-16));
#24238=CARTESIAN_POINT('Ctrl Pts',(-37.9581383688774,32.4524234721426,-1.26765506881022E-15));
#24239=CARTESIAN_POINT('Ctrl Pts',(-37.8809743110047,32.3557958917759,-1.62370117351429E-15));
#24240=CARTESIAN_POINT('Ctrl Pts',(-37.82656120339,32.2876578612733,-1.87477110872936E-15));
#24241=CARTESIAN_POINT('Ctrl Pts',(-37.7699241047827,32.2211674765398,1.39931090156461E-15));
#24242=CARTESIAN_POINT('Ctrl Pts',(-37.7111553490298,32.1564437978227,1.60982338570648E-15));
#24243=CARTESIAN_POINT('Ctrl Pts',(-37.6849229569216,32.1275533287794,1.70378906452554E-15));
#24244=CARTESIAN_POINT('Ctrl Pts',(-37.6582657142846,32.0990149717255,2.33543966985802E-16));
#24245=CARTESIAN_POINT('Ctrl Pts',(-37.6311912225754,32.0708398884709,3.05311331771918E-16));
#24246=CARTESIAN_POINT('Ctrl Pts',(-37.6195692277271,32.0587454537553,3.36118186902312E-16));
#24247=CARTESIAN_POINT('Ctrl Pts',(-37.6078717672662,32.0467194961249,-1.14899013469077E-15));
#24248=CARTESIAN_POINT('Ctrl Pts',(-37.5961059477358,32.034769281675,-1.17961196366423E-15));
#24249=CARTESIAN_POINT('Ctrl Pts',(-37.5076636824121,31.9449409416833,-1.40979260818075E-15));
#24250=CARTESIAN_POINT('Ctrl Pts',(-37.4152620841693,31.8592852286376,-2.45663089159861E-15));
#24251=CARTESIAN_POINT('Ctrl Pts',(-37.3192298936088,31.778120294682,-2.019218126037E-15));
#24252=CARTESIAN_POINT('Ctrl Pts',(-37.2371898445147,31.7087813040001,-1.64553754506066E-15));
#24253=CARTESIAN_POINT('Ctrl Pts',(-37.1524990927587,31.6427198578901,-2.42654488972963E-15));
#24254=CARTESIAN_POINT('Ctrl Pts',(-37.0653383821438,31.5801518871639,-2.52575738102223E-15));
#24255=CARTESIAN_POINT('Ctrl Pts',(-37.0262273476737,31.5520761860535,-2.57027632928952E-15));
#24256=CARTESIAN_POINT('Ctrl Pts',(-36.9866187071144,31.524704156366,-1.17712968719052E-15));
#24257=CARTESIAN_POINT('Ctrl Pts',(-36.946527548351,31.4980566647868,-6.31439345255558E-16));
#24258=CARTESIAN_POINT('Ctrl Pts',(-36.9192934800282,31.479954927928,-2.60749933581654E-16));
#24259=CARTESIAN_POINT('Ctrl Pts',(-36.89183110785,31.4621841581827,-1.11508673223599E-15));
#24260=CARTESIAN_POINT('Ctrl Pts',(-36.8641751230777,31.4447696709256,-1.17267306976032E-15));
#24261=CARTESIAN_POINT('Ctrl Pts',(-36.757370770553,31.3775168483861,-1.39506513224507E-15));
#24262=CARTESIAN_POINT('Ctrl Pts',(-36.6476196941272,31.3155308365787,-2.17833836995006E-15));
#24263=CARTESIAN_POINT('Ctrl Pts',(-36.5352238715355,31.2591452947779,-6.38378239159465E-16));
#24264=CARTESIAN_POINT('Ctrl Pts',(-36.4331301648989,31.2079280090246,7.60430312613923E-16));
#24265=CARTESIAN_POINT('Ctrl Pts',(-36.3288535333025,31.1613315369686,5.40797342115576E-17));
#24266=CARTESIAN_POINT('Ctrl Pts',(-36.2225969429285,31.1196350477066,-1.58727198051878E-16));
#24267=CARTESIAN_POINT('Ctrl Pts',(-36.1671664218874,31.0978833792477,-2.38185072021888E-16));
#24268=CARTESIAN_POINT('Ctrl Pts',(-36.1111967480356,31.0774656809663,2.2162435752245E-16));
#24269=CARTESIAN_POINT('Ctrl Pts',(-36.0547320440516,31.0583698407596,1.38777878078145E-16));
#24270=CARTESIAN_POINT('Ctrl Pts',(-38.5153120432796,35.002811202661,7.11258330249199));
#24271=CARTESIAN_POINT('Ctrl Pts',(-38.5180431912138,35.3538028140734,7.09672411194513));
#24272=CARTESIAN_POINT('Ctrl Pts',(-38.4695957643305,35.7040585809451,7.08086492139827));
#24273=CARTESIAN_POINT('Ctrl Pts',(-38.3668186228693,36.0375700163406,7.06500573085141));
#24274=CARTESIAN_POINT('Ctrl Pts',(-38.0276667128012,37.1381166820277,7.01267235506732));
#24275=CARTESIAN_POINT('Ctrl Pts',(-37.0969083679288,38.05633118704,6.96033897928324));
#24276=CARTESIAN_POINT('Ctrl Pts',(-35.9918737299572,38.3805513419917,6.90800560349915));
#24277=CARTESIAN_POINT('Ctrl Pts',(-34.8868390919855,38.7047714969434,6.85567222771507));
#24278=CARTESIAN_POINT('Ctrl Pts',(-33.6075281609145,38.4349973018346,6.80333885193099));
#24279=CARTESIAN_POINT('Ctrl Pts',(-32.7275161143991,37.6921715510808,6.7510054761469));
#24280=CARTESIAN_POINT('Ctrl Pts',(-31.8475040678837,36.949345800327,6.69867210036282));
#24281=CARTESIAN_POINT('Ctrl Pts',(-31.3667909059239,35.7334684939282,6.64633872457873));
#24282=CARTESIAN_POINT('Ctrl Pts',(-31.5009116523996,34.5896898927146,6.59400534879465));
#24283=CARTESIAN_POINT('Ctrl Pts',(-31.6350323988753,33.445911291501,6.54167197301056));
#24284=CARTESIAN_POINT('Ctrl Pts',(-32.3839870537864,32.3742313954726,6.48933859722648));
#24285=CARTESIAN_POINT('Ctrl Pts',(-33.4119757367826,31.8551401282763,6.43700522144239));
#24286=CARTESIAN_POINT('Ctrl Pts',(-34.4399644197788,31.33604886108,6.38467184565831));
#24287=CARTESIAN_POINT('Ctrl Pts',(-35.74698713086,31.3695462227158,6.33233846987422));
#24288=CARTESIAN_POINT('Ctrl Pts',(-36.7470351933603,31.9406149492898,6.28000509409014));
#24289=CARTESIAN_POINT('Ctrl Pts',(-37.7470832558605,32.5116836758639,6.22767171830605));
#24290=CARTESIAN_POINT('Ctrl Pts',(-38.4401566697799,33.6203237673762,6.17533834252197));
#24291=CARTESIAN_POINT('Ctrl Pts',(-38.5155120371445,34.769470406568,6.12300496673789));
#24292=CARTESIAN_POINT('Ctrl Pts',(-38.5205141244106,34.8457507296795,6.11953107865592));
#24293=CARTESIAN_POINT('Ctrl Pts',(-38.5227943601281,34.922209536826,6.11605719057395));
#24294=CARTESIAN_POINT('Ctrl Pts',(-38.5224238694764,34.9986908177615,6.11258330249199));
#24295=CARTESIAN_POINT('Origin',(35.,-35.,4.));
#24296=CARTESIAN_POINT('Origin',(-35.,-35.,4.));
#24297=CARTESIAN_POINT('Origin',(-35.,35.,4.));
#24298=CARTESIAN_POINT('Origin',(35.,35.,4.));
#24299=CARTESIAN_POINT('Origin',(50.,50.,0.));
#24300=CARTESIAN_POINT('',(50.,50.,0.));
#24301=CARTESIAN_POINT('',(-50.,50.,0.));
#24302=CARTESIAN_POINT('',(50.,50.,0.));
#24303=CARTESIAN_POINT('',(-50.,50.,0.));
#24304=CARTESIAN_POINT('',(50.,50.,0.));
#24305=CARTESIAN_POINT('Origin',(50.,-50.,0.));
#24306=CARTESIAN_POINT('',(50.,-50.,0.));
#24307=CARTESIAN_POINT('',(50.,-50.,0.));
#24308=CARTESIAN_POINT('',(50.,-50.,0.));
#24309=CARTESIAN_POINT('Origin',(-50.,-50.,0.));
#24310=CARTESIAN_POINT('',(-50.,-50.,0.));
#24311=CARTESIAN_POINT('',(-50.,-50.,0.));
#24312=CARTESIAN_POINT('',(-50.,-50.,0.));
#24313=CARTESIAN_POINT('Origin',(-50.,50.,0.));
#24314=CARTESIAN_POINT('',(-50.,50.,0.));
#24315=CARTESIAN_POINT('Origin',(0.,0.,0.));
#63720=UNCERTAINTY_MEASURE_WITH_UNIT(LENGTH_MEASURE(0.01),#63756,
'DISTANCE_ACCURACY_VALUE',
'Maximum model space distance between geometric entities at asserted c
onnectivities');
#63735=UNCERTAINTY_MEASURE_WITH_UNIT(LENGTH_MEASURE(0.01),#63756,
'DISTANCE_ACCURACY_VALUE',
'Maximum model space distance between geometric entities at asserted c
onnectivities');
#63740=(
GEOMETRIC_REPRESENTATION_CONTEXT(3)
GLOBAL_UNCERTAINTY_ASSIGNED_CONTEXT((#63720))
GLOBAL_UNIT_ASSIGNED_CONTEXT((#63756,#63758,#63759))
REPRESENTATION_CONTEXT('','3D')
);
#63755=(
GEOMETRIC_REPRESENTATION_CONTEXT(3)
GLOBAL_UNCERTAINTY_ASSIGNED_CONTEXT((#63735))
GLOBAL_UNIT_ASSIGNED_CONTEXT((#63756,#63758,#63759))
REPRESENTATION_CONTEXT('','3D')
);
#63756=(
LENGTH_UNIT()
NAMED_UNIT(*)
SI_UNIT(.MILLI.,.METRE.)
);
#63758=(
NAMED_UNIT(*)
PLANE_ANGLE_UNIT()
SI_UNIT($,.RADIAN.)
);
#63759=(
NAMED_UNIT(*)
SI_UNIT($,.STERADIAN.)
SOLID_ANGLE_UNIT()
);
#63764=SHAPE_DEFINITION_REPRESENTATION(#63783,#63862);
#63783=PRODUCT_DEFINITION_SHAPE('',$,#63882);
#63862=SHAPE_REPRESENTATION('',(#14526),#63740);
#63877=PRODUCT_DEFINITION_CONTEXT('part definition',#63936,'design');
#63882=PRODUCT_DEFINITION('Corner plate','Corner plate',#63901,#63877);
#63901=PRODUCT_DEFINITION_FORMATION('',$,#63942);
#63936=APPLICATION_CONTEXT(
'Core Data for Automotive Mechanical Design Process');
#63937=PRODUCT_CONTEXT('part definition',#63936,'mechanical');
#63942=PRODUCT('Corner plate','Corner plate',
'Weld rails to upper face. Four M8x1 attachment taps on 70 mm square p
attern match the leg plate clearance holes.',(#63937));
#63959=PRESENTATION_STYLE_ASSIGNMENT((#63966));
#63966=SURFACE_STYLE_USAGE(.BOTH.,#63973);
#63973=SURFACE_SIDE_STYLE('',(#63980));
#63980=SURFACE_STYLE_FILL_AREA(#63987);
#63987=FILL_AREA_STYLE('Sky blue',(#63994));
#63994=FILL_AREA_STYLE_COLOUR('Sky blue',#64001);
#64001=COLOUR_RGB('Sky blue',0.317647058823529,0.686274509803922,0.890196078431372);
ENDSEC;
END-ISO-10303-21;
